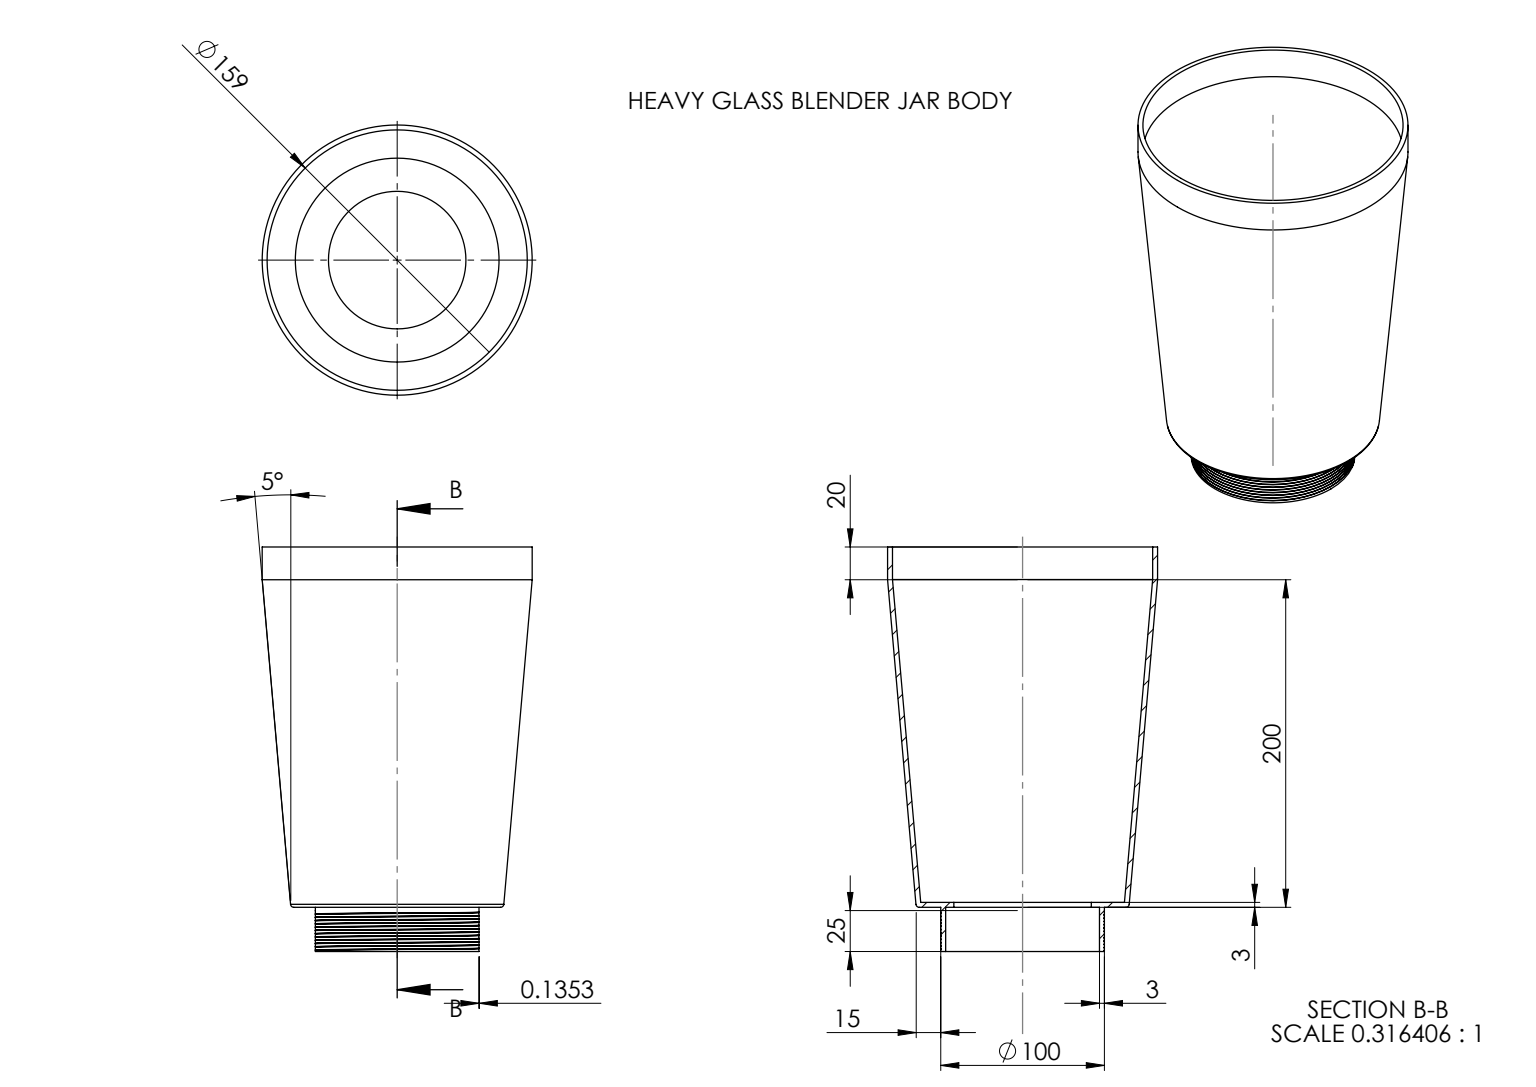
ISO-10303-21;
HEADER;
FILE_DESCRIPTION (('STEP AP214'),
    '1' );
FILE_NAME ('Heavy Glass Blender Jar Body.step',
    '2026-10-09T15:02:13',
    ( '' ),
    ( '' ),
    'SwSTEP 2.0',
    'SolidWorks 2026',
    '' );
FILE_SCHEMA (( 'AUTOMOTIVE_DESIGN' ));
ENDSEC;

DATA;
#4=CARTESIAN_POINT ( 'NONE',  ( -40.34137639590981905, 29.65937500034139518, -29.30972558990011478 ) ) ;
#8=CARTESIAN_POINT ( 'NONE',  ( 47.50025713571348263, 25.00000000000000000, -15.17274647889483496 ) ) ;
#9=CARTESIAN_POINT ( 'NONE',  ( 49.86468353124999453, 35.02187500034139589, -16.20201782572376104 ) ) ;
#10=EDGE_CURVE ( 'NONE', #4476, #13481, #11027, .T. ) ;
#13=LINE ( 'NONE', #15220, #1773 ) ;
#15=DIRECTION ( 'NONE',  ( 0.000000000000000000, 0.9961946980917455452, 0.08715574274765836016 ) ) ;
#18=CARTESIAN_POINT ( 'NONE',  ( 15.40903463028481113, 31.32187500034139305, -47.42413220539094709 ) ) ;
#22=CARTESIAN_POINT ( 'NONE',  ( -30.81806926056962226, 34.15937500034139163, 42.41743335407647209 ) ) ;
#23=ORIENTED_EDGE ( 'NONE', *, *, #4819, .F. ) ;
#26=CARTESIAN_POINT ( 'NONE',  ( -40.45084971874737079, 19.98125000068279888, 29.38926261462367151 ) ) ;
#28=CARTESIAN_POINT ( 'NONE',  ( 15.40903463028481113, 21.32187500034139660, -47.42413220539094709 ) ) ;
#33=CARTESIAN_POINT ( 'NONE',  ( -40.45084971874737789, 45.79999999999999716, -29.38926261462365730 ) ) ;
#41=EDGE_CURVE ( 'NONE', #13641, #5789, #12730, .T. ) ;
#47=( NAMED_UNIT ( * ) SI_UNIT ( $, .STERADIAN. ) SOLID_ANGLE_UNIT ( ) );
#54=CARTESIAN_POINT ( 'NONE',  ( -15.40903463028481646, 25.45937500034139589, -47.42413220539093999 ) ) ;
#56=CARTESIAN_POINT ( 'NONE',  ( -40.45084971874737789, 25.80000000000000071, -29.38926261462365730 ) ) ;
#59=FACE_OUTER_BOUND ( 'NONE', #13989, .T. ) ;
#61=CARTESIAN_POINT ( 'NONE',  ( -1.240322475938754499E-13, 36.28125000068280315, 50.00000000000000000 ) ) ;
#72=CARTESIAN_POINT ( 'NONE',  ( -49.99999999999999289, 23.90000000000000213, -16.24598481164531449 ) ) ;
#76=CARTESIAN_POINT ( 'NONE',  ( 49.86468353124999453, 44.95937500034139589, -16.20201782572376459 ) ) ;
#79=DIRECTION ( 'NONE',  ( -0.000000000000000000, -1.000000000000000000, -0.000000000000000000 ) ) ;
#80=CARTESIAN_POINT ( 'NONE',  ( -49.86468353124999453, 25.95937500034139944, 16.20201782572377525 ) ) ;
#85=CARTESIAN_POINT ( 'NONE',  ( 47.13255506291616115, 25.00000000000000711, -16.27994764699579022 ) ) ;
#86=CARTESIAN_POINT ( 'NONE',  ( -15.40903463028480580, 34.32187500034139305, 47.42413220539094709 ) ) ;
#87=( BOUNDED_CURVE ( )  B_SPLINE_CURVE ( 2, ( #12702, #8875, #13934, #16199, #7548, #15262, #4829, #3730, #6314, #2555, #11379, #10211, #16445 ),
 .UNSPECIFIED., .F., .F. ) 
 B_SPLINE_CURVE_WITH_KNOTS ( ( 3, 2, 2, 2, 2, 2, 3 ),
 ( 0.3166666666666667074, 0.3200000000000000067, 0.3266666666666666607, 0.3333333333333333148, 0.3400000000000000244, 0.3466666666666666785, 0.3500000000000000333 ),
 .UNSPECIFIED. ) 
 CURVE ( )  GEOMETRIC_REPRESENTATION_ITEM ( )  RATIONAL_B_SPLINE_CURVE ( ( 0.9755282581475768211, 0.9755282581475770431, 1.000000000000000000, 0.9510565162951535312, 1.000000000000000000, 0.9510565162951535312, 1.000000000000000000, 0.9510565162951535312, 1.000000000000000000, 0.9510565162951535312, 1.000000000000000000, 0.9755282581475765991, 0.9755282581475768211 ) ) 
 REPRESENTATION_ITEM ( '' )  );
#96=CARTESIAN_POINT ( 'NONE',  ( 30.81806926056964002, 30.62187500034139020, 42.41743335407647209 ) ) ;
#101=CARTESIAN_POINT ( 'NONE',  ( -40.34137639590981905, 35.65937500034139873, -29.30972558990011478 ) ) ;
#104=CARTESIAN_POINT ( 'NONE',  ( -30.81806926056963292, 47.55937500034139731, -42.41743335407647209 ) ) ;
#106=CARTESIAN_POINT ( 'NONE',  ( -49.86468353124999453, 23.82187500034139305, -16.20201782572375393 ) ) ;
#111=CARTESIAN_POINT ( 'NONE',  ( 40.45084971874737789, 44.79999999999999716, 29.38926261462365375 ) ) ;
#120=CARTESIAN_POINT ( 'NONE',  ( -30.90169943749473447, 32.30000000000000426, 42.53254041760200721 ) ) ;
#123=CARTESIAN_POINT ( 'NONE',  ( -49.86468353124999453, 48.02187500034139589, 16.20201782572377169 ) ) ;
#125=EDGE_CURVE ( 'NONE', #10026, #5291, #8135, .T. ) ;
#130=DIRECTION ( 'NONE',  ( 0.000000000000000000, 0.000000000000000000, -1.000000000000000000 ) ) ;
#135=CARTESIAN_POINT ( 'NONE',  ( -15.40903463028481646, 47.52187500034139589, -47.42413220539093999 ) ) ;
#136=ORIENTED_EDGE ( 'NONE', *, *, #8247, .T. ) ;
#138=ORIENTED_EDGE ( 'NONE', *, *, #3634, .T. ) ;
#145=DIRECTION ( 'NONE',  ( 0.000000000000000000, 1.000000000000000000, 0.000000000000000000 ) ) ;
#160=CARTESIAN_POINT ( 'NONE',  ( 15.45084971874737789, 20.60000000000000142, 47.55282581475767500 ) ) ;
#163=CARTESIAN_POINT ( 'NONE',  ( -49.86468353124999453, 37.95937500034140299, 16.20201782572377525 ) ) ;
#171=CARTESIAN_POINT ( 'NONE',  ( -40.34137639590981905, 31.65937500034139873, -29.30972558990011478 ) ) ;
#175=CARTESIAN_POINT ( 'NONE',  ( 46.62157290631164130, 24.99999999999999289, -17.69020581816995730 ) ) ;
#176=CARTESIAN_POINT ( 'NONE',  ( -40.34137639590981195, 32.12187500034140442, 29.30972558990012189 ) ) ;
#177=CARTESIAN_POINT ( 'NONE',  ( 30.90169943749475223, 46.48125000068280599, 42.53254041760199300 ) ) ;
#185=CARTESIAN_POINT ( 'NONE',  ( 9.631387414534489405E-15, 32.42187500034139447, 52.43083105670540789 ) ) ;
#186=ORIENTED_EDGE ( 'NONE', *, *, #13105, .F. ) ;
#187=CARTESIAN_POINT ( 'NONE',  ( 40.34137639590981195, 33.05937500034139731, -29.30972558990011834 ) ) ;
#188=ORIENTED_EDGE ( 'NONE', *, *, #204, .F. ) ;
#191=CARTESIAN_POINT ( 'NONE',  ( -30.90169943749473802, 20.08125000068279320, 42.53254041760200721 ) ) ;
#194=CARTESIAN_POINT ( 'NONE',  ( 30.81806926056964002, 26.62187500034139731, 42.41743335407647209 ) ) ;
#200=CARTESIAN_POINT ( 'NONE',  ( 30.90169943749474157, 49.29999999999999716, -42.53254041760200721 ) ) ;
#204=EDGE_CURVE ( 'NONE', #5010, #3842, #426, .T. ) ;
#206=EDGE_LOOP ( 'NONE', ( #10234, #136 ) ) ;
#207=CARTESIAN_POINT ( 'NONE',  ( 50.00000000000000000, 36.78125000068280315, -6.123233995736766085E-15 ) ) ;
#208=AXIS2_PLACEMENT_3D ( 'NONE', #5247, #15355, #10131 ) ;
#209=ORIENTED_EDGE ( 'NONE', *, *, #12461, .T. ) ;
#215=CARTESIAN_POINT ( 'NONE',  ( 49.86468353124999453, 45.02187500034138878, -16.20201782572376104 ) ) ;
#221=CARTESIAN_POINT ( 'NONE',  ( 50.00000000000000000, 34.78125000068280315, -6.123233995736766085E-15 ) ) ;
#225=CARTESIAN_POINT ( 'NONE',  ( -49.86468353125000164, 45.92187500034139447, 0.000000000000000000 ) ) ;
#241=CARTESIAN_POINT ( 'NONE',  ( -50.00000000000000000, 20.00000000000000000, 0.000000000000000000 ) ) ;
#244=CARTESIAN_POINT ( 'NONE',  ( -3.210462471511496205E-15, 39.35937500034138736, -52.43083105670540789 ) ) ;
#247=CARTESIAN_POINT ( 'NONE',  ( 49.99999999999999289, 48.88125000068279746, -16.24598481164532160 ) ) ;
#249=CARTESIAN_POINT ( 'NONE',  ( -49.86468353124999453, 31.75937500034140015, -16.20201782572375393 ) ) ;
#252=CARTESIAN_POINT ( 'NONE',  ( 50.00000000000000711, 26.89999999999999858, 16.24598481164530739 ) ) ;
#255=CARTESIAN_POINT ( 'NONE',  ( 30.81806926056962936, 35.22187500034138452, -42.41743335407646498 ) ) ;
#263=CARTESIAN_POINT ( 'NONE',  ( -15.40903463028481646, 27.52187500034139944, -47.42413220539093999 ) ) ;
#266=B_SPLINE_CURVE_WITH_KNOTS ( 'NONE', 3,
 ( #13888, #7584, #1338, #3766, #3845, #12662, #9000, #3929, #8825, #2503, #1169, #9081, #15216, #1258, #12497, #11416, #1090, #15389, #12572, #6350, #6265, #8, #6428, #1418, #6182, #14058, #2674, #11488, #85, #7748, #12816, #6510, #3692, #15064, #11567, #5111, #10245, #175, #10166, #5280, #11336, #10331, #4011, #2348, #16313, #7429, #11256, #8911, #4949, #10007, #8747, #13812, #2423, #7501, #16403, #10088, #13975, #5036, #2594, #15138, #7670 ),
 .UNSPECIFIED., .F., .F.,
 ( 4, 3, 3, 3, 3, 3, 3, 3, 3, 3, 3, 3, 3, 3, 3, 3, 3, 3, 3, 3, 4 ),
 ( 5.250942343321584884E-16, 0.0001250000981872776470, 0.0006250122739946113812, 0.001125024449802053753, 0.001625036625609322868, 0.002125048801416675251, 0.002625060977223842018, 0.003125073153031292413, 0.003625085328838458312, 0.004125097504645739571, 0.004625109680452853429, 0.005125121856260251782, 0.005625134032067363038, 0.006125146207874809963, 0.006625158383682325410, 0.007125170559489371613, 0.007625182735296599096, 0.008125194911103644432, 0.008625207086911109572, 0.009137502482430032158, 0.009649851960371033655 ),
 .UNSPECIFIED. ) ;
#267=CARTESIAN_POINT ( 'NONE',  ( 15.40903463028481113, 39.25937500034140015, -47.42413220539094709 ) ) ;
#268=ORIENTED_EDGE ( 'NONE', *, *, #1513, .T. ) ;
#271=CARTESIAN_POINT ( 'NONE',  ( -49.86468353124999453, 47.75937500034139305, -16.20201782572375393 ) ) ;
#272=CARTESIAN_POINT ( 'NONE',  ( -49.86468353125000164, 49.85937500034139447, 0.000000000000000000 ) ) ;
#273=CARTESIAN_POINT ( 'NONE',  ( -15.40903463028480580, 20.32187500034139660, 47.42413220539094709 ) ) ;
#278=CARTESIAN_POINT ( 'NONE',  ( -15.45084971874736368, 40.40000000000000568, 47.55282581475768211 ) ) ;
#287=CARTESIAN_POINT ( 'NONE',  ( 30.90169943749475578, 34.48125000068279888, 42.53254041760200010 ) ) ;
#291=DIRECTION ( 'NONE',  ( 0.000000000000000000, 0.000000000000000000, 1.000000000000000000 ) ) ;
#292=CARTESIAN_POINT ( 'NONE',  ( 49.86468353125000164, 48.92187500034139447, -6.106662507704105588E-15 ) ) ;
#299=CARTESIAN_POINT ( 'NONE',  ( 40.45084971874737079, 34.98125000068279888, -29.38926261462366440 ) ) ;
#303=CARTESIAN_POINT ( 'NONE',  ( 9.631387414534489405E-15, 48.42187500034140157, 52.43083105670540789 ) ) ;
#304=ORIENTED_EDGE ( 'NONE', *, *, #3039, .T. ) ;
#305=VERTEX_POINT ( 'NONE', #3593 ) ;
#319=CARTESIAN_POINT ( 'NONE',  ( 1.293669679204937499E-13, 37.28125000068280315, -50.00000000000000000 ) ) ;
#320=EDGE_CURVE ( 'NONE', #5080, #1275, #14407, .T. ) ;
#324=CARTESIAN_POINT ( 'NONE',  ( -49.86468353125000164, 39.85937500034139447, 0.000000000000000000 ) ) ;
#326=VERTEX_POINT ( 'NONE', #10076 ) ;
#327=CARTESIAN_POINT ( 'NONE',  ( -50.00000000000000000, 47.78125000068279604, 0.000000000000000000 ) ) ;
#330=CARTESIAN_POINT ( 'NONE',  ( -15.40903463028480580, 20.25937500034139660, 47.42413220539094709 ) ) ;
#336=CARTESIAN_POINT ( 'NONE',  ( 40.34137639590981195, 27.12187500034139731, -29.30972558990011834 ) ) ;
#343=CARTESIAN_POINT ( 'NONE',  ( 15.45084971874736723, 35.39999999999999858, -47.55282581475768211 ) ) ;
#348=CARTESIAN_POINT ( 'NONE',  ( 49.86468353124999453, 26.95937500034139944, -16.20201782572376104 ) ) ;
#351=CARTESIAN_POINT ( 'NONE',  ( -49.86468353124999453, 39.95937500034139589, 16.20201782572377525 ) ) ;
#358=CARTESIAN_POINT ( 'NONE',  ( -49.99999999999999289, 44.09999999999999432, 16.24598481164533226 ) ) ;
#360=CARTESIAN_POINT ( 'NONE',  ( -49.86468353124999453, 43.82187500034140015, -16.20201782572375393 ) ) ;
#363=CARTESIAN_POINT ( 'NONE',  ( -15.40903463028480580, 48.25937500034140015, 47.42413220539094709 ) ) ;
#365=CARTESIAN_POINT ( 'NONE',  ( 9.657523855033129090E-15, 36.28125000068278894, 52.57311121191334990 ) ) ;
#370=CARTESIAN_POINT ( 'NONE',  ( 9.631387414534489405E-15, 44.42187500034140157, 52.43083105670540789 ) ) ;
#376=CARTESIAN_POINT ( 'NONE',  ( 0.000000000000000000, 54.99999999999999289, 0.000000000000000000 ) ) ;
#380=CARTESIAN_POINT ( 'NONE',  ( -49.86468353124999453, 49.82187500034140015, -16.20201782572375393 ) ) ;
#389=DIRECTION ( 'NONE',  ( 0.000000000000000000, 0.000000000000000000, 1.000000000000000000 ) ) ;
#393=CARTESIAN_POINT ( 'NONE',  ( 0.000000000000000000, 193.4213562373095385, -50.00000000000000000 ) ) ;
#394=CARTESIAN_POINT ( 'NONE',  ( -50.00000000000000000, 33.78125000068280315, 0.000000000000000000 ) ) ;
#397=CARTESIAN_POINT ( 'NONE',  ( -1.240322475938754499E-13, 38.28125000068280315, 50.00000000000000000 ) ) ;
#402=EDGE_LOOP ( 'NONE', ( #5956, #13937, #15950, #9796 ) ) ;
#403=CARTESIAN_POINT ( 'NONE',  ( -49.86468353124999453, 39.95937500034139589, 16.20201782572377525 ) ) ;
#412=CARTESIAN_POINT ( 'NONE',  ( -15.40903463028480580, 22.25937500034139660, 47.42413220539094709 ) ) ;
#417=CARTESIAN_POINT ( 'NONE',  ( 30.90169943749473802, 35.29999999999999716, -42.53254041760200721 ) ) ;
#418=CARTESIAN_POINT ( 'NONE',  ( -40.34137639590981195, 42.05937500034139731, 29.30972558990012189 ) ) ;
#419=DIRECTION ( 'NONE',  ( 1.224646799147349509E-16, 0.000000000000000000, -1.000000000000000000 ) ) ;
#420=CARTESIAN_POINT ( 'NONE',  ( -3.210462471511496205E-15, 27.42187500034139092, -52.43083105670540789 ) ) ;
#421=CARTESIAN_POINT ( 'NONE',  ( -5.823736356558309156E-14, 44.50000000000000000, 50.00000000000000000 ) ) ;
#426=CIRCLE ( 'NONE', #15019, 62.25100647794772613 ) ;
#427=CARTESIAN_POINT ( 'NONE',  ( 40.45084971874737789, 34.80000000000000426, 29.38926261462365375 ) ) ;
#435=CARTESIAN_POINT ( 'NONE',  ( -15.40903463028481646, 29.45937500034139589, -47.42413220539093999 ) ) ;
#436=VERTEX_POINT ( 'NONE', #8430 ) ;
#438=CARTESIAN_POINT ( 'NONE',  ( 15.40903463028482356, 42.45937500034140299, 47.42413220539093999 ) ) ;
#439=CARTESIAN_POINT ( 'NONE',  ( -3.111920190527341144E-15, 27.50000000000000000, -50.00000000000000000 ) ) ;
#440=CARTESIAN_POINT ( 'NONE',  ( 9.631387414534489405E-15, 20.42187500034139802, 52.43083105670540789 ) ) ;
#447=CARTESIAN_POINT ( 'NONE',  ( -30.90169943749473802, 44.30000000000001137, 42.53254041760200721 ) ) ;
#449=CARTESIAN_POINT ( 'NONE',  ( 15.40903463028482356, 42.52187500034139589, 47.42413220539093999 ) ) ;
#453=ORIENTED_EDGE ( 'NONE', *, *, #626, .F. ) ;
#454=CARTESIAN_POINT ( 'NONE',  ( 50.00000000000000000, 30.78125000068279959, -6.123233995736766085E-15 ) ) ;
#459=CARTESIAN_POINT ( 'NONE',  ( 30.81806926056964002, 46.62187500034139731, 42.41743335407646498 ) ) ;
#468=CARTESIAN_POINT ( 'NONE',  ( -40.34137639590981905, 49.72187500034139873, -29.30972558990011478 ) ) ;
#480=AXIS2_PLACEMENT_3D ( 'NONE', #4431, #4348, #13149 ) ;
#486=CARTESIAN_POINT ( 'NONE',  ( 8.446640517145639571E-15, 26.28125000068279959, 50.00000000000000000 ) ) ;
#488=CARTESIAN_POINT ( 'NONE',  ( 15.40903463028481113, 37.25937500034140015, -47.42413220539094709 ) ) ;
#490=ORIENTED_EDGE ( 'NONE', *, *, #10727, .F. ) ;
#491=CARTESIAN_POINT ( 'NONE',  ( -15.45084971874736368, 48.18125000068280173, 47.55282581475768211 ) ) ;
#494=CARTESIAN_POINT ( 'NONE',  ( -49.86468353124999453, 23.75937500034140015, -16.20201782572375393 ) ) ;
#495=VERTEX_POINT ( 'NONE', #2020 ) ;
#497=CARTESIAN_POINT ( 'NONE',  ( -30.90169943749474513, 47.70000000000000284, -42.53254041760200721 ) ) ;
#500=CARTESIAN_POINT ( 'NONE',  ( -3.210462471511496205E-15, 25.42187500034139447, -52.43083105670540789 ) ) ;
#508=CIRCLE ( 'NONE', #13785, 50.00000000000000000 ) ;
#509=CARTESIAN_POINT ( 'NONE',  ( 15.45084971874737789, 32.60000000000000142, 47.55282581475767500 ) ) ;
#511=CARTESIAN_POINT ( 'NONE',  ( 1.293669679204937499E-13, 41.28125000068279604, -50.00000000000000000 ) ) ;
#514=CARTESIAN_POINT ( 'NONE',  ( 40.34137639590981195, 27.05937500034139731, -29.30972558990011834 ) ) ;
#517=CARTESIAN_POINT ( 'NONE',  ( 49.86468353125000164, 40.85937500034139447, -6.106662507704105588E-15 ) ) ;
#525=CARTESIAN_POINT ( 'NONE',  ( -40.45084971874737079, 40.20000000000000284, 29.38926261462367151 ) ) ;
#527=CARTESIAN_POINT ( 'NONE',  ( 15.40903463028481113, 47.32187500034140015, -47.42413220539094709 ) ) ;
#531=CARTESIAN_POINT ( 'NONE',  ( 15.40903463028481113, 47.25937500034140015, -47.42413220539094709 ) ) ;
#533=CARTESIAN_POINT ( 'NONE',  ( 50.00000000000000000, 32.78125000068279604, -6.123233995736766085E-15 ) ) ;
#534=EDGE_CURVE ( 'NONE', #9508, #1121, #9961, .T. ) ;
#538=CARTESIAN_POINT ( 'NONE',  ( 40.34137639590981195, 43.12187500034139731, -29.30972558990011834 ) ) ;
#540=FACE_OUTER_BOUND ( 'NONE', #4983, .T. ) ;
#546=CARTESIAN_POINT ( 'NONE',  ( -30.81806926056963292, 41.62187500034139020, -42.41743335407647209 ) ) ;
#559=LINE ( 'NONE', #811, #4989 ) ;
#561=CARTESIAN_POINT ( 'NONE',  ( 40.45084971874737789, 36.79999999999999716, 29.38926261462365375 ) ) ;
#563=CARTESIAN_POINT ( 'NONE',  ( -49.86468353124999453, 31.75937500034140015, -16.20201782572375393 ) ) ;
#565=ORIENTED_EDGE ( 'NONE', *, *, #14515, .F. ) ;
#570=CARTESIAN_POINT ( 'NONE',  ( 40.34137639590981905, 22.65937500034139518, 29.30972558990010768 ) ) ;
#575=CARTESIAN_POINT ( 'NONE',  ( 15.40903463028482356, 30.52187500034139589, 47.42413220539093999 ) ) ;
#576=DIRECTION ( 'NONE',  ( -0.000000000000000000, -1.000000000000000000, -0.000000000000000000 ) ) ;
#582=CARTESIAN_POINT ( 'NONE',  ( -49.99999999999999289, 35.90000000000000568, -16.24598481164531449 ) ) ;
#584=CARTESIAN_POINT ( 'NONE',  ( -40.34137639590981905, 47.65937500034139873, -29.30972558990011478 ) ) ;
#587=UNCERTAINTY_MEASURE_WITH_UNIT (LENGTH_MEASURE( 1.000000000000000082E-05 ), #11527, 'distance_accuracy_value', 'NONE');
#588=CARTESIAN_POINT ( 'NONE',  ( 15.40903463028482356, 28.45937500034139589, 47.42413220539093999 ) ) ;
#592=CARTESIAN_POINT ( 'NONE',  ( 30.81806926056962936, 41.15937500034139873, -42.41743335407647209 ) ) ;
#598=CARTESIAN_POINT ( 'NONE',  ( 30.81806926056962936, 31.22187500034139873, -42.41743335407647209 ) ) ;
#599=CARTESIAN_POINT ( 'NONE',  ( 30.90169943749474157, 39.30000000000000426, -42.53254041760200721 ) ) ;
#602=CARTESIAN_POINT ( 'NONE',  ( -49.86468353124999453, 46.02187500034140299, 16.20201782572377525 ) ) ;
#609=CARTESIAN_POINT ( 'NONE',  ( -40.45084971874737079, 29.98125000068279888, 29.38926261462367151 ) ) ;
#614=CARTESIAN_POINT ( 'NONE',  ( -30.81806926056963292, 39.62187500034139020, -42.41743335407646498 ) ) ;
#623=CARTESIAN_POINT ( 'NONE',  ( 15.40903463028482356, 40.52187500034139589, 47.42413220539093999 ) ) ;
#625=ORIENTED_EDGE ( 'NONE', *, *, #15445, .T. ) ;
#626=EDGE_CURVE ( 'NONE', #4982, #15172, #5286, .T. ) ;
#631=DIRECTION ( 'NONE',  ( -0.000000000000000000, -1.000000000000000000, -0.000000000000000000 ) ) ;
#636=CARTESIAN_POINT ( 'NONE',  ( -30.90169943749474513, 45.70000000000000284, -42.53254041760200721 ) ) ;
#643=CARTESIAN_POINT ( 'NONE',  ( -40.34137639590981905, 31.65937500034139873, -29.30972558990011478 ) ) ;
#647=CARTESIAN_POINT ( 'NONE',  ( -15.45084971874736368, 46.18125000068280173, 47.55282581475768211 ) ) ;
#649=CARTESIAN_POINT ( 'NONE',  ( -49.86468353125000164, 21.85937500034139802, 0.000000000000000000 ) ) ;
#651=CARTESIAN_POINT ( 'NONE',  ( -1.240322475938754499E-13, 38.50000000000000711, 50.00000000000000000 ) ) ;
#655=CARTESIAN_POINT ( 'NONE',  ( 9.631387414534489405E-15, 28.42187500034139447, 52.43083105670540789 ) ) ;
#657=EDGE_CURVE ( 'NONE', #9775, #5127, #7632, .T. ) ;
#665=CARTESIAN_POINT ( 'NONE',  ( -40.45084971874737789, 31.80000000000000071, -29.38926261462365730 ) ) ;
#669=CARTESIAN_POINT ( 'NONE',  ( -15.40903463028480580, 28.25937500034139660, 47.42413220539094709 ) ) ;
#670=ORIENTED_EDGE ( 'NONE', *, *, #3372, .F. ) ;
#673=CARTESIAN_POINT ( 'NONE',  ( 30.81806926056962936, 39.15937500034139873, -42.41743335407647209 ) ) ;
#681=AXIS2_PLACEMENT_3D ( 'NONE', #11414, #6347, #2840 ) ;
#683=CARTESIAN_POINT ( 'NONE',  ( -40.34137639590981905, 27.72187500034139873, -29.30972558990011478 ) ) ;
#684=CIRCLE ( 'NONE', #9999, 82.49773270518484480 ) ;
#685=CIRCLE ( 'NONE', #1492, 47.00000000000000000 ) ;
#688=CARTESIAN_POINT ( 'NONE',  ( -3.210462471511496205E-15, 43.42187500034140157, -52.43083105670540789 ) ) ;
#692=CARTESIAN_POINT ( 'NONE',  ( 30.81806926056964002, 48.55937500034139020, 42.41743335407646498 ) ) ;
#699=CARTESIAN_POINT ( 'NONE',  ( -30.90169943749473802, 28.08125000068280031, 42.53254041760200721 ) ) ;
#701=EDGE_CURVE ( 'NONE', #14905, #2524, #8950, .T. ) ;
#703=CARTESIAN_POINT ( 'NONE',  ( -3.210462471511496205E-15, 43.42187500034140157, -52.43083105670540789 ) ) ;
#710=CIRCLE ( 'NONE', #11875, 50.00000000000000000 ) ;
#715=CARTESIAN_POINT ( 'NONE',  ( -15.40903463028480580, 40.32187500034140015, 47.42413220539094709 ) ) ;
#722=( BOUNDED_CURVE ( )  B_SPLINE_CURVE ( 2, ( #13103, #13189, #11525, #15348, #2961, #2709, #1463, #9040, #11857, #15677, #292, #15427, #1708, #11770, #7789, #4222, #14094, #6468, #8029, #123, #9117, #2884, #6721, #9367, #14176, #2794, #7869, #3965, #6805, #1551, #4303, #9207, #14263, #459, #12858, #10368, #6644, #5391, #5238, #10294, #10542, #10450, #15506, #4132, #6557, #11617, #8109, #7953, #9289, #215, #13025, #1627, #14345, #5562, #5318, #370, #5473, #14417, #3037, #15601, #2112, #7125, #12096, #14741, #12015, #703, #11937, #2034, #538, #5791, #782, #4627, #6885, #9689, #9535, #5874, #1793, #3204, #863, #12262, #1866, #14829, #5632, #10936, #12183, #10696, #16000, #3376, #10858, #8441, #15924, #3286, #15752, #4546, #13505, #4380, #3458, #11020, #7039, #15844, #9609, #7199, #6962, #614, #13343, #14658, #8355, #5958, #16088, #5710, #13424, #9445, #4723, #14499, #9784, #8519, #3128, #8200, #1946, #13266, #10778, #4468, #14579, #8277, #14059, #1260, #1419, #4091, #10167, #945, #4012, #13584, #11489, #13889, #2753, #7671, #2191, #12663, #6351, #4806, #11417, #6429, #13976, #12904, #10246, #6044, #14138, #255, #5360, #9, #7829, #11115, #15217, #15307, #5112, #9082, #86, #1512, #10089, #5191, #12741, #10414, #16176, #6604, #6511, #11657, #7288, #15470, #2595, #12344, #7585, #15139, #3846, #3767, #8826, #3930, #9001, #2504, #176, #8912, #1339, #2675, #7749, #12817, #11568, #5281, #10332, #15390, #13306, #14305, #8072, #4344, #15641, #7000, #575, #11814, #4428, #10585, #1830, #5599, #11979, #1906, #2844, #11901, #10825, #8163, #6769, #6925, #12988, #1671, #3171, #9252, #11734, #9161, #4185, #655, #15797, #1592, #10737, #6686, #12055, #8240, #9497, #13145, #4264, #420, #5522, #5670, #336, #9331, #5756, #2927, #5435, #14218, #7994, #15888, #14543, #10497, #7911, #15555, #13068, #14382, #3003, #1754, #6853, #500, #9409, #10661, #15714, #14455, #3086 ),
 .UNSPECIFIED., .F., .T. ) 
 B_SPLINE_CURVE_WITH_KNOTS ( ( 3, 2, 2, 2, 2, 2, 2, 2, 2, 2, 2, 2, 2, 2, 2, 2, 2, 2, 2, 2, 2, 2, 2, 2, 2, 2, 2, 2, 2, 2, 2, 2, 2, 2, 2, 2, 2, 2, 2, 2, 2, 2, 2, 2, 2, 2, 2, 2, 2, 2, 2, 2, 2, 2, 2, 2, 2, 2, 2, 2, 2, 2, 2, 2, 2, 2, 2, 2, 2, 2, 2, 2, 2, 2, 2, 2, 2, 2, 2, 2, 2, 2, 2, 2, 2, 2, 2, 2, 2, 2, 2, 2, 2, 2, 2, 2, 2, 2, 2, 2, 2, 2, 2, 2, 2, 2, 2, 2, 2, 2, 2, 2, 2, 2, 2, 2, 2, 2, 2, 2, 2, 2, 2, 2, 2, 3 ),
 ( 0.000000000000000000, 0.006666666666666667095, 0.01333333333333333419, 0.02000000000000000042, 0.02666666666666666838, 0.03333333333333333287, 0.04000000000000000083, 0.04666666666666666879, 0.05333333333333333676, 0.05999999999999999778, 0.06666666666666666574, 0.07333333333333333370, 0.08000000000000000167, 0.08666666666666666963, 0.09333333333333333759, 0.1000000000000000194, 0.1066666666666666735, 0.1133333333333333276, 0.1199999999999999956, 0.1266666666666666774, 0.1333333333333333315, 0.1400000000000000133, 0.1466666666666666674, 0.1533333333333333215, 0.1600000000000000033, 0.1666666666666666574, 0.1733333333333333393, 0.1799999999999999933, 0.1866666666666666752, 0.1933333333333333570, 0.2000000000000000389, 0.2066666666666666652, 0.2133333333333333470, 0.2200000000000000011, 0.2266666666666666552, 0.2333333333333333370, 0.2399999999999999911, 0.2466666666666666730, 0.2533333333333333548, 0.2600000000000000089, 0.2666666666666666630, 0.2733333333333333171, 0.2800000000000000266, 0.2866666666666666807, 0.2933333333333333348, 0.2999999999999999889, 0.3066666666666666430, 0.3133333333333333526, 0.3200000000000000067, 0.3266666666666666052, 0.3333333333333333148, 0.3399999999999999689, 0.3466666666666666785, 0.3533333333333333326, 0.3599999999999999867, 0.3666666666666666408, 0.3733333333333333504, 0.3800000000000000044, 0.3866666666666667140, 0.3933333333333333126, 0.4000000000000000777, 0.4066666666666666763, 0.4133333333333333304, 0.4199999999999999845, 0.4266666666666666941, 0.4333333333333333481, 0.4400000000000000022, 0.4466666666666667118, 0.4533333333333333104, 0.4600000000000000755, 0.4666666666666666741, 0.4733333333333333282, 0.4799999999999999822, 0.4866666666666666918, 0.4933333333333333459, 0.5000000000000000000, 0.5066666666666667096, 0.5133333333333333082, 0.5200000000000000178, 0.5266666666666666163, 0.5333333333333333259, 0.5400000000000000355, 0.5466666666666666341, 0.5533333333333333437, 0.5600000000000000533, 0.5666666666666666519, 0.5733333333333333615, 0.5799999999999999600, 0.5866666666666666696, 0.5933333333333333792, 0.5999999999999999778, 0.6066666666666665764, 0.6133333333333332860, 0.6199999999999999956, 0.6266666666666667052, 0.6333333333333333037, 0.6400000000000000133, 0.6466666666666666119, 0.6533333333333332105, 0.6600000000000000311, 0.6666666666666666297, 0.6733333333333333393, 0.6799999999999999378, 0.6866666666666666474, 0.6933333333333333570, 0.6999999999999998446, 0.7066666666666666652, 0.7133333333333333748, 0.7199999999999999734, 0.7266666666666665719, 0.7333333333333332815, 0.7399999999999999911, 0.7466666666666667007, 0.7533333333333332993, 0.7600000000000000089, 0.7666666666666667185, 0.7733333333333334281, 0.7800000000000000266, 0.7866666666666666252, 0.7933333333333333348, 0.8000000000000001554, 0.8066666666666666430, 0.8133333333333333526, 0.8200000000000000622, 0.8266666666666666607, 0.8307121371438114243 ),
 .UNSPECIFIED. ) 
 CURVE ( )  GEOMETRIC_REPRESENTATION_ITEM ( )  RATIONAL_B_SPLINE_CURVE ( ( 1.000000000000000000, 0.9510565162951535312, 1.000000000000000000, 0.9510565162951535312, 1.000000000000000000, 0.9510565162951535312, 1.000000000000000000, 0.9510565162951535312, 1.000000000000000000, 0.9510565162951535312, 1.000000000000000000, 0.9510565162951535312, 1.000000000000000000, 0.9510565162951535312, 1.000000000000000000, 0.9510565162951535312, 1.000000000000000000, 0.9510565162951535312, 1.000000000000000000, 0.9510565162951535312, 1.000000000000000000, 0.9510565162951535312, 1.000000000000000000, 0.9510565162951535312, 1.000000000000000000, 0.9510565162951535312, 1.000000000000000000, 0.9510565162951535312, 1.000000000000000000, 0.9510565162951535312, 1.000000000000000000, 0.9510565162951535312, 1.000000000000000000, 0.9510565162951535312, 1.000000000000000000, 0.9510565162951535312, 1.000000000000000000, 0.9510565162951535312, 1.000000000000000000, 0.9510565162951535312, 1.000000000000000000, 0.9510565162951535312, 1.000000000000000000, 0.9510565162951535312, 1.000000000000000000, 0.9510565162951535312, 1.000000000000000000, 0.9510565162951535312, 1.000000000000000000, 0.9510565162951535312, 1.000000000000000000, 0.9510565162951535312, 1.000000000000000000, 0.9510565162951535312, 1.000000000000000000, 0.9510565162951535312, 1.000000000000000000, 0.9510565162951535312, 1.000000000000000000, 0.9510565162951535312, 1.000000000000000000, 0.9510565162951535312, 1.000000000000000000, 0.9510565162951535312, 1.000000000000000000, 0.9510565162951535312, 1.000000000000000000, 0.9510565162951535312, 1.000000000000000000, 0.9510565162951535312, 1.000000000000000000, 0.9510565162951535312, 1.000000000000000000, 0.9510565162951535312, 1.000000000000000000, 0.9510565162951535312, 1.000000000000000000, 0.9510565162951535312, 1.000000000000000000, 0.9510565162951535312, 1.000000000000000000, 0.9510565162951535312, 1.000000000000000000, 0.9510565162951535312, 1.000000000000000000, 0.9510565162951535312, 1.000000000000000000, 0.9510565162951535312, 1.000000000000000000, 0.9510565162951535312, 1.000000000000000000, 0.9510565162951535312, 1.000000000000000000, 0.9510565162951535312, 1.000000000000000000, 0.9510565162951535312, 1.000000000000000000, 0.9510565162951535312, 1.000000000000000000, 0.9510565162951535312, 1.000000000000000000, 0.9510565162951535312, 1.000000000000000000, 0.9510565162951535312, 1.000000000000000000, 0.9510565162951535312, 1.000000000000000000, 0.9510565162951535312, 1.000000000000000000, 0.9510565162951535312, 1.000000000000000000, 0.9510565162951535312, 1.000000000000000000, 0.9510565162951535312, 1.000000000000000000, 0.9510565162951535312, 1.000000000000000000, 0.9510565162951535312, 1.000000000000000000, 0.9510565162951535312, 1.000000000000000000, 0.9510565162951535312, 1.000000000000000000, 0.9510565162951535312, 1.000000000000000000, 0.9510565162951535312, 1.000000000000000000, 0.9510565162951535312, 1.000000000000000000, 0.9510565162951535312, 1.000000000000000000, 0.9510565162951535312, 1.000000000000000000, 0.9510565162951535312, 1.000000000000000000, 0.9510565162951535312, 1.000000000000000000, 0.9510565162951535312, 1.000000000000000000, 0.9510565162951535312, 1.000000000000000000, 0.9510565162951535312, 1.000000000000000000, 0.9510565162951535312, 1.000000000000000000, 0.9510565162951535312, 1.000000000000000000, 0.9510565162951535312, 1.000000000000000000, 0.9510565162951535312, 1.000000000000000000, 0.9510565162951535312, 1.000000000000000000, 0.9510565162951535312, 1.000000000000000000, 0.9510565162951535312, 1.000000000000000000, 0.9510565162951535312, 1.000000000000000000, 0.9510565162951535312, 1.000000000000000000, 0.9510565162951535312, 1.000000000000000000, 0.9510565162951535312, 1.000000000000000000, 0.9510565162951535312, 1.000000000000000000, 0.9510565162951535312, 1.000000000000000000, 0.9510565162951535312, 1.000000000000000000, 0.9510565162951535312, 1.000000000000000000, 0.9510565162951535312, 1.000000000000000000, 0.9510565162951535312, 1.000000000000000000, 0.9510565162951535312, 1.000000000000000000, 0.9510565162951535312, 1.000000000000000000, 0.9510565162951535312, 1.000000000000000000, 0.9510565162951535312, 1.000000000000000000, 0.9510565162951535312, 1.000000000000000000, 0.9510565162951535312, 1.000000000000000000, 0.9510565162951535312, 1.000000000000000000, 0.9510565162951535312, 1.000000000000000000, 0.9510565162951535312, 1.000000000000000000, 0.9510565162951535312, 1.000000000000000000, 0.9510565162951535312, 1.000000000000000000, 0.9510565162951535312, 1.000000000000000000, 0.9510565162951535312, 1.000000000000000000, 0.9510565162951535312, 1.000000000000000000, 0.9510565162951535312, 1.000000000000000000, 0.9510565162951535312, 1.000000000000000000, 0.9510565162951535312, 1.000000000000000000, 0.9510565162951535312, 1.000000000000000000, 0.9510565162951535312, 1.000000000000000000, 0.9510565162951535312, 1.000000000000000000, 0.9510565162951535312, 1.000000000000000000, 0.9510565162951535312, 1.000000000000000000, 0.9510565162951535312, 1.000000000000000000, 0.9510565162951535312, 1.000000000000000000, 0.9510565162951535312, 1.000000000000000000, 0.9510565162951535312, 1.000000000000000000, 0.9510565162951535312, 1.000000000000000000, 0.9510565162951535312, 1.000000000000000000, 0.9510565162951535312, 1.000000000000000000, 0.9510565162951535312, 1.000000000000000000, 0.9510565162951535312, 1.000000000000000000, 0.9510565162951535312, 1.000000000000000000, 0.9510565162951535312, 1.000000000000000000, 0.9510565162951535312, 1.000000000000000000, 0.9510565162951535312, 1.000000000000000000, 0.9510565162951535312, 1.000000000000000000, 0.9703000872435151303, 0.9766452105560694541 ) ) 
 REPRESENTATION_ITEM ( '' )  );
#723=ADVANCED_FACE ( 'NONE', ( #12824 ), #12909, .T. ) ;
#736=EDGE_LOOP ( 'NONE', ( #3284, #6956, #2417, #3297 ) ) ;
#737=CARTESIAN_POINT ( 'NONE',  ( -30.81806926056962226, 28.15937500034139518, 42.41743335407647919 ) ) ;
#741=CARTESIAN_POINT ( 'NONE',  ( -40.45084971874737079, 43.98125000068279888, 29.38926261462367151 ) ) ;
#746=CARTESIAN_POINT ( 'NONE',  ( -30.90169943749473447, 38.29999999999999716, 42.53254041760200721 ) ) ;
#748=DIRECTION ( 'NONE',  ( 0.000000000000000000, -1.000000000000000000, 0.000000000000000000 ) ) ;
#754=CARTESIAN_POINT ( 'NONE',  ( 9.657523855033129090E-15, 28.49999999999999645, 52.57311121191334990 ) ) ;
#756=CARTESIAN_POINT ( 'NONE',  ( 30.81806926056962936, 49.15937500034138452, -42.41743335407647209 ) ) ;
#763=CARTESIAN_POINT ( 'NONE',  ( -49.86468353124999453, 35.95937500034139589, 16.20201782572377525 ) ) ;
#765=CARTESIAN_POINT ( 'NONE',  ( -3.111920190527341144E-15, 45.28125000068279604, -50.00000000000000000 ) ) ;
#770=CARTESIAN_POINT ( 'NONE',  ( -30.81806926056963292, 29.62187500034139376, -42.41743335407647209 ) ) ;
#771=CARTESIAN_POINT ( 'NONE',  ( 49.99999999999999289, 33.10000000000000142, -16.24598481164532160 ) ) ;
#773=CARTESIAN_POINT ( 'NONE',  ( 30.81806926056962936, 35.22187500034138452, -42.41743335407647209 ) ) ;
#775=ORIENTED_EDGE ( 'NONE', *, *, #10887, .F. ) ;
#777=CARTESIAN_POINT ( 'NONE',  ( -49.86468353124999453, 41.95937500034139589, 16.20201782572377169 ) ) ;
#779=CARTESIAN_POINT ( 'NONE',  ( -49.99999999999999289, 33.68125000068278752, -16.24598481164531449 ) ) ;
#782=CARTESIAN_POINT ( 'NONE',  ( 49.86468353125000164, 42.92187500034140157, -6.106662507704105588E-15 ) ) ;
#786=CARTESIAN_POINT ( 'NONE',  ( -15.40903463028480580, 22.32187500034139660, 47.42413220539094709 ) ) ;
#795=CARTESIAN_POINT ( 'NONE',  ( 30.81806926056962936, 43.22187500034140584, -42.41743335407647209 ) ) ;
#801=CARTESIAN_POINT ( 'NONE',  ( 7.960204194457797252E-15, 52.00000000000000711, -65.00000000000000000 ) ) ;
#807=CARTESIAN_POINT ( 'NONE',  ( 30.90169943749473802, 25.30000000000000071, -42.53254041760200721 ) ) ;
#808=CARTESIAN_POINT ( 'NONE',  ( 6.123233995736766085E-15, 193.4213562373095385, 50.00000000000000000 ) ) ;
#809=( NAMED_UNIT ( * ) PLANE_ANGLE_UNIT ( ) SI_UNIT ( $, .RADIAN. ) );
#811=CARTESIAN_POINT ( 'NONE',  ( 0.000000000000000000, 193.4213562373095385, -50.00000000000000000 ) ) ;
#812=CARTESIAN_POINT ( 'NONE',  ( 30.90169943749475223, 42.48125000068279888, 42.53254041760199300 ) ) ;
#816=CARTESIAN_POINT ( 'NONE',  ( 30.81806926056964002, 32.55937500034139731, 42.41743335407647209 ) ) ;
#819=ORIENTED_EDGE ( 'NONE', *, *, #13945, .T. ) ;
#821=CARTESIAN_POINT ( 'NONE',  ( 40.45084971874737079, 42.98125000068279888, -29.38926261462366440 ) ) ;
#824=ORIENTED_EDGE ( 'NONE', *, *, #7579, .T. ) ;
#837=CARTESIAN_POINT ( 'NONE',  ( -49.99999999999999289, 25.89999999999999858, -16.24598481164531449 ) ) ;
#839=CARTESIAN_POINT ( 'NONE',  ( -49.86468353124999453, 47.95937500034138878, 16.20201782572377525 ) ) ;
#844=CARTESIAN_POINT ( 'NONE',  ( 30.81806926056962936, 35.15937500034139873, -42.41743335407647209 ) ) ;
#852=CARTESIAN_POINT ( 'NONE',  ( 15.40903463028481113, 33.32187500034139305, -47.42413220539094709 ) ) ;
#855=CARTESIAN_POINT ( 'NONE',  ( 9.631387414534489405E-15, 40.42187500034138736, 52.43083105670540789 ) ) ;
#859=CARTESIAN_POINT ( 'NONE',  ( 49.86468353124999453, 42.95937500034139589, -16.20201782572376104 ) ) ;
#861=CARTESIAN_POINT ( 'NONE',  ( 30.90169943749475578, 22.48125000068279533, 42.53254041760200010 ) ) ;
#863=CARTESIAN_POINT ( 'NONE',  ( -40.34137639590981195, 42.12187500034139731, 29.30972558990012189 ) ) ;
#865=CARTESIAN_POINT ( 'NONE',  ( 15.45084971874736723, 41.40000000000000568, -47.55282581475768211 ) ) ;
#866=CARTESIAN_POINT ( 'NONE',  ( -49.86468353125000164, 25.92187500034139802, 0.000000000000000000 ) ) ;
#873=CARTESIAN_POINT ( 'NONE',  ( 40.34137639590981195, 37.12187500034139731, -29.30972558990011834 ) ) ;
#892=CARTESIAN_POINT ( 'NONE',  ( -30.81806926056963292, 31.55937500034139731, -42.41743335407647209 ) ) ;
#896=AXIS2_PLACEMENT_3D ( 'NONE', #7779, #2786, #3798 ) ;
#897=CARTESIAN_POINT ( 'NONE',  ( -40.45084971874737789, 41.58125000068280031, -29.38926261462365730 ) ) ;
#912=CARTESIAN_POINT ( 'NONE',  ( 30.90169943749475578, 26.70000000000000284, 42.53254041760200010 ) ) ;
#914=CARTESIAN_POINT ( 'NONE',  ( -40.45084971874737079, 44.20000000000000284, 29.38926261462367151 ) ) ;
#920=EDGE_LOOP ( 'NONE', ( #2916, #8700, #11462, #7137 ) ) ;
#922=CARTESIAN_POINT ( 'NONE',  ( -30.81806926056963292, 37.55937500034139020, -42.41743335407647209 ) ) ;
#924=CARTESIAN_POINT ( 'NONE',  ( 0.000000000000000000, 193.4213562373095385, -50.00000000000000000 ) ) ;
#931=CARTESIAN_POINT ( 'NONE',  ( -30.81806926056963292, 31.62187500034139731, -42.41743335407647209 ) ) ;
#932=CARTESIAN_POINT ( 'NONE',  ( 15.45084971874737789, 32.60000000000000142, 47.55282581475767500 ) ) ;
#934=CARTESIAN_POINT ( 'NONE',  ( -49.86468353124999453, 39.82187500034140015, -16.20201782572375393 ) ) ;
#938=CARTESIAN_POINT ( 'NONE',  ( -49.86468353124999453, 43.95937500034138878, 16.20201782572377169 ) ) ;
#940=CARTESIAN_POINT ( 'NONE',  ( -30.90169943749474868, 27.48125000068279888, -42.53254041760200721 ) ) ;
#945=CARTESIAN_POINT ( 'NONE',  ( 49.86468353124999453, 37.02187500034138878, -16.20201782572376104 ) ) ;
#947=PRODUCT_DEFINITION_FORMATION_WITH_SPECIFIED_SOURCE ( 'ANY', '', #7717, .NOT_KNOWN. ) ;
#949=CARTESIAN_POINT ( 'NONE',  ( 40.34137639590981905, 20.72187500034139873, 29.30972558990010768 ) ) ;
#957=CARTESIAN_POINT ( 'NONE',  ( 9.631387414534489405E-15, 38.42187500034139447, 52.43083105670540789 ) ) ;
#966=CARTESIAN_POINT ( 'NONE',  ( -49.99999999999999289, 49.89999999999999147, -16.24598481164531449 ) ) ;
#971=CARTESIAN_POINT ( 'NONE',  ( 0.000000000000000000, 25.00000000000000000, 0.000000000000000000 ) ) ;
#974=DIRECTION ( 'NONE',  ( 0.000000000000000000, 0.000000000000000000, -1.000000000000000000 ) ) ;
#978=CARTESIAN_POINT ( 'NONE',  ( -49.86468353124999453, 21.75937500034140015, -16.20201782572375393 ) ) ;
#980=EDGE_LOOP ( 'NONE', ( #7460, #8207, #4357, #5512 ) ) ;
#981=ORIENTED_EDGE ( 'NONE', *, *, #4267, .T. ) ;
#983=CARTESIAN_POINT ( 'NONE',  ( -49.99999999999999289, 45.88125000068279746, 16.24598481164533226 ) ) ;
#985=ORIENTED_EDGE ( 'NONE', *, *, #3765, .T. ) ;
#986=CARTESIAN_POINT ( 'NONE',  ( 1.293669679204937499E-13, 39.28125000068280315, -50.00000000000000000 ) ) ;
#992=FACE_OUTER_BOUND ( 'NONE', #13500, .T. ) ;
#993=CARTESIAN_POINT ( 'NONE',  ( 40.45084971874737789, 36.58125000068280031, 29.38926261462365375 ) ) ;
#994=CARTESIAN_POINT ( 'NONE',  ( -49.99999999999999289, 41.90000000000000568, -16.24598481164531449 ) ) ;
#997=CARTESIAN_POINT ( 'NONE',  ( -15.45084971874737256, 31.60000000000000142, -47.55282581475767500 ) ) ;
#1000=CARTESIAN_POINT ( 'NONE',  ( -3.210462471511496205E-15, 43.35937500034138736, -52.43083105670540789 ) ) ;
#1001=VERTEX_POINT ( 'NONE', #7172 ) ;
#1006=CARTESIAN_POINT ( 'NONE',  ( 49.86468353125000164, 32.85937500034139447, -6.106662507704105588E-15 ) ) ;
#1012=CARTESIAN_POINT ( 'NONE',  ( 40.45084971874737079, 44.98125000068279888, -29.38926261462366440 ) ) ;
#1021=CARTESIAN_POINT ( 'NONE',  ( 40.34137639590981195, 37.12187500034139731, -29.30972558990011834 ) ) ;
#1024=ADVANCED_FACE ( 'NONE', ( #5926 ), #3253, .T. ) ;
#1025=CARTESIAN_POINT ( 'NONE',  ( -49.86468353125000164, 41.85937500034139447, 0.000000000000000000 ) ) ;
#1027=CARTESIAN_POINT ( 'NONE',  ( -40.45084971874737789, 21.58125000068279675, -29.38926261462365730 ) ) ;
#1032=CARTESIAN_POINT ( 'NONE',  ( 49.86468353125000164, 22.92187500034139802, -6.106662507704105588E-15 ) ) ;
#1038=CARTESIAN_POINT ( 'NONE',  ( -15.40903463028481646, 37.52187500034139589, -47.42413220539093999 ) ) ;
#1059=CARTESIAN_POINT ( 'NONE',  ( 40.34137639590981195, 27.05937500034139731, -29.30972558990011834 ) ) ;
#1060=EDGE_LOOP ( 'NONE', ( #3862, #4804, #10733, #13726 ) ) ;
#1062=VERTEX_POINT ( 'NONE', #8489 ) ;
#1063=CARTESIAN_POINT ( 'NONE',  ( -15.45084971874737256, 39.38125000068279746, -47.55282581475767500 ) ) ;
#1064=CARTESIAN_POINT ( 'NONE',  ( 15.45084971874736723, 47.40000000000000568, -47.55282581475768211 ) ) ;
#1068=CARTESIAN_POINT ( 'NONE',  ( -40.45084971874737079, 38.20000000000000284, 29.38926261462367151 ) ) ;
#1072=DIRECTION ( 'NONE',  ( -0.000000000000000000, -1.000000000000000000, -0.000000000000000000 ) ) ;
#1077=DIRECTION ( 'NONE',  ( -0.000000000000000000, -1.000000000000000000, -0.000000000000000000 ) ) ;
#1078=CARTESIAN_POINT ( 'NONE',  ( 40.45084971874737789, 28.80000000000000426, 29.38926261462365375 ) ) ;
#1082=CARTESIAN_POINT ( 'NONE',  ( -30.81806926056962226, 46.15937500034139873, 42.41743335407647919 ) ) ;
#1087=CARTESIAN_POINT ( 'NONE',  ( -15.40903463028480580, 34.25937500034139305, 47.42413220539094709 ) ) ;
#1090=CARTESIAN_POINT ( 'NONE',  ( 47.74744883082096436, 24.99999999999999289, -14.37691108325706679 ) ) ;
#1091=CARTESIAN_POINT ( 'NONE',  ( 49.99999999999999289, 46.88125000068279036, -16.24598481164532160 ) ) ;
#1098=CARTESIAN_POINT ( 'NONE',  ( -30.81806926056962226, 36.22187500034139873, 42.41743335407647919 ) ) ;
#1102=CARTESIAN_POINT ( 'NONE',  ( -15.40903463028481646, 41.45937500034140299, -47.42413220539093999 ) ) ;
#1104=CARTESIAN_POINT ( 'NONE',  ( 40.45084971874737789, 22.58125000068279675, 29.38926261462365375 ) ) ;
#1108=CARTESIAN_POINT ( 'NONE',  ( -2.547328955960238000E-13, 30.49999999999999645, 49.99999999999999289 ) ) ;
#1110=CARTESIAN_POINT ( 'NONE',  ( 30.81806926056964002, 24.62187500034139731, 42.41743335407647209 ) ) ;
#1116=CARTESIAN_POINT ( 'NONE',  ( -40.34137639590981195, 34.12187500034139731, 29.30972558990012189 ) ) ;
#1121=VERTEX_POINT ( 'NONE', #6248 ) ;
#1132=CARTESIAN_POINT ( 'NONE',  ( -50.00000000000000000, 35.78125000068280315, 0.000000000000000000 ) ) ;
#1135=CARTESIAN_POINT ( 'NONE',  ( -49.86468353125000164, 27.85937500034139447, 0.000000000000000000 ) ) ;
#1136=CARTESIAN_POINT ( 'NONE',  ( -49.99999999999999289, 47.88125000068281167, 16.24598481164533226 ) ) ;
#1138=VERTEX_POINT ( 'NONE', #14043 ) ;
#1140=CARTESIAN_POINT ( 'NONE',  ( -15.45084971874736368, 36.18125000068280173, 47.55282581475768211 ) ) ;
#1142=ADVANCED_FACE ( 'NONE', ( #7415 ), #13717, .T. ) ;
#1146=CARTESIAN_POINT ( 'NONE',  ( 40.45084971874737789, 38.58125000068280031, 29.38926261462365375 ) ) ;
#1156=CARTESIAN_POINT ( 'NONE',  ( 40.45084971874737079, 23.20000000000000284, -29.38926261462366440 ) ) ;
#1158=CARTESIAN_POINT ( 'NONE',  ( -5.823736356558307894E-14, 44.50000000000000000, 50.00000000000000000 ) ) ;
#1160=CARTESIAN_POINT ( 'NONE',  ( -49.86468353124999453, 41.95937500034138878, 16.20201782572377525 ) ) ;
#1162=ORIENTED_EDGE ( 'NONE', *, *, #8619, .T. ) ;
#1164=CARTESIAN_POINT ( 'NONE',  ( -15.40903463028480580, 30.25937500034140015, 47.42413220539094709 ) ) ;
#1169=CARTESIAN_POINT ( 'NONE',  ( 48.02615145421076193, 25.00000000000000000, -13.41652781627779234 ) ) ;
#1179=CARTESIAN_POINT ( 'NONE',  ( 49.86468353124999453, 29.02187500034139234, -16.20201782572376459 ) ) ;
#1183=CARTESIAN_POINT ( 'NONE',  ( 30.81806926056964002, 34.55937500034139731, 42.41743335407646498 ) ) ;
#1186=CARTESIAN_POINT ( 'NONE',  ( 15.45084971874736723, 23.18125000068279817, -47.55282581475768211 ) ) ;
#1188=CARTESIAN_POINT ( 'NONE',  ( 9.631387414534489405E-15, 22.42187500034139802, 52.43083105670540789 ) ) ;
#1189=DIRECTION ( 'NONE',  ( 0.000000000000000000, 1.000000000000000000, 0.000000000000000000 ) ) ;
#1192=AXIS2_PLACEMENT_3D ( 'NONE', #11874, #15769, #13204 ) ;
#1193=CARTESIAN_POINT ( 'NONE',  ( -15.45084971874736368, 46.40000000000000568, 47.55282581475768211 ) ) ;
#1195=CARTESIAN_POINT ( 'NONE',  ( -30.81806926056963292, 49.62187500034139020, -42.41743335407647209 ) ) ;
#1198=CARTESIAN_POINT ( 'NONE',  ( 15.40903463028482356, 38.52187500034139589, 47.42413220539093999 ) ) ;
#1203=CIRCLE ( 'NONE', #13968, 42.00000000000000711 ) ;
#1224=CARTESIAN_POINT ( 'NONE',  ( 40.34137639590981905, 22.65937500034139518, 29.30972558990010768 ) ) ;
#1235=CARTESIAN_POINT ( 'NONE',  ( 1.293669679204937499E-13, 37.50000000000000711, -50.00000000000000000 ) ) ;
#1238=CARTESIAN_POINT ( 'NONE',  ( 30.90169943749475223, 26.48125000068279888, 42.53254041760199300 ) ) ;
#1240=CYLINDRICAL_SURFACE ( 'NONE', #6816, 50.00000000000000000 ) ;
#1244=CARTESIAN_POINT ( 'NONE',  ( 50.00000000000000711, 24.90000000000000213, 16.24598481164530739 ) ) ;
#1248=CARTESIAN_POINT ( 'NONE',  ( -3.210462471511496205E-15, 41.35937500034138736, -52.43083105670540789 ) ) ;
#1254=CARTESIAN_POINT ( 'NONE',  ( 49.86468353125001585, 26.75937500034139660, 16.20201782572375038 ) ) ;
#1258=CARTESIAN_POINT ( 'NONE',  ( 47.88920767661677047, 25.00000000000000000, -13.89741811465768428 ) ) ;
#1259=ADVANCED_BREP_SHAPE_REPRESENTATION ( '', ( #3161, #15812 ), #11844 ) ;
#1260=CARTESIAN_POINT ( 'NONE',  ( -3.210462471511496205E-15, 37.42187500034140157, -52.43083105670540789 ) ) ;
#1261=( BOUNDED_CURVE ( )  B_SPLINE_CURVE ( 2, ( #986, #7239, #9979, #6086, #8722, #5011, #13788, #12548, #1146, #3741, #8803, #13866, #7164 ),
 .UNSPECIFIED., .F., .F. ) 
 B_SPLINE_CURVE_WITH_KNOTS ( ( 3, 2, 2, 2, 2, 2, 3 ),
 ( 0.3500000000000000333, 0.3533333333333333326, 0.3599999999999999867, 0.3666666666666666408, 0.3733333333333333504, 0.3800000000000000044, 0.3833333333333333592 ),
 .UNSPECIFIED. ) 
 CURVE ( )  GEOMETRIC_REPRESENTATION_ITEM ( )  RATIONAL_B_SPLINE_CURVE ( ( 0.9755282581475768211, 0.9755282581475770431, 1.000000000000000000, 0.9510565162951535312, 1.000000000000000000, 0.9510565162951535312, 1.000000000000000000, 0.9510565162951535312, 1.000000000000000000, 0.9510565162951535312, 1.000000000000000000, 0.9755282581475765991, 0.9755282581475768211 ) ) 
 REPRESENTATION_ITEM ( '' )  );
#1269=CARTESIAN_POINT ( 'NONE',  ( 40.34137639590981905, 32.72187500034139873, 29.30972558990010768 ) ) ;
#1274=CARTESIAN_POINT ( 'NONE',  ( 30.81806926056962936, 35.15937500034139873, -42.41743335407646498 ) ) ;
#1275=VERTEX_POINT ( 'NONE', #13128 ) ;
#1278=CARTESIAN_POINT ( 'NONE',  ( -49.86468353124999453, 45.75937500034140015, -16.20201782572375393 ) ) ;
#1280=CARTESIAN_POINT ( 'NONE',  ( 49.86468353125000164, 22.92187500034139802, -6.106662507704105588E-15 ) ) ;
#1284=CARTESIAN_POINT ( 'NONE',  ( -50.00000000000000000, 25.78125000068279959, 0.000000000000000000 ) ) ;
#1285=CARTESIAN_POINT ( 'NONE',  ( 49.99999999999999289, 47.10000000000000853, -16.24598481164532160 ) ) ;
#1297=EDGE_CURVE ( 'NONE', #4024, #14468, #9336, .T. ) ;
#1306=CARTESIAN_POINT ( 'NONE',  ( -15.40903463028480580, 22.25937500034139660, 47.42413220539094709 ) ) ;
#1307=ORIENTED_EDGE ( 'NONE', *, *, #9049, .T. ) ;
#1315=CARTESIAN_POINT ( 'NONE',  ( -50.00000000000000000, 38.00000000000000711, 0.000000000000000000 ) ) ;
#1324=CARTESIAN_POINT ( 'NONE',  ( -49.99999999999999289, 24.10000000000000142, 16.24598481164533226 ) ) ;
#1327=CARTESIAN_POINT ( 'NONE',  ( 9.631387414534489405E-15, 46.35937500034139447, 52.43083105670540789 ) ) ;
#1332=CARTESIAN_POINT ( 'NONE',  ( -40.34137639590981195, 26.05937500034139731, 29.30972558990012189 ) ) ;
#1338=CARTESIAN_POINT ( 'NONE',  ( 48.33688377893788157, 25.00000000000000000, -12.24883938693806229 ) ) ;
#1339=CARTESIAN_POINT ( 'NONE',  ( -49.86468353125000164, 31.92187500034139447, 0.000000000000000000 ) ) ;
#1347=CARTESIAN_POINT ( 'NONE',  ( -40.34137639590981905, 31.72187500034139873, -29.30972558990011478 ) ) ;
#1349=ORIENTED_EDGE ( 'NONE', *, *, #2891, .T. ) ;
#1351=CARTESIAN_POINT ( 'NONE',  ( -49.86468353125000164, 35.85937500034140157, 0.000000000000000000 ) ) ;
#1352=VERTEX_POINT ( 'NONE', #9237 ) ;
#1356=CARTESIAN_POINT ( 'NONE',  ( -50.00000000000000000, 19.78125000068279604, 0.000000000000000000 ) ) ;
#1360=CARTESIAN_POINT ( 'NONE',  ( 49.86468353125000164, 20.92187500034139802, -6.106662507704105588E-15 ) ) ;
#1365=CARTESIAN_POINT ( 'NONE',  ( 15.45084971874737789, 46.60000000000000142, 47.55282581475767500 ) ) ;
#1370=CARTESIAN_POINT ( 'NONE',  ( 0.000000000000000000, 51.99999999999999289, 0.000000000000000000 ) ) ;
#1383=CARTESIAN_POINT ( 'NONE',  ( 40.45084971874737789, 34.58125000068280031, 29.38926261462365375 ) ) ;
#1388=CARTESIAN_POINT ( 'NONE',  ( -30.81806926056963292, 21.55937500034140086, -42.41743335407647209 ) ) ;
#1390=CARTESIAN_POINT ( 'NONE',  ( -15.45084971874736368, 26.40000000000000213, 47.55282581475768211 ) ) ;
#1395=CARTESIAN_POINT ( 'NONE',  ( -15.45084971874736368, 28.40000000000000213, 47.55282581475768211 ) ) ;
#1405=CARTESIAN_POINT ( 'NONE',  ( 50.00000000000000000, 25.00000000000000000, -6.123233995736766085E-15 ) ) ;
#1406=DIRECTION ( 'NONE',  ( -0.000000000000000000, -1.000000000000000000, -0.000000000000000000 ) ) ;
#1408=CARTESIAN_POINT ( 'NONE',  ( -15.40903463028480580, 38.25937500034140015, 47.42413220539094709 ) ) ;
#1413=CARTESIAN_POINT ( 'NONE',  ( 40.34137639590981905, 30.65937500034139518, 29.30972558990010768 ) ) ;
#1418=CARTESIAN_POINT ( 'NONE',  ( 47.39803307437463786, 25.00000000000000000, -15.49002591438228293 ) ) ;
#1419=CARTESIAN_POINT ( 'NONE',  ( 15.40903463028481113, 37.32187500034140015, -47.42413220539094709 ) ) ;
#1420=CARTESIAN_POINT ( 'NONE',  ( 7.919222016226807881, 46.33250428222964246, 50.00000000000000000 ) ) ;
#1430=CARTESIAN_POINT ( 'NONE',  ( 40.34137639590981195, 31.12187500034139731, -29.30972558990011834 ) ) ;
#1432=EDGE_CURVE ( 'NONE', #8369, #9508, #559, .T. ) ;
#1436=CARTESIAN_POINT ( 'NONE',  ( -30.81806926056962226, 36.15937500034139163, 42.41743335407647209 ) ) ;
#1440=CARTESIAN_POINT ( 'NONE',  ( -30.81806926056963292, 45.55937500034139731, -42.41743335407647209 ) ) ;
#1443=CARTESIAN_POINT ( 'NONE',  ( 40.34137639590981905, 24.72187500034139873, 29.30972558990010768 ) ) ;
#1448=CARTESIAN_POINT ( 'NONE',  ( -30.90169943749474868, 49.70000000000000284, -42.53254041760200721 ) ) ;
#1453=( BOUNDED_CURVE ( )  B_SPLINE_CURVE ( 2, ( #4655, #4750, #9560, #12463, #7064, #9808, #12376, #14859, #3404, #9724, #13611, #6148, #14605 ),
 .UNSPECIFIED., .F., .F. ) 
 B_SPLINE_CURVE_WITH_KNOTS ( ( 3, 2, 2, 2, 2, 2, 3 ),
 ( 0.5166666666666667185, 0.5200000000000000178, 0.5266666666666666163, 0.5333333333333333259, 0.5400000000000000355, 0.5466666666666666341, 0.5500000000000000444 ),
 .UNSPECIFIED. ) 
 CURVE ( )  GEOMETRIC_REPRESENTATION_ITEM ( )  RATIONAL_B_SPLINE_CURVE ( ( 0.9755282581475768211, 0.9755282581475771542, 1.000000000000000000, 0.9510565162951535312, 1.000000000000000000, 0.9510565162951535312, 1.000000000000000000, 0.9510565162951535312, 1.000000000000000000, 0.9510565162951535312, 1.000000000000000000, 0.9755282581475763770, 0.9755282581475768211 ) ) 
 REPRESENTATION_ITEM ( '' )  );
#1456=CARTESIAN_POINT ( 'NONE',  ( -30.90169943749474868, 39.48125000068278467, -42.53254041760200721 ) ) ;
#1463=CARTESIAN_POINT ( 'NONE',  ( 15.40903463028481113, 49.32187500034139305, -47.42413220539094709 ) ) ;
#1469=CARTESIAN_POINT ( 'NONE',  ( 50.00000000000000000, 25.00000000000000000, -6.123233995736766085E-15 ) ) ;
#1472=ORIENTED_EDGE ( 'NONE', *, *, #10992, .T. ) ;
#1474=CARTESIAN_POINT ( 'NONE',  ( -30.81806926056962226, 46.22187500034139163, 42.41743335407647919 ) ) ;
#1478=EDGE_LOOP ( 'NONE', ( #4757, #9240, #1605, #15687, #2456, #2395, #11688, #12194 ) ) ;
#1483=CARTESIAN_POINT ( 'NONE',  ( -40.45084971874737079, 28.20000000000000284, 29.38926261462367151 ) ) ;
#1488=VECTOR ( 'NONE', #16400, 1000.000000000000000 ) ;
#1489=CARTESIAN_POINT ( 'NONE',  ( 30.90169943749473802, 49.08125000068280031, -42.53254041760200721 ) ) ;
#1492=AXIS2_PLACEMENT_3D ( 'NONE', #15123, #13345, #9612 ) ;
#1494=( GEOMETRIC_REPRESENTATION_CONTEXT ( 3 ) GLOBAL_UNCERTAINTY_ASSIGNED_CONTEXT ( ( #9092 ) ) GLOBAL_UNIT_ASSIGNED_CONTEXT ( ( #11140, #9883, #15945 ) ) REPRESENTATION_CONTEXT ( 'NONE', 'WORKASPACE' ) );
#1500=CARTESIAN_POINT ( 'NONE',  ( 49.86468353125001585, 34.75937500034139305, 16.20201782572375038 ) ) ;
#1505=CARTESIAN_POINT ( 'NONE',  ( 15.45084971874736723, 47.18125000068280173, -47.55282581475768211 ) ) ;
#1507=CARTESIAN_POINT ( 'NONE',  ( 30.81806926056964002, 30.55937500034139731, 42.41743335407647209 ) ) ;
#1512=CARTESIAN_POINT ( 'NONE',  ( -30.81806926056962226, 34.22187500034139163, 42.41743335407647209 ) ) ;
#1513=EDGE_CURVE ( 'NONE', #326, #15172, #4405, .T. ) ;
#1523=CARTESIAN_POINT ( 'NONE',  ( 15.40903463028481113, 29.32187500034139660, -47.42413220539094709 ) ) ;
#1526=CARTESIAN_POINT ( 'NONE',  ( 49.86468353125000164, 36.85937500034139447, -6.106662507704105588E-15 ) ) ;
#1529=CARTESIAN_POINT ( 'NONE',  ( -49.86468353124999453, 47.95937500034138878, 16.20201782572377525 ) ) ;
#1531=CARTESIAN_POINT ( 'NONE',  ( -15.40903463028481646, 23.52187500034139944, -47.42413220539093999 ) ) ;
#1538=CARTESIAN_POINT ( 'NONE',  ( -40.34137639590981195, 20.12187500034139731, 29.30972558990012189 ) ) ;
#1541=CARTESIAN_POINT ( 'NONE',  ( 9.631387414534489405E-15, 48.42187500034140157, 52.43083105670540789 ) ) ;
#1545=ORIENTED_EDGE ( 'NONE', *, *, #9863, .F. ) ;
#1546=CARTESIAN_POINT ( 'NONE',  ( -30.90169943749474868, 35.48125000068279888, -42.53254041760200721 ) ) ;
#1551=CARTESIAN_POINT ( 'NONE',  ( 49.86468353124999453, 47.02187500034139589, -16.20201782572376104 ) ) ;
#1560=CARTESIAN_POINT ( 'NONE',  ( -3.210462471511496205E-15, 49.42187500034138736, -52.43083105670540789 ) ) ;
#1568=CARTESIAN_POINT ( 'NONE',  ( 15.45084971874736723, 29.40000000000000213, -47.55282581475768211 ) ) ;
#1576=CARTESIAN_POINT ( 'NONE',  ( 0.000000000000000000, 272.0000000000000000, 0.000000000000000000 ) ) ;
#1582=CARTESIAN_POINT ( 'NONE',  ( 49.86468353124999453, 36.95937500034139589, -16.20201782572376459 ) ) ;
#1585=CARTESIAN_POINT ( 'NONE',  ( 30.90169943749475578, 48.48125000068279888, 42.53254041760200010 ) ) ;
#1586=CARTESIAN_POINT ( 'NONE',  ( 8.446640517145639571E-15, 28.49999999999999645, 50.00000000000000000 ) ) ;
#1587=CARTESIAN_POINT ( 'NONE',  ( 49.86468353124999453, 20.95937500034138878, -16.20201782572376459 ) ) ;
#1588=ORIENTED_EDGE ( 'NONE', *, *, #13663, .F. ) ;
#1589=CARTESIAN_POINT ( 'NONE',  ( 7.919222016226809657, 27.44874571845315003, -50.00000000000000000 ) ) ;
#1592=CARTESIAN_POINT ( 'NONE',  ( -30.81806926056962226, 28.22187500034139873, 42.41743335407647209 ) ) ;
#1598=CARTESIAN_POINT ( 'NONE',  ( -50.00000000000000000, 36.00000000000000711, 0.000000000000000000 ) ) ;
#1600=CARTESIAN_POINT ( 'NONE',  ( 30.81806926056962936, 27.22187500034139518, -42.41743335407647209 ) ) ;
#1604=CARTESIAN_POINT ( 'NONE',  ( 30.81806926056962936, 27.15937500034139163, -42.41743335407646498 ) ) ;
#1605=ORIENTED_EDGE ( 'NONE', *, *, #9196, .T. ) ;
#1607=CARTESIAN_POINT ( 'NONE',  ( -30.81806926056963292, 43.55937500034139731, -42.41743335407647209 ) ) ;
#1614=CARTESIAN_POINT ( 'NONE',  ( -40.45084971874737079, 38.20000000000000284, 29.38926261462367151 ) ) ;
#1617=CARTESIAN_POINT ( 'NONE',  ( 49.86468353125001585, 46.82187500034139305, 16.20201782572375038 ) ) ;
#1619=CARTESIAN_POINT ( 'NONE',  ( -49.86468353125000164, 47.85937500034139447, 0.000000000000000000 ) ) ;
#1621=CARTESIAN_POINT ( 'NONE',  ( 9.657523855033129090E-15, 34.28125000068278894, 52.57311121191334990 ) ) ;
#1624=CARTESIAN_POINT ( 'NONE',  ( 0.000000000000000000, 272.0000000000000000, -82.49773270518484480 ) ) ;
#1626=CARTESIAN_POINT ( 'NONE',  ( 50.00000000000000000, 32.78125000068279604, -6.123233995736766085E-15 ) ) ;
#1627=CARTESIAN_POINT ( 'NONE',  ( 49.86468353125001585, 44.82187500034139305, 16.20201782572375038 ) ) ;
#1629=CARTESIAN_POINT ( 'NONE',  ( -30.90169943749474513, 39.48125000068278467, -42.53254041760200721 ) ) ;
#1631=FACE_OUTER_BOUND ( 'NONE', #14650, .T. ) ;
#1632=ADVANCED_FACE ( 'NONE', ( #12769 ), #7108, .T. ) ;
#1638=CARTESIAN_POINT ( 'NONE',  ( 30.81806926056964002, 48.62187500034139731, 42.41743335407647209 ) ) ;
#1639=VERTEX_POINT ( 'NONE', #1891 ) ;
#1640=CARTESIAN_POINT ( 'NONE',  ( -7.919222016226804328, 26.44874571845315359, 50.00000000000000000 ) ) ;
#1642=ORIENTED_EDGE ( 'NONE', *, *, #3754, .T. ) ;
#1649=DIRECTION ( 'NONE',  ( -0.000000000000000000, -1.000000000000000000, -0.000000000000000000 ) ) ;
#1650=CARTESIAN_POINT ( 'NONE',  ( -30.90169943749473447, 46.30000000000000426, 42.53254041760200721 ) ) ;
#1652=CARTESIAN_POINT ( 'NONE',  ( -3.111920190527341144E-15, 43.28125000068280315, -50.00000000000000000 ) ) ;
#1655=AXIS2_PLACEMENT_3D ( 'NONE', #14370, #1406, #6837 ) ;
#1659=CARTESIAN_POINT ( 'NONE',  ( 49.86468353125000164, 36.85937500034139447, -6.106662507704105588E-15 ) ) ;
#1665=CARTESIAN_POINT ( 'NONE',  ( -49.86468353124999453, 19.95937500034138878, 16.20201782572377525 ) ) ;
#1666=VECTOR ( 'NONE', #3718, 1000.000000000000000 ) ;
#1668=CARTESIAN_POINT ( 'NONE',  ( 0.000000000000000000, 252.1309828287255357, 0.000000000000000000 ) ) ;
#1669=CARTESIAN_POINT ( 'NONE',  ( 15.45084971874736723, 35.39999999999999858, -47.55282581475768211 ) ) ;
#1671=CARTESIAN_POINT ( 'NONE',  ( 49.86468353124999453, 29.02187500034139234, -16.20201782572376104 ) ) ;
#1677=CARTESIAN_POINT ( 'NONE',  ( 30.90169943749474157, 37.30000000000000426, -42.53254041760200721 ) ) ;
#1681=ORIENTED_EDGE ( 'NONE', *, *, #11408, .T. ) ;
#1683=CARTESIAN_POINT ( 'NONE',  ( -3.210462471511496205E-15, 31.35937500034138736, -52.43083105670540789 ) ) ;
#1687=CARTESIAN_POINT ( 'NONE',  ( -49.86468353125000164, 43.85937500034140157, 0.000000000000000000 ) ) ;
#1695=CARTESIAN_POINT ( 'NONE',  ( -40.45084971874737079, 42.20000000000000284, 29.38926261462367151 ) ) ;
#1697=CARTESIAN_POINT ( 'NONE',  ( 49.86468353125000164, 42.92187500034140157, -6.106662507704105588E-15 ) ) ;
#1703=CARTESIAN_POINT ( 'NONE',  ( -30.90169943749474868, 33.48125000068279888, -42.53254041760200721 ) ) ;
#1706=CARTESIAN_POINT ( 'NONE',  ( 0.000000000000000000, 193.4213562373095385, -50.00000000000000000 ) ) ;
#1707=CARTESIAN_POINT ( 'NONE',  ( 40.45084971874737079, 32.98125000068279888, -29.38926261462366440 ) ) ;
#1708=CARTESIAN_POINT ( 'NONE',  ( 40.34137639590981905, 48.72187500034139873, 29.30972558990010768 ) ) ;
#1710=CARTESIAN_POINT ( 'NONE',  ( 5.143516556418884111E-15, 272.0000000000000000, 42.00000000000000711 ) ) ;
#1711=AXIS2_PLACEMENT_3D ( 'NONE', #16274, #4910, #12536 ) ;
#1718=CARTESIAN_POINT ( 'NONE',  ( -30.81806926056962226, 20.15937500034139518, 42.41743335407647919 ) ) ;
#1720=DIRECTION ( 'NONE',  ( 0.000000000000000000, 0.000000000000000000, 1.000000000000000000 ) ) ;
#1721=EDGE_LOOP ( 'NONE', ( #9897, #11430, #1349, #3595 ) ) ;
#1725=EDGE_CURVE ( 'NONE', #13481, #11385, #10478, .T. ) ;
#1737=FACE_OUTER_BOUND ( 'NONE', #736, .T. ) ;
#1739=ORIENTED_EDGE ( 'NONE', *, *, #16001, .F. ) ;
#1741=CARTESIAN_POINT ( 'NONE',  ( 30.81806926056964002, 36.55937500034139731, 42.41743335407647209 ) ) ;
#1746=CARTESIAN_POINT ( 'NONE',  ( 49.86468353125000164, 22.85937500034139802, -6.106662507704105588E-15 ) ) ;
#1751=CARTESIAN_POINT ( 'NONE',  ( 40.45084971874737079, 35.20000000000000284, -29.38926261462366440 ) ) ;
#1754=CARTESIAN_POINT ( 'NONE',  ( -30.81806926056963292, 25.62187500034139731, -42.41743335407646498 ) ) ;
#1760=CARTESIAN_POINT ( 'NONE',  ( -3.219174618344376363E-15, 33.50000000000000711, -52.57311121191334990 ) ) ;
#1767=VERTEX_POINT ( 'NONE', #8620 ) ;
#1768=CARTESIAN_POINT ( 'NONE',  ( -40.34137639590981905, 29.65937500034139518, -29.30972558990011478 ) ) ;
#1771=CARTESIAN_POINT ( 'NONE',  ( 40.34137639590981195, 43.05937500034139731, -29.30972558990011834 ) ) ;
#1773=VECTOR ( 'NONE', #10170, 1000.000000000000000 ) ;
#1780=CARTESIAN_POINT ( 'NONE',  ( 50.00000000000000711, 38.89999999999999858, 16.24598481164530739 ) ) ;
#1783=CARTESIAN_POINT ( 'NONE',  ( -40.34137639590981905, 41.72187500034139873, -29.30972558990011478 ) ) ;
#1787=CARTESIAN_POINT ( 'NONE',  ( 30.81806926056962936, 49.15937500034139163, -42.41743335407646498 ) ) ;
#1789=CARTESIAN_POINT ( 'NONE',  ( 50.00000000000000000, 28.78125000068279959, -6.123233995736766085E-15 ) ) ;
#1792=CARTESIAN_POINT ( 'NONE',  ( 30.90169943749475223, 32.48125000068280599, 42.53254041760199300 ) ) ;
#1793=CARTESIAN_POINT ( 'NONE',  ( -15.40903463028480580, 42.32187500034139305, 47.42413220539094709 ) ) ;
#1801=CARTESIAN_POINT ( 'NONE',  ( -40.45084971874737789, 45.58125000068280031, -29.38926261462365730 ) ) ;
#1803=CARTESIAN_POINT ( 'NONE',  ( -30.81806926056962226, 44.22187500034139163, 42.41743335407647919 ) ) ;
#1806=EDGE_CURVE ( 'NONE', #7158, #15132, #8259, .T. ) ;
#1807=CARTESIAN_POINT ( 'NONE',  ( -5.823736356558309156E-14, 44.28125000068280315, 50.00000000000000000 ) ) ;
#1814=CARTESIAN_POINT ( 'NONE',  ( -15.45084971874737256, 45.60000000000000142, -47.55282581475767500 ) ) ;
#1818=EDGE_CURVE ( 'NONE', #7740, #9508, #1453, .T. ) ;
#1820=CARTESIAN_POINT ( 'NONE',  ( -40.34137639590981195, 30.05937500034139731, 29.30972558990012189 ) ) ;
#1828=CARTESIAN_POINT ( 'NONE',  ( 15.45084971874737789, 34.60000000000000853, 47.55282581475767500 ) ) ;
#1830=CARTESIAN_POINT ( 'NONE',  ( -40.34137639590981195, 30.12187500034139731, 29.30972558990012189 ) ) ;
#1837=CARTESIAN_POINT ( 'NONE',  ( -30.90169943749474868, 35.69999999999999574, -42.53254041760200721 ) ) ;
#1839=CYLINDRICAL_SURFACE ( 'NONE', #13610, 50.00000000000000000 ) ;
#1840=VERTEX_POINT ( 'NONE', #7795 ) ;
#1842=CARTESIAN_POINT ( 'NONE',  ( 49.86468353124999453, 30.95937500034139944, -16.20201782572376104 ) ) ;
#1844=DIRECTION ( 'NONE',  ( -0.000000000000000000, -1.000000000000000000, -0.000000000000000000 ) ) ;
#1845=CARTESIAN_POINT ( 'NONE',  ( -40.34137639590981195, 40.05937500034140442, 29.30972558990012189 ) ) ;
#1846=AXIS2_PLACEMENT_3D ( 'NONE', #12793, #145, #15039 ) ;
#1847=CARTESIAN_POINT ( 'NONE',  ( -49.86468353124999453, 20.02187500034139589, 16.20201782572377525 ) ) ;
#1852=CARTESIAN_POINT ( 'NONE',  ( 49.86468353124999453, 29.02187500034139234, -16.20201782572376459 ) ) ;
#1853=CARTESIAN_POINT ( 'NONE',  ( 9.657523855033129090E-15, 40.50000000000000711, 52.57311121191334990 ) ) ;
#1855=CARTESIAN_POINT ( 'NONE',  ( 40.34137639590981195, 45.12187500034139731, -29.30972558990011834 ) ) ;
#1860=CARTESIAN_POINT ( 'NONE',  ( -40.34137639590981195, 46.05937500034139731, 29.30972558990012189 ) ) ;
#1862=CARTESIAN_POINT ( 'NONE',  ( 50.00000000000000711, 28.68125000068279462, 16.24598481164530739 ) ) ;
#1863=VERTEX_POINT ( 'NONE', #6315 ) ;
#1866=CARTESIAN_POINT ( 'NONE',  ( -49.86468353125000164, 41.92187500034139447, 0.000000000000000000 ) ) ;
#1871=EDGE_CURVE ( 'NONE', #1062, #5162, #15872, .T. ) ;
#1875=ORIENTED_EDGE ( 'NONE', *, *, #125, .F. ) ;
#1876=CARTESIAN_POINT ( 'NONE',  ( 49.86468353125001585, 40.82187500034140726, 16.20201782572375038 ) ) ;
#1880=EDGE_CURVE ( 'NONE', #3644, #8369, #7005, .T. ) ;
#1882=DIRECTION ( 'NONE',  ( -0.000000000000000000, -1.000000000000000000, -0.000000000000000000 ) ) ;
#1889=CARTESIAN_POINT ( 'NONE',  ( 0.000000000000000000, 193.4213562373095385, 0.000000000000000000 ) ) ;
#1891=CARTESIAN_POINT ( 'NONE',  ( 0.000000000000000000, 252.1309828287255357, 79.49773270518484480 ) ) ;
#1892=CARTESIAN_POINT ( 'NONE',  ( 49.99999999999999289, 37.10000000000000142, -16.24598481164532160 ) ) ;
#1894=CARTESIAN_POINT ( 'NONE',  ( 49.86468353125001585, 28.75937500034139305, 16.20201782572375038 ) ) ;
#1898=CARTESIAN_POINT ( 'NONE',  ( 50.00000000000000000, 42.78125000068280315, -6.123233995736766085E-15 ) ) ;
#1900=CARTESIAN_POINT ( 'NONE',  ( -15.40903463028481646, 25.45937500034139589, -47.42413220539093999 ) ) ;
#1902=CARTESIAN_POINT ( 'NONE',  ( -15.45084971874737256, 27.38125000068280102, -47.55282581475767500 ) ) ;
#1905=CARTESIAN_POINT ( 'NONE',  ( 0.000000000000000000, 193.4213562373095385, 0.000000000000000000 ) ) ;
#1906=CARTESIAN_POINT ( 'NONE',  ( -49.86468353124999453, 29.82187500034139660, -16.20201782572375393 ) ) ;
#1912=CARTESIAN_POINT ( 'NONE',  ( -50.00000000000000000, 32.00000000000000000, 0.000000000000000000 ) ) ;
#1916=ADVANCED_FACE ( 'NONE', ( #9964 ), #7549, .T. ) ;
#1919=CARTESIAN_POINT ( 'NONE',  ( 30.81806926056962936, 29.15937500034139518, -42.41743335407646498 ) ) ;
#1922=CARTESIAN_POINT ( 'NONE',  ( 40.34137639590981905, 44.65937500034139163, 29.30972558990010768 ) ) ;
#1930=CARTESIAN_POINT ( 'NONE',  ( 9.631387414534489405E-15, 28.42187500034139092, 52.43083105670540789 ) ) ;
#1935=CARTESIAN_POINT ( 'NONE',  ( 30.81806926056964002, 44.62187500034140442, 42.41743335407647209 ) ) ;
#1939=FACE_OUTER_BOUND ( 'NONE', #2477, .T. ) ;
#1940=ORIENTED_EDGE ( 'NONE', *, *, #7735, .F. ) ;
#1942=CARTESIAN_POINT ( 'NONE',  ( -50.00000000000000000, 27.78125000068279959, 0.000000000000000000 ) ) ;
#1946=CARTESIAN_POINT ( 'NONE',  ( -40.34137639590981195, 38.12187500034139731, 29.30972558990012189 ) ) ;
#1950=AXIS2_PLACEMENT_3D ( 'NONE', #12374, #11049, #974 ) ;
#1952=CARTESIAN_POINT ( 'NONE',  ( -49.99999999999999289, 45.88125000068279746, 16.24598481164533226 ) ) ;
#1954=CARTESIAN_POINT ( 'NONE',  ( -49.86468353124999453, 39.82187500034140015, -16.20201782572375393 ) ) ;
#1960=CIRCLE ( 'NONE', #12861, 42.00000000000000711 ) ;
#1961=CARTESIAN_POINT ( 'NONE',  ( 0.000000000000000000, 55.00000000000000711, 62.25100647794772613 ) ) ;
#1966=DIRECTION ( 'NONE',  ( 0.000000000000000000, 1.000000000000000000, 0.000000000000000000 ) ) ;
#1970=CARTESIAN_POINT ( 'NONE',  ( 50.00000000000000711, 42.68125000068280173, 16.24598481164530739 ) ) ;
#1975=CARTESIAN_POINT ( 'NONE',  ( -30.81806926056963292, 29.55937500034139376, -42.41743335407647209 ) ) ;
#1976=EDGE_LOOP ( 'NONE', ( #5329, #7799, #7517, #2611 ) ) ;
#1979=( BOUNDED_CURVE ( )  B_SPLINE_CURVE ( 2, ( #12632, #2652, #1568, #10468, #3987, #15526, #12877, #3908, #6661, #6328, #9059, #2727, #2482 ),
 .UNSPECIFIED., .F., .T. ) 
 B_SPLINE_CURVE_WITH_KNOTS ( ( 3, 2, 2, 2, 2, 2, 3 ),
 ( 0.6833333333333333481, 0.6866666666666666474, 0.6933333333333333570, 0.6999999999999999556, 0.7066666666666666652, 0.7133333333333333748, 0.7166666666666666741 ),
 .UNSPECIFIED. ) 
 CURVE ( )  GEOMETRIC_REPRESENTATION_ITEM ( )  RATIONAL_B_SPLINE_CURVE ( ( 0.9755282581475768211, 0.9755282581475768211, 1.000000000000000000, 0.9510565162951535312, 1.000000000000000000, 0.9510565162951535312, 1.000000000000000000, 0.9510565162951535312, 1.000000000000000000, 0.9510565162951535312, 1.000000000000000000, 0.9755282581475768211, 0.9755282581475768211 ) ) 
 REPRESENTATION_ITEM ( '' )  );
#1980=CARTESIAN_POINT ( 'NONE',  ( 40.45084971874737789, 44.58125000068280031, 29.38926261462365375 ) ) ;
#1987=CARTESIAN_POINT ( 'NONE',  ( 7.919222016226693306, 34.55125428154684641, 50.00000000000003553 ) ) ;
#1993=CARTESIAN_POINT ( 'NONE',  ( 0.000000000000000000, 25.00000000000000000, -47.00000000000000000 ) ) ;
#1997=CARTESIAN_POINT ( 'NONE',  ( -50.00000000000000000, 28.00000000000000000, 0.000000000000000000 ) ) ;
#1999=CARTESIAN_POINT ( 'NONE',  ( 0.000000000000000000, 252.0000000000000000, 82.49773270518484480 ) ) ;
#2007=CARTESIAN_POINT ( 'NONE',  ( -49.86468353124999453, 33.75937500034140015, -16.20201782572375393 ) ) ;
#2016=CIRCLE ( 'NONE', #8120, 79.49773270518484480 ) ;
#2018=CARTESIAN_POINT ( 'NONE',  ( -15.40903463028480580, 30.32187500034140015, 47.42413220539094709 ) ) ;
#2020=CARTESIAN_POINT ( 'NONE',  ( 9.041411772857449839E-15, 53.82568851450475478, -65.15972704814865324 ) ) ;
#2022=CARTESIAN_POINT ( 'NONE',  ( -30.81806926056963292, 39.62187500034138310, -42.41743335407647209 ) ) ;
#2026=CARTESIAN_POINT ( 'NONE',  ( -40.34137639590981905, 41.65937500034139873, -29.30972558990011478 ) ) ;
#2030=CARTESIAN_POINT ( 'NONE',  ( -49.99999999999999289, 33.88125000068280457, 16.24598481164533226 ) ) ;
#2034=CARTESIAN_POINT ( 'NONE',  ( 30.81806926056962936, 43.22187500034139873, -42.41743335407646498 ) ) ;
#2038=CARTESIAN_POINT ( 'NONE',  ( 15.40903463028482356, 24.52187500034139589, 47.42413220539093999 ) ) ;
#2045=CARTESIAN_POINT ( 'NONE',  ( 49.86468353124999453, 39.02187500034138878, -16.20201782572376459 ) ) ;
#2065=CARTESIAN_POINT ( 'NONE',  ( 30.81806926056962936, 29.15937500034139518, -42.41743335407647209 ) ) ;
#2070=CARTESIAN_POINT ( 'NONE',  ( -15.45084971874736368, 44.18125000068280173, 47.55282581475768211 ) ) ;
#2078=CARTESIAN_POINT ( 'NONE',  ( -2.445080149700054274E-14, 46.28125000068280315, 50.00000000000000000 ) ) ;
#2084=CARTESIAN_POINT ( 'NONE',  ( -3.219174618344376363E-15, 29.49999999999999645, -52.57311121191334990 ) ) ;
#2086=CARTESIAN_POINT ( 'NONE',  ( 49.86468353125001585, 48.75937500034140015, 16.20201782572375038 ) ) ;
#2089=CARTESIAN_POINT ( 'NONE',  ( -49.86468353124999453, 25.95937500034139589, 16.20201782572377169 ) ) ;
#2092=CARTESIAN_POINT ( 'NONE',  ( 9.631387414534489405E-15, 38.35937500034139447, 52.43083105670540789 ) ) ;
#2095=CARTESIAN_POINT ( 'NONE',  ( 49.99999999999999289, 44.88125000068279036, -16.24598481164532160 ) ) ;
#2100=CARTESIAN_POINT ( 'NONE',  ( -49.86468353124999453, 27.82187500034139305, -16.20201782572375393 ) ) ;
#2103=CARTESIAN_POINT ( 'NONE',  ( 49.86468353124999453, 41.02187500034139589, -16.20201782572376459 ) ) ;
#2106=VECTOR ( 'NONE', #5726, 1000.000000000000000 ) ;
#2107=CARTESIAN_POINT ( 'NONE',  ( -40.34137639590981195, 42.05937500034139731, 29.30972558990012189 ) ) ;
#2108=ORIENTED_EDGE ( 'NONE', *, *, #9058, .T. ) ;
#2109=CARTESIAN_POINT ( 'NONE',  ( -15.45084971874736368, 26.18125000068280173, 47.55282581475768211 ) ) ;
#2112=CARTESIAN_POINT ( 'NONE',  ( -49.86468353125000164, 43.92187500034140157, 0.000000000000000000 ) ) ;
#2115=CARTESIAN_POINT ( 'NONE',  ( -30.81806926056962226, 26.22187500034139518, 42.41743335407647919 ) ) ;
#2118=LINE ( 'NONE', #14917, #5932 ) ;
#2120=CARTESIAN_POINT ( 'NONE',  ( -49.86468353125000164, 41.92187500034139447, 0.000000000000000000 ) ) ;
#2121=CARTESIAN_POINT ( 'NONE',  ( -50.00000000000000000, 43.78125000068280315, 0.000000000000000000 ) ) ;
#2123=ORIENTED_EDGE ( 'NONE', *, *, #4267, .F. ) ;
#2124=( BOUNDED_SURFACE ( )  B_SPLINE_SURFACE ( 1, 2, ( 
 ( #4522, #9507, #5766, #2247, #15897, #14709, #8327, #756, #10910, #7257, #15974, #2086, #8413, #11083, #13638, #13480, #12237, #14632, #7341, #839, #10993, #10748, #584, #15806, #3179, #3256, #13391, #11246, #5101, #11478, #7660, #12563, #10155, #3594, #16304, #1327, #12410, #1082, #4940, #8653, #16392, #13964, #13725, #12731, #5181, #5025, #4857, #6419, #15295, #76, #14048, #10235, #15130, #9914, #3920, #9994, #8991, #2665, #2587, #7420, #2339, #12489, #6100, #3683, #6254, #1000, #13804, #8737, #6173, #11170, #7493, #14968, #2496, #15055, #16225, #10078, #7573, #2415, #418, #1160, #11324, #3757, #8816, #13881, #12650, #1248, #6341, #11405, #15206, #3837, #8902, #6595, #9398, #10651, #14126, #6501, #6839, #2832, #9073, #403, #324, #5350, #8061, #11649, #7739, #244, #6675, #12979, #7818, #11557, #12806, #5511, #11804, #14207, #13057, #10404, #1408, #9242, #15460, #163, #9321, #4331, #2742, #2917, #10482, #11890, #488, #4078, #13134, #1582, #1659, #5271, #15629, #1741, #14294, #10321, #5424, #15704, #9152, #12891, #7902, #6758, #2992, #15380, #11724, #15542, #4172, #7983, #14372, #10574, #4254, #1500, #4001, #5588, #14446, #3071, #13538, #5822, #15876, #12042, #10813, #8387, #5905, #2143, #4498, #9636, #8306, #10723, #9810, #3408, #10888, #5739, #7231, #816, #11056, #10966, #14689, #16031, #6914, #12289, #13372, #563, #643, #892, #14532, #12215, #5988, #9728, #4659, #11967, #15951, #14776, #8472, #16124, #4754, #9563, #8151, #3316, #1820, #9483, #13218, #5658, #13458, #1975, #13294, #15785, #14609, #2065, #4410, #3154, #8228, #1894, #7155, #6986, #3233, #7068, #12131, #737, #4573, #15186, #1135, #6319, #13939, #8714, #16449, #8625, #8545, #10055, #1059, #6078, #9969, #3658, #3490, #11300, #7641, #5081, #13779, #13697, #4832, #3570, #4915, #2313, #2221, #7398, #54, #16203, #7473, #6151, #15027, #2392, #13859, #16279, #16362, #12540, #10134, #3815, #6229, #5000, #12467, #5158, #15109, #3734, #13615, #8795, #7316, #11458, #11221, #2474, #7552, #12624, #2562, #8880, #1224, #11384, #11145, #12707, #1306, #14861, #6397, #12381, #9889, #978, #14943, #1388, #5484, #2971, #14187, #2642, #15610, #13112, #4232, #11867, #10554, #12956, #7716, #14354, #7798, #1718, #6817, #11780, #5250 ),
 ( #3900, #380, #468, #10302, #5402, #1560, #8041, #10215, #12868, #9301, #15438, #15516, #15267, #1638, #8969, #303, #14027, #7879, #12785, #14104, #11534, #10382, #4147, #6477, #135, #2805, #4057, #11628, #9127, #15359, #13035, #6654, #3978, #9050, #7962, #10460, #2719, #1474, #11704, #6570, #225, #5331, #9219, #6733, #14272, #2896, #12109, #10793, #13199, #12270, #5884, #8285, #8208, #9702, #3296, #5719, #14667, #1803, #4390, #10946, #5572, #10704, #14512, #6895, #9543, #7134, #11948, #795, #14757, #14588, #14427, #16011, #8452, #4637, #7209, #3386, #13354, #3047, #13516, #3136, #2120, #10632, #12193, #546, #5638, #15763, #15684, #13276, #15855, #4311, #6971, #1876, #9458, #9377, #623, #8124, #715, #12024, #4477, #3214, #5799, #1954, #9618, #7046, #10869, #15933, #4555, #8365, #13437, #2045, #13594, #13840, #7380, #8602, #1198, #957, #6299, #7535, #2201, #11031, #3719, #13676, #8526, #7457, #1038, #16186, #10039, #6055, #873, #11126, #12446, #2291, #12353, #16102, #6134, #3469, #15003, #15091, #7297, #3550, #9792, #4815, #4980, #14839, #11205, #9868, #14919, #9948, #16257, #4891, #3641, #8695, #13761, #4735, #2374, #5968, #8779, #12524, #1116, #6212, #11282, #16340, #2454, #12604, #9597, #5944, #852, #5780, #10846, #14567, #6029, #12169, #15910, #9431, #8342, #14481, #12329, #9520, #4534, #3191, #8429, #14815, #11007, #931, #14644, #8186, #5860, #598, #3114, #3272, #10924, #3446, #3358, #16069, #13328, #13403, #2018, #15735, #15986, #5693, #10761, #13573, #7113, #770, #4366, #8264, #13252, #2177, #15823, #1852, #8508, #4612, #4455, #13492, #9675, #1930, #4704, #7023, #6948, #12077, #14725, #2100, #683, #12002, #7188, #12249, #9768, #7273, #9022, #6450, #5134, #7520, #6621, #194, #2615, #2529, #4029, #14077, #7848, #7768, #11509, #12838, #3711, #15412, #10187, #13830, #8850, #9099, #11357, #2692, #14158, #6531, #1443, #8768, #12761, #11596, #5300, #10349, #2774, #7609, #12928, #106, #15082, #6287, #1531, #2443, #5212, #15241, #10108, #12593, #1280, #15329, #16331, #10030, #4970, #1188, #3948, #16422, #5058, #15160, #3786, #13910, #12684, #6370, #7691, #11436, #28, #3866, #8939, #13998, #1360, #10272, #14326, #2864, #6787, #440, #273, #8091, #4449, #1847, #5543 ) ),
 .UNSPECIFIED., .F., .F., .F. ) 
 B_SPLINE_SURFACE_WITH_KNOTS ( ( 2, 2 ),
 ( 3, 2, 2, 2, 2, 2, 2, 2, 2, 2, 2, 2, 2, 2, 2, 2, 2, 2, 2, 2, 2, 2, 2, 2, 2, 2, 2, 2, 2, 2, 2, 2, 2, 2, 2, 2, 2, 2, 2, 2, 2, 2, 2, 2, 2, 2, 2, 2, 2, 2, 2, 2, 2, 2, 2, 2, 2, 2, 2, 2, 2, 2, 2, 2, 2, 2, 2, 2, 2, 2, 2, 2, 2, 2, 2, 2, 2, 2, 2, 2, 2, 2, 2, 2, 2, 2, 2, 2, 2, 2, 2, 2, 2, 2, 2, 2, 2, 2, 2, 2, 2, 2, 2, 2, 2, 2, 2, 2, 2, 2, 2, 2, 2, 2, 2, 2, 2, 2, 2, 2, 2, 2, 2, 2, 2, 2, 2, 2, 2, 2, 2, 2, 2, 2, 2, 2, 2, 2, 2, 2, 2, 2, 2, 2, 2, 2, 2, 2, 2, 2, 3 ),
 ( 0.000000000000000000, 1.000000000000000000 ),
 ( 0.000000000000000000, 0.006666666666666667095, 0.01333333333333333419, 0.02000000000000000042, 0.02666666666666666838, 0.03333333333333333287, 0.04000000000000000083, 0.04666666666666666879, 0.05333333333333333676, 0.05999999999999999778, 0.06666666666666666574, 0.07333333333333333370, 0.08000000000000000167, 0.08666666666666666963, 0.09333333333333333759, 0.1000000000000000056, 0.1066666666666666735, 0.1133333333333333276, 0.1199999999999999956, 0.1266666666666666774, 0.1333333333333333315, 0.1400000000000000133, 0.1466666666666666674, 0.1533333333333333215, 0.1600000000000000033, 0.1666666666666666574, 0.1733333333333333393, 0.1799999999999999933, 0.1866666666666666752, 0.1933333333333333293, 0.2000000000000000111, 0.2066666666666666652, 0.2133333333333333470, 0.2200000000000000011, 0.2266666666666666552, 0.2333333333333333370, 0.2399999999999999911, 0.2466666666666666730, 0.2533333333333333548, 0.2600000000000000089, 0.2666666666666666630, 0.2733333333333333171, 0.2800000000000000266, 0.2866666666666666807, 0.2933333333333333348, 0.2999999999999999889, 0.3066666666666666430, 0.3133333333333333526, 0.3200000000000000067, 0.3266666666666666607, 0.3333333333333333148, 0.3400000000000000244, 0.3466666666666666785, 0.3533333333333333326, 0.3599999999999999867, 0.3666666666666666408, 0.3733333333333333504, 0.3800000000000000044, 0.3866666666666666585, 0.3933333333333333126, 0.4000000000000000222, 0.4066666666666666763, 0.4133333333333333304, 0.4199999999999999845, 0.4266666666666666941, 0.4333333333333333481, 0.4400000000000000022, 0.4466666666666666563, 0.4533333333333333104, 0.4600000000000000200, 0.4666666666666666741, 0.4733333333333333282, 0.4799999999999999822, 0.4866666666666666918, 0.4933333333333333459, 0.5000000000000000000, 0.5066666666666667096, 0.5133333333333333082, 0.5200000000000000178, 0.5266666666666666163, 0.5333333333333333259, 0.5400000000000000355, 0.5466666666666666341, 0.5533333333333333437, 0.5600000000000000533, 0.5666666666666666519, 0.5733333333333333615, 0.5799999999999999600, 0.5866666666666666696, 0.5933333333333333792, 0.5999999999999999778, 0.6066666666666666874, 0.6133333333333332860, 0.6199999999999999956, 0.6266666666666667052, 0.6333333333333333037, 0.6400000000000000133, 0.6466666666666666119, 0.6533333333333333215, 0.6600000000000000311, 0.6666666666666666297, 0.6733333333333333393, 0.6800000000000000488, 0.6866666666666666474, 0.6933333333333333570, 0.6999999999999999556, 0.7066666666666666652, 0.7133333333333333748, 0.7199999999999999734, 0.7266666666666666829, 0.7333333333333332815, 0.7399999999999999911, 0.7466666666666667007, 0.7533333333333332993, 0.7600000000000000089, 0.7666666666666667185, 0.7733333333333333171, 0.7800000000000000266, 0.7866666666666666252, 0.7933333333333333348, 0.8000000000000000444, 0.8066666666666666430, 0.8133333333333333526, 0.8199999999999999512, 0.8266666666666666607, 0.8333333333333333703, 0.8399999999999999689, 0.8466666666666666785, 0.8533333333333333881, 0.8599999999999999867, 0.8666666666666666963, 0.8733333333333332948, 0.8800000000000000044, 0.8866666666666667140, 0.8933333333333333126, 0.9000000000000000222, 0.9066666666666666208, 0.9133333333333333304, 0.9200000000000000400, 0.9266666666666666385, 0.9333333333333333481, 0.9399999999999999467, 0.9466666666666666563, 0.9533333333333333659, 0.9599999999999999645, 0.9666666666666666741, 0.9733333333333333837, 0.9799999999999999822, 0.9866666666666666918, 0.9933333333333332904, 1.000000000000000000 ),
 .UNSPECIFIED. ) 
 GEOMETRIC_REPRESENTATION_ITEM ( )  RATIONAL_B_SPLINE_SURFACE ( (
 ( 1.000000000000000000, 0.9510565162951535312, 1.000000000000000000, 0.9510565162951535312, 1.000000000000000000, 0.9510565162951535312, 1.000000000000000000, 0.9510565162951535312, 1.000000000000000000, 0.9510565162951535312, 1.000000000000000000, 0.9510565162951535312, 1.000000000000000000, 0.9510565162951535312, 1.000000000000000000, 0.9510565162951535312, 1.000000000000000000, 0.9510565162951535312, 1.000000000000000000, 0.9510565162951535312, 1.000000000000000000, 0.9510565162951535312, 1.000000000000000000, 0.9510565162951535312, 1.000000000000000000, 0.9510565162951535312, 1.000000000000000000, 0.9510565162951535312, 1.000000000000000000, 0.9510565162951535312, 1.000000000000000000, 0.9510565162951535312, 1.000000000000000000, 0.9510565162951535312, 1.000000000000000000, 0.9510565162951535312, 1.000000000000000000, 0.9510565162951535312, 1.000000000000000000, 0.9510565162951535312, 1.000000000000000000, 0.9510565162951535312, 1.000000000000000000, 0.9510565162951535312, 1.000000000000000000, 0.9510565162951535312, 1.000000000000000000, 0.9510565162951535312, 1.000000000000000000, 0.9510565162951535312, 1.000000000000000000, 0.9510565162951535312, 1.000000000000000000, 0.9510565162951535312, 1.000000000000000000, 0.9510565162951535312, 1.000000000000000000, 0.9510565162951535312, 1.000000000000000000, 0.9510565162951535312, 1.000000000000000000, 0.9510565162951535312, 1.000000000000000000, 0.9510565162951535312, 1.000000000000000000, 0.9510565162951535312, 1.000000000000000000, 0.9510565162951535312, 1.000000000000000000, 0.9510565162951535312, 1.000000000000000000, 0.9510565162951535312, 1.000000000000000000, 0.9510565162951535312, 1.000000000000000000, 0.9510565162951535312, 1.000000000000000000, 0.9510565162951535312, 1.000000000000000000, 0.9510565162951535312, 1.000000000000000000, 0.9510565162951535312, 1.000000000000000000, 0.9510565162951535312, 1.000000000000000000, 0.9510565162951535312, 1.000000000000000000, 0.9510565162951535312, 1.000000000000000000, 0.9510565162951535312, 1.000000000000000000, 0.9510565162951535312, 1.000000000000000000, 0.9510565162951535312, 1.000000000000000000, 0.9510565162951535312, 1.000000000000000000, 0.9510565162951535312, 1.000000000000000000, 0.9510565162951535312, 1.000000000000000000, 0.9510565162951535312, 1.000000000000000000, 0.9510565162951535312, 1.000000000000000000, 0.9510565162951535312, 1.000000000000000000, 0.9510565162951535312, 1.000000000000000000, 0.9510565162951535312, 1.000000000000000000, 0.9510565162951535312, 1.000000000000000000, 0.9510565162951535312, 1.000000000000000000, 0.9510565162951535312, 1.000000000000000000, 0.9510565162951535312, 1.000000000000000000, 0.9510565162951535312, 1.000000000000000000, 0.9510565162951535312, 1.000000000000000000, 0.9510565162951535312, 1.000000000000000000, 0.9510565162951535312, 1.000000000000000000, 0.9510565162951535312, 1.000000000000000000, 0.9510565162951535312, 1.000000000000000000, 0.9510565162951535312, 1.000000000000000000, 0.9510565162951535312, 1.000000000000000000, 0.9510565162951535312, 1.000000000000000000, 0.9510565162951535312, 1.000000000000000000, 0.9510565162951535312, 1.000000000000000000, 0.9510565162951535312, 1.000000000000000000, 0.9510565162951535312, 1.000000000000000000, 0.9510565162951535312, 1.000000000000000000, 0.9510565162951535312, 1.000000000000000000, 0.9510565162951535312, 1.000000000000000000, 0.9510565162951535312, 1.000000000000000000, 0.9510565162951535312, 1.000000000000000000, 0.9510565162951535312, 1.000000000000000000, 0.9510565162951535312, 1.000000000000000000, 0.9510565162951535312, 1.000000000000000000, 0.9510565162951535312, 1.000000000000000000, 0.9510565162951535312, 1.000000000000000000, 0.9510565162951535312, 1.000000000000000000, 0.9510565162951535312, 1.000000000000000000, 0.9510565162951535312, 1.000000000000000000, 0.9510565162951535312, 1.000000000000000000, 0.9510565162951535312, 1.000000000000000000, 0.9510565162951535312, 1.000000000000000000, 0.9510565162951535312, 1.000000000000000000, 0.9510565162951535312, 1.000000000000000000, 0.9510565162951535312, 1.000000000000000000, 0.9510565162951535312, 1.000000000000000000, 0.9510565162951535312, 1.000000000000000000, 0.9510565162951535312, 1.000000000000000000, 0.9510565162951535312, 1.000000000000000000, 0.9510565162951535312, 1.000000000000000000, 0.9510565162951535312, 1.000000000000000000, 0.9510565162951535312, 1.000000000000000000, 0.9510565162951535312, 1.000000000000000000, 0.9510565162951535312, 1.000000000000000000, 0.9510565162951535312, 1.000000000000000000, 0.9510565162951535312, 1.000000000000000000, 0.9510565162951535312, 1.000000000000000000, 0.9510565162951535312, 1.000000000000000000, 0.9510565162951535312, 1.000000000000000000, 0.9510565162951535312, 1.000000000000000000, 0.9510565162951535312, 1.000000000000000000, 0.9510565162951535312, 1.000000000000000000, 0.9510565162951535312, 1.000000000000000000, 0.9510565162951535312, 1.000000000000000000, 0.9510565162951535312, 1.000000000000000000, 0.9510565162951535312, 1.000000000000000000, 0.9510565162951535312, 1.000000000000000000, 0.9510565162951535312, 1.000000000000000000, 0.9510565162951535312, 1.000000000000000000, 0.9510565162951535312, 1.000000000000000000, 0.9510565162951535312, 1.000000000000000000, 0.9510565162951535312, 1.000000000000000000, 0.9510565162951535312, 1.000000000000000000, 0.9510565162951535312, 1.000000000000000000, 0.9510565162951535312, 1.000000000000000000, 0.9510565162951535312, 1.000000000000000000, 0.9510565162951535312, 1.000000000000000000, 0.9510565162951535312, 1.000000000000000000, 0.9510565162951535312, 1.000000000000000000, 0.9510565162951535312, 1.000000000000000000, 0.9510565162951535312, 1.000000000000000000, 0.9510565162951535312, 1.000000000000000000, 0.9510565162951535312, 1.000000000000000000, 0.9510565162951535312, 1.000000000000000000, 0.9510565162951535312, 1.000000000000000000, 0.9510565162951535312, 1.000000000000000000, 0.9510565162951535312, 1.000000000000000000, 0.9510565162951535312, 1.000000000000000000, 0.9510565162951535312, 1.000000000000000000, 0.9510565162951535312, 1.000000000000000000, 0.9510565162951535312, 1.000000000000000000, 0.9510565162951535312, 1.000000000000000000, 0.9510565162951535312, 1.000000000000000000, 0.9510565162951535312, 1.000000000000000000, 0.9510565162951535312, 1.000000000000000000, 0.9510565162951535312, 1.000000000000000000, 0.9510565162951535312, 1.000000000000000000, 0.9510565162951535312, 1.000000000000000000, 0.9510565162951535312, 1.000000000000000000, 0.9510565162951535312, 1.000000000000000000, 0.9510565162951535312, 1.000000000000000000, 0.9510565162951535312, 1.000000000000000000, 0.9510565162951535312, 1.000000000000000000, 0.9510565162951535312, 1.000000000000000000),
 ( 1.000000000000000000, 0.9510565162951535312, 1.000000000000000000, 0.9510565162951535312, 1.000000000000000000, 0.9510565162951535312, 1.000000000000000000, 0.9510565162951535312, 1.000000000000000000, 0.9510565162951535312, 1.000000000000000000, 0.9510565162951535312, 1.000000000000000000, 0.9510565162951535312, 1.000000000000000000, 0.9510565162951535312, 1.000000000000000000, 0.9510565162951535312, 1.000000000000000000, 0.9510565162951535312, 1.000000000000000000, 0.9510565162951535312, 1.000000000000000000, 0.9510565162951535312, 1.000000000000000000, 0.9510565162951535312, 1.000000000000000000, 0.9510565162951535312, 1.000000000000000000, 0.9510565162951535312, 1.000000000000000000, 0.9510565162951535312, 1.000000000000000000, 0.9510565162951535312, 1.000000000000000000, 0.9510565162951535312, 1.000000000000000000, 0.9510565162951535312, 1.000000000000000000, 0.9510565162951535312, 1.000000000000000000, 0.9510565162951535312, 1.000000000000000000, 0.9510565162951535312, 1.000000000000000000, 0.9510565162951535312, 1.000000000000000000, 0.9510565162951535312, 1.000000000000000000, 0.9510565162951535312, 1.000000000000000000, 0.9510565162951535312, 1.000000000000000000, 0.9510565162951535312, 1.000000000000000000, 0.9510565162951535312, 1.000000000000000000, 0.9510565162951535312, 1.000000000000000000, 0.9510565162951535312, 1.000000000000000000, 0.9510565162951535312, 1.000000000000000000, 0.9510565162951535312, 1.000000000000000000, 0.9510565162951535312, 1.000000000000000000, 0.9510565162951535312, 1.000000000000000000, 0.9510565162951535312, 1.000000000000000000, 0.9510565162951535312, 1.000000000000000000, 0.9510565162951535312, 1.000000000000000000, 0.9510565162951535312, 1.000000000000000000, 0.9510565162951535312, 1.000000000000000000, 0.9510565162951535312, 1.000000000000000000, 0.9510565162951535312, 1.000000000000000000, 0.9510565162951535312, 1.000000000000000000, 0.9510565162951535312, 1.000000000000000000, 0.9510565162951535312, 1.000000000000000000, 0.9510565162951535312, 1.000000000000000000, 0.9510565162951535312, 1.000000000000000000, 0.9510565162951535312, 1.000000000000000000, 0.9510565162951535312, 1.000000000000000000, 0.9510565162951535312, 1.000000000000000000, 0.9510565162951535312, 1.000000000000000000, 0.9510565162951535312, 1.000000000000000000, 0.9510565162951535312, 1.000000000000000000, 0.9510565162951535312, 1.000000000000000000, 0.9510565162951535312, 1.000000000000000000, 0.9510565162951535312, 1.000000000000000000, 0.9510565162951535312, 1.000000000000000000, 0.9510565162951535312, 1.000000000000000000, 0.9510565162951535312, 1.000000000000000000, 0.9510565162951535312, 1.000000000000000000, 0.9510565162951535312, 1.000000000000000000, 0.9510565162951535312, 1.000000000000000000, 0.9510565162951535312, 1.000000000000000000, 0.9510565162951535312, 1.000000000000000000, 0.9510565162951535312, 1.000000000000000000, 0.9510565162951535312, 1.000000000000000000, 0.9510565162951535312, 1.000000000000000000, 0.9510565162951535312, 1.000000000000000000, 0.9510565162951535312, 1.000000000000000000, 0.9510565162951535312, 1.000000000000000000, 0.9510565162951535312, 1.000000000000000000, 0.9510565162951535312, 1.000000000000000000, 0.9510565162951535312, 1.000000000000000000, 0.9510565162951535312, 1.000000000000000000, 0.9510565162951535312, 1.000000000000000000, 0.9510565162951535312, 1.000000000000000000, 0.9510565162951535312, 1.000000000000000000, 0.9510565162951535312, 1.000000000000000000, 0.9510565162951535312, 1.000000000000000000, 0.9510565162951535312, 1.000000000000000000, 0.9510565162951535312, 1.000000000000000000, 0.9510565162951535312, 1.000000000000000000, 0.9510565162951535312, 1.000000000000000000, 0.9510565162951535312, 1.000000000000000000, 0.9510565162951535312, 1.000000000000000000, 0.9510565162951535312, 1.000000000000000000, 0.9510565162951535312, 1.000000000000000000, 0.9510565162951535312, 1.000000000000000000, 0.9510565162951535312, 1.000000000000000000, 0.9510565162951535312, 1.000000000000000000, 0.9510565162951535312, 1.000000000000000000, 0.9510565162951535312, 1.000000000000000000, 0.9510565162951535312, 1.000000000000000000, 0.9510565162951535312, 1.000000000000000000, 0.9510565162951535312, 1.000000000000000000, 0.9510565162951535312, 1.000000000000000000, 0.9510565162951535312, 1.000000000000000000, 0.9510565162951535312, 1.000000000000000000, 0.9510565162951535312, 1.000000000000000000, 0.9510565162951535312, 1.000000000000000000, 0.9510565162951535312, 1.000000000000000000, 0.9510565162951535312, 1.000000000000000000, 0.9510565162951535312, 1.000000000000000000, 0.9510565162951535312, 1.000000000000000000, 0.9510565162951535312, 1.000000000000000000, 0.9510565162951535312, 1.000000000000000000, 0.9510565162951535312, 1.000000000000000000, 0.9510565162951535312, 1.000000000000000000, 0.9510565162951535312, 1.000000000000000000, 0.9510565162951535312, 1.000000000000000000, 0.9510565162951535312, 1.000000000000000000, 0.9510565162951535312, 1.000000000000000000, 0.9510565162951535312, 1.000000000000000000, 0.9510565162951535312, 1.000000000000000000, 0.9510565162951535312, 1.000000000000000000, 0.9510565162951535312, 1.000000000000000000, 0.9510565162951535312, 1.000000000000000000, 0.9510565162951535312, 1.000000000000000000, 0.9510565162951535312, 1.000000000000000000, 0.9510565162951535312, 1.000000000000000000, 0.9510565162951535312, 1.000000000000000000, 0.9510565162951535312, 1.000000000000000000, 0.9510565162951535312, 1.000000000000000000, 0.9510565162951535312, 1.000000000000000000, 0.9510565162951535312, 1.000000000000000000, 0.9510565162951535312, 1.000000000000000000, 0.9510565162951535312, 1.000000000000000000, 0.9510565162951535312, 1.000000000000000000, 0.9510565162951535312, 1.000000000000000000, 0.9510565162951535312, 1.000000000000000000, 0.9510565162951535312, 1.000000000000000000, 0.9510565162951535312, 1.000000000000000000, 0.9510565162951535312, 1.000000000000000000, 0.9510565162951535312, 1.000000000000000000, 0.9510565162951535312, 1.000000000000000000, 0.9510565162951535312, 1.000000000000000000, 0.9510565162951535312, 1.000000000000000000, 0.9510565162951535312, 1.000000000000000000, 0.9510565162951535312, 1.000000000000000000, 0.9510565162951535312, 1.000000000000000000, 0.9510565162951535312, 1.000000000000000000, 0.9510565162951535312, 1.000000000000000000, 0.9510565162951535312, 1.000000000000000000, 0.9510565162951535312, 1.000000000000000000, 0.9510565162951535312, 1.000000000000000000, 0.9510565162951535312, 1.000000000000000000, 0.9510565162951535312, 1.000000000000000000, 0.9510565162951535312, 1.000000000000000000, 0.9510565162951535312, 1.000000000000000000, 0.9510565162951535312, 1.000000000000000000, 0.9510565162951535312, 1.000000000000000000) ) ) 
 REPRESENTATION_ITEM ( '' )  SURFACE ( )  );
#2128=CARTESIAN_POINT ( 'NONE',  ( 2.600676159226421000E-13, 33.49999999999999289, -49.99999999999999289 ) ) ;
#2129=CARTESIAN_POINT ( 'NONE',  ( -30.90169943749474513, 49.70000000000000284, -42.53254041760200721 ) ) ;
#2139=EDGE_CURVE ( 'NONE', #13613, #10886, #15084, .T. ) ;
#2141=CARTESIAN_POINT ( 'NONE',  ( -3.111920190527341144E-15, 25.28125000068279604, -50.00000000000000000 ) ) ;
#2142=ORIENTED_EDGE ( 'NONE', *, *, #4336, .F. ) ;
#2143=CARTESIAN_POINT ( 'NONE',  ( -30.81806926056963292, 33.55937500034138310, -42.41743335407647209 ) ) ;
#2145=ORIENTED_EDGE ( 'NONE', *, *, #8837, .T. ) ;
#2147=CARTESIAN_POINT ( 'NONE',  ( 15.45084971874737789, 46.38125000068279746, 47.55282581475767500 ) ) ;
#2151=DIRECTION ( 'NONE',  ( 0.000000000000000000, 1.000000000000000000, 0.000000000000000000 ) ) ;
#2156=FACE_OUTER_BOUND ( 'NONE', #8589, .T. ) ;
#2157=CYLINDRICAL_SURFACE ( 'NONE', #10270, 50.00000000000000000 ) ;
#2158=CARTESIAN_POINT ( 'NONE',  ( 0.000000000000000000, 0.000000000000000000, 0.000000000000000000 ) ) ;
#2162=CARTESIAN_POINT ( 'NONE',  ( -15.45084971874736368, 28.40000000000000213, 47.55282581475768211 ) ) ;
#2165=ORIENTED_EDGE ( 'NONE', *, *, #6538, .F. ) ;
#2170=CARTESIAN_POINT ( 'NONE',  ( 15.40903463028482356, 34.45937500034139589, 47.42413220539093999 ) ) ;
#2177=CARTESIAN_POINT ( 'NONE',  ( 30.81806926056962936, 29.22187500034139873, -42.41743335407647209 ) ) ;
#2180=CARTESIAN_POINT ( 'NONE',  ( 40.34137639590981905, 36.72187500034139163, 29.30972558990010768 ) ) ;
#2185=CARTESIAN_POINT ( 'NONE',  ( -49.86468353124999453, 43.75937500034140015, -16.20201782572375393 ) ) ;
#2187=CARTESIAN_POINT ( 'NONE',  ( -15.45084971874737256, 23.38125000068280102, -47.55282581475767500 ) ) ;
#2191=CARTESIAN_POINT ( 'NONE',  ( -15.40903463028480580, 36.32187500034140015, 47.42413220539094709 ) ) ;
#2194=CARTESIAN_POINT ( 'NONE',  ( 15.40903463028481113, 25.32187500034139660, -47.42413220539094709 ) ) ;
#2201=CARTESIAN_POINT ( 'NONE',  ( -40.34137639590981195, 38.12187500034139731, 29.30972558990012189 ) ) ;
#2202=CARTESIAN_POINT ( 'NONE',  ( -15.45084971874737256, 31.38125000068280102, -47.55282581475767500 ) ) ;
#2217=CARTESIAN_POINT ( 'NONE',  ( -3.111920190527341144E-15, 43.28125000068280315, -50.00000000000000000 ) ) ;
#2218=DIRECTION ( 'NONE',  ( 0.000000000000000000, -1.000000000000000000, 0.000000000000000000 ) ) ;
#2219=ORIENTED_EDGE ( 'NONE', *, *, #7014, .F. ) ;
#2221=CARTESIAN_POINT ( 'NONE',  ( -40.34137639590981905, 25.65937500034139518, -29.30972558990011478 ) ) ;
#2228=CARTESIAN_POINT ( 'NONE',  ( 40.45084971874737079, 40.98125000068279888, -29.38926261462366440 ) ) ;
#2230=CARTESIAN_POINT ( 'NONE',  ( 6.123233995736766085E-15, 193.4213562373095385, 50.00000000000000000 ) ) ;
#2231=ORIENTED_EDGE ( 'NONE', *, *, #7880, .T. ) ;
#2233=CARTESIAN_POINT ( 'NONE',  ( -15.45084971874736368, 28.18125000068279817, 47.55282581475768211 ) ) ;
#2243=DIRECTION ( 'NONE',  ( 0.000000000000000000, 0.000000000000000000, -1.000000000000000000 ) ) ;
#2246=CARTESIAN_POINT ( 'NONE',  ( 50.00000000000000711, 26.89999999999999503, 16.24598481164530739 ) ) ;
#2247=CARTESIAN_POINT ( 'NONE',  ( -30.81806926056963292, 49.55937500034139731, -42.41743335407647209 ) ) ;
#2248=ORIENTED_EDGE ( 'NONE', *, *, #9105, .T. ) ;
#2252=CARTESIAN_POINT ( 'NONE',  ( -49.86468353125000164, 37.85937500034139447, 0.000000000000000000 ) ) ;
#2255=CARTESIAN_POINT ( 'NONE',  ( 15.45084971874737789, 40.38125000068280457, 47.55282581475767500 ) ) ;
#2257=CARTESIAN_POINT ( 'NONE',  ( 2.600676159226421000E-13, 31.28125000068279604, -49.99999999999999289 ) ) ;
#2258=CARTESIAN_POINT ( 'NONE',  ( 50.00000000000000711, 44.68125000068278752, 16.24598481164530739 ) ) ;
#2266=CARTESIAN_POINT ( 'NONE',  ( -15.40903463028481646, 35.52187500034139589, -47.42413220539093999 ) ) ;
#2272=CARTESIAN_POINT ( 'NONE',  ( 49.86468353124999453, 40.95937500034140299, -16.20201782572376104 ) ) ;
#2275=CARTESIAN_POINT ( 'NONE',  ( -50.00000000000000000, 23.78125000068279959, 0.000000000000000000 ) ) ;
#2278=AXIS2_PLACEMENT_3D ( 'NONE', #11213, #11289, #3478 ) ;
#2283=CARTESIAN_POINT ( 'NONE',  ( 50.00000000000000711, 30.89999999999999858, 16.24598481164530739 ) ) ;
#2284=CARTESIAN_POINT ( 'NONE',  ( 49.86468353124999453, 23.02187500034139944, -16.20201782572376459 ) ) ;
#2291=CARTESIAN_POINT ( 'NONE',  ( 49.86468353125001585, 36.82187500034140015, 16.20201782572375038 ) ) ;
#2294=ORIENTED_EDGE ( 'NONE', *, *, #3693, .F. ) ;
#2310=CARTESIAN_POINT ( 'NONE',  ( 30.90169943749473802, 43.08125000068280031, -42.53254041760200721 ) ) ;
#2313=CARTESIAN_POINT ( 'NONE',  ( -49.86468353124999453, 25.75937500034140015, -16.20201782572375393 ) ) ;
#2315=CARTESIAN_POINT ( 'NONE',  ( -50.00000000000000000, 47.78125000068279604, 0.000000000000000000 ) ) ;
#2318=CARTESIAN_POINT ( 'NONE',  ( 15.45084971874737789, 36.38125000068279746, 47.55282581475767500 ) ) ;
#2319=CARTESIAN_POINT ( 'NONE',  ( 50.00000000000000711, 46.90000000000000568, 16.24598481164530739 ) ) ;
#2326=CARTESIAN_POINT ( 'NONE',  ( 50.00000000000000000, 26.78125000068279959, -6.123233995736766085E-15 ) ) ;
#2327=CARTESIAN_POINT ( 'NONE',  ( 5.143516556418884111E-15, 52.00000000000000711, 42.00000000000000711 ) ) ;
#2330=CARTESIAN_POINT ( 'NONE',  ( -1.240322475938754499E-13, 36.28125000068280315, 50.00000000000000000 ) ) ;
#2332=CARTESIAN_POINT ( 'NONE',  ( 7.919222016226807881, 49.44874571845315359, -50.00000000000000000 ) ) ;
#2336=CARTESIAN_POINT ( 'NONE',  ( 15.45084971874737789, 26.60000000000000142, 47.55282581475767500 ) ) ;
#2339=CARTESIAN_POINT ( 'NONE',  ( -49.86468353125000164, 43.85937500034140157, 0.000000000000000000 ) ) ;
#2341=CARTESIAN_POINT ( 'NONE',  ( -49.86468353124999453, 25.75937500034139660, -16.20201782572375393 ) ) ;
#2344=CARTESIAN_POINT ( 'NONE',  ( 30.81806926056964002, 38.55937500034140442, 42.41743335407647209 ) ) ;
#2346=CARTESIAN_POINT ( 'NONE',  ( 1.293669679204937499E-13, 41.28125000068279604, -50.00000000000000000 ) ) ;
#2348=CARTESIAN_POINT ( 'NONE',  ( 46.25745152662987891, 25.00000000000000000, -18.62156331807923593 ) ) ;
#2349=EDGE_CURVE ( 'NONE', #11917, #15953, #722, .T. ) ;
#2357=CARTESIAN_POINT ( 'NONE',  ( 9.631387414534489405E-15, 36.42187500034139447, 52.43083105670540789 ) ) ;
#2361=CARTESIAN_POINT ( 'NONE',  ( 40.34137639590981195, 45.05937500034139731, -29.30972558990011834 ) ) ;
#2363=CARTESIAN_POINT ( 'NONE',  ( -15.45084971874737256, 21.38125000068279746, -47.55282581475767500 ) ) ;
#2368=CARTESIAN_POINT ( 'NONE',  ( 1.293669679204937499E-13, 41.50000000000000000, -50.00000000000000000 ) ) ;
#2369=CARTESIAN_POINT ( 'NONE',  ( -15.40903463028480580, 26.32187500034140015, 47.42413220539094709 ) ) ;
#2374=CARTESIAN_POINT ( 'NONE',  ( 15.40903463028482356, 34.52187500034140299, 47.42413220539093999 ) ) ;
#2379=CARTESIAN_POINT ( 'NONE',  ( -15.45084971874737256, 31.60000000000000142, -47.55282581475767500 ) ) ;
#2387=CARTESIAN_POINT ( 'NONE',  ( 0.000000000000000000, 272.0000000000000000, 0.000000000000000000 ) ) ;
#2389=CARTESIAN_POINT ( 'NONE',  ( 15.45084971874736723, 25.18125000068279817, -47.55282581475768211 ) ) ;
#2390=EDGE_LOOP ( 'NONE', ( #1940, #14090 ) ) ;
#2392=CARTESIAN_POINT ( 'NONE',  ( 49.86468353124999453, 24.95937500034139234, -16.20201782572376459 ) ) ;
#2395=ORIENTED_EDGE ( 'NONE', *, *, #10165, .T. ) ;
#2397=EDGE_LOOP ( 'NONE', ( #16288, #625, #15296, #11611 ) ) ;
#2398=CARTESIAN_POINT ( 'NONE',  ( 30.90169943749474157, 39.08125000068280031, -42.53254041760200721 ) ) ;
#2405=DIRECTION ( 'NONE',  ( -0.000000000000000000, -1.000000000000000000, -0.000000000000000000 ) ) ;
#2406=CARTESIAN_POINT ( 'NONE',  ( 15.45084971874736723, 27.18125000068279817, -47.55282581475768211 ) ) ;
#2409=LINE ( 'NONE', #16464, #4097 ) ;
#2412=CARTESIAN_POINT ( 'NONE',  ( -40.45084971874737789, 23.80000000000000071, -29.38926261462365730 ) ) ;
#2415=CARTESIAN_POINT ( 'NONE',  ( -30.81806926056962226, 42.15937500034139163, 42.41743335407647919 ) ) ;
#2417=ORIENTED_EDGE ( 'NONE', *, *, #13348, .F. ) ;
#2420=CARTESIAN_POINT ( 'NONE',  ( -15.40903463028480580, 28.25937500034139660, 47.42413220539094709 ) ) ;
#2421=CARTESIAN_POINT ( 'NONE',  ( 0.000000000000000000, 54.00000000000000711, 0.000000000000000000 ) ) ;
#2423=CARTESIAN_POINT ( 'NONE',  ( 45.67643563158024023, 25.00000000000000000, -20.00444126042648207 ) ) ;
#2425=CARTESIAN_POINT ( 'NONE',  ( 49.99999999999999289, 30.88125000068279746, -16.24598481164532160 ) ) ;
#2428=CARTESIAN_POINT ( 'NONE',  ( 50.00000000000000000, 43.00000000000000000, -6.123233995736766085E-15 ) ) ;
#2433=CARTESIAN_POINT ( 'NONE',  ( -49.86468353124999453, 33.82187500034138594, -16.20201782572375393 ) ) ;
#2437=CARTESIAN_POINT ( 'NONE',  ( 40.34137639590981195, 35.05937500034139731, -29.30972558990011834 ) ) ;
#2440=CARTESIAN_POINT ( 'NONE',  ( -3.219174618344376363E-15, 23.28125000068279959, -52.57311121191334990 ) ) ;
#2443=CARTESIAN_POINT ( 'NONE',  ( -3.210462471511496205E-15, 23.42187500034139802, -52.43083105670540789 ) ) ;
#2445=EDGE_CURVE ( 'NONE', #1138, #5870, #13520, .T. ) ;
#2448=CARTESIAN_POINT ( 'NONE',  ( 40.45084971874737789, 48.80000000000000426, 29.38926261462365375 ) ) ;
#2454=CARTESIAN_POINT ( 'NONE',  ( -40.34137639590981905, 33.72187500034139873, -29.30972558990011478 ) ) ;
#2455=CARTESIAN_POINT ( 'NONE',  ( -7.919222016226773242, 42.22999571913594963, 50.00000000000000711 ) ) ;
#2456=ORIENTED_EDGE ( 'NONE', *, *, #14582, .T. ) ;
#2472=ORIENTED_EDGE ( 'NONE', *, *, #5004, .T. ) ;
#2473=B_SPLINE_CURVE_WITH_KNOTS ( 'NONE', 3,
 ( #1469, #5396, #10455, #15512 ),
 .UNSPECIFIED., .F., .F.,
 ( 4, 4 ),
 ( 0.000000000000000000, 0.01231015999390750251 ),
 .UNSPECIFIED. ) ;
#2474=CARTESIAN_POINT ( 'NONE',  ( 30.81806926056962936, 23.15937500034139873, -42.41743335407647209 ) ) ;
#2477=EDGE_LOOP ( 'NONE', ( #3235, #12674, #6153, #11970 ) ) ;
#2482=CARTESIAN_POINT ( 'NONE',  ( 8.446640517145639571E-15, 28.49999999999999645, 50.00000000000000000 ) ) ;
#2493=CARTESIAN_POINT ( 'NONE',  ( 50.00000000000000000, 23.00000000000000355, -6.123233995736766085E-15 ) ) ;
#2496=CARTESIAN_POINT ( 'NONE',  ( 40.34137639590981905, 42.65937500034139873, 29.30972558990010768 ) ) ;
#2500=CARTESIAN_POINT ( 'NONE',  ( 49.86468353125001585, 28.75937500034139305, 16.20201782572375038 ) ) ;
#2503=CARTESIAN_POINT ( 'NONE',  ( 48.07045810499300842, 25.00000000000000000, -13.25585611146359177 ) ) ;
#2504=CARTESIAN_POINT ( 'NONE',  ( -30.81806926056962226, 32.22187500034139163, 42.41743335407647209 ) ) ;
#2509=CARTESIAN_POINT ( 'NONE',  ( 40.45084971874737079, 43.20000000000000284, -29.38926261462366440 ) ) ;
#2514=CARTESIAN_POINT ( 'NONE',  ( -30.81806926056962226, 32.22187500034139163, 42.41743335407647919 ) ) ;
#2521=CARTESIAN_POINT ( 'NONE',  ( -3.210462471511496205E-15, 39.35937500034138736, -52.43083105670540789 ) ) ;
#2523=EDGE_LOOP ( 'NONE', ( #15213, #12449 ) ) ;
#2524=VERTEX_POINT ( 'NONE', #2327 ) ;
#2526=CARTESIAN_POINT ( 'NONE',  ( -15.40903463028481646, 49.45937500034140299, -47.42413220539093999 ) ) ;
#2529=CARTESIAN_POINT ( 'NONE',  ( 9.631387414534489405E-15, 26.42187500034139447, 52.43083105670540789 ) ) ;
#2532=VECTOR ( 'NONE', #14359, 1000.000000000000000 ) ;
#2533=CARTESIAN_POINT ( 'NONE',  ( -49.99999999999999289, 48.10000000000000142, 16.24598481164533226 ) ) ;
#2536=CARTESIAN_POINT ( 'NONE',  ( -30.81806926056963292, 47.62187500034139731, -42.41743335407647209 ) ) ;
#2542=AXIS2_PLACEMENT_3D ( 'NONE', #15257, #6388, #7868 ) ;
#2545=CARTESIAN_POINT ( 'NONE',  ( -40.45084971874737079, 32.20000000000000284, 29.38926261462367151 ) ) ;
#2547=ADVANCED_FACE ( 'NONE', ( #2156 ), #7245, .T. ) ;
#2555=CARTESIAN_POINT ( 'NONE',  ( -30.90169943749474513, 39.69999999999999574, -42.53254041760200721 ) ) ;
#2562=CARTESIAN_POINT ( 'NONE',  ( 49.86468353125000164, 22.85937500034139802, -6.106662507704105588E-15 ) ) ;
#2566=ORIENTED_EDGE ( 'NONE', *, *, #5224, .T. ) ;
#2569=CARTESIAN_POINT ( 'NONE',  ( 0.000000000000000000, 193.4213562373095385, -50.00000000000000000 ) ) ;
#2575=DIRECTION ( 'NONE',  ( -0.000000000000000000, -1.000000000000000000, -0.000000000000000000 ) ) ;
#2582=CARTESIAN_POINT ( 'NONE',  ( -3.219174618344376363E-15, 21.50000000000000355, -52.57311121191334990 ) ) ;
#2586=VECTOR ( 'NONE', #7969, 1000.000000000000000 ) ;
#2587=CARTESIAN_POINT ( 'NONE',  ( -40.34137639590981195, 44.05937500034139731, 29.30972558990012189 ) ) ;
#2591=CARTESIAN_POINT ( 'NONE',  ( 49.86468353125000164, 28.85937500034139802, -6.106662507704105588E-15 ) ) ;
#2594=CARTESIAN_POINT ( 'NONE',  ( 45.25922935877483155, 25.00000000000000000, -20.93126818148093804 ) ) ;
#2595=CARTESIAN_POINT ( 'NONE',  ( 40.34137639590981195, 33.12187500034139731, -29.30972558990011834 ) ) ;
#2604=CARTESIAN_POINT ( 'NONE',  ( -30.81806926056962226, 30.22187500034139518, 42.41743335407647919 ) ) ;
#2607=ORIENTED_EDGE ( 'NONE', *, *, #7708, .F. ) ;
#2608=ORIENTED_EDGE ( 'NONE', *, *, #657, .F. ) ;
#2609=CARTESIAN_POINT ( 'NONE',  ( 49.86468353125001585, 38.75937500034139305, 16.20201782572375038 ) ) ;
#2611=ORIENTED_EDGE ( 'NONE', *, *, #1818, .F. ) ;
#2613=CARTESIAN_POINT ( 'NONE',  ( 49.86468353125001585, 48.75937500034140015, 16.20201782572375038 ) ) ;
#2615=CARTESIAN_POINT ( 'NONE',  ( 15.40903463028482356, 26.52187500034139589, 47.42413220539093999 ) ) ;
#2620=CARTESIAN_POINT ( 'NONE',  ( -30.90169943749474513, 25.48125000068279888, -42.53254041760200721 ) ) ;
#2621=CARTESIAN_POINT ( 'NONE',  ( 15.40903463028482356, 20.52187500034139589, 47.42413220539093999 ) ) ;
#2638=CARTESIAN_POINT ( 'NONE',  ( -30.90169943749474513, 35.48125000068279888, -42.53254041760200721 ) ) ;
#2642=CARTESIAN_POINT ( 'NONE',  ( 30.81806926056962936, 21.15937500034140228, -42.41743335407647209 ) ) ;
#2643=ORIENTED_EDGE ( 'NONE', *, *, #11408, .F. ) ;
#2645=ORIENTED_EDGE ( 'NONE', *, *, #3926, .T. ) ;
#2652=CARTESIAN_POINT ( 'NONE',  ( 7.919222016226809657, 29.44874571845315359, -50.00000000000000000 ) ) ;
#2662=CARTESIAN_POINT ( 'NONE',  ( 9.657523855033129090E-15, 24.50000000000000355, 52.57311121191334990 ) ) ;
#2665=CARTESIAN_POINT ( 'NONE',  ( -30.81806926056962226, 44.15937500034139163, 42.41743335407647919 ) ) ;
#2670=CARTESIAN_POINT ( 'NONE',  ( 15.40903463028482356, 26.45937500034139589, 47.42413220539093999 ) ) ;
#2671=ORIENTED_EDGE ( 'NONE', *, *, #15404, .T. ) ;
#2674=CARTESIAN_POINT ( 'NONE',  ( 47.24032962522667134, 25.00000000000000711, -15.96451374291363301 ) ) ;
#2675=CARTESIAN_POINT ( 'NONE',  ( -49.86468353124999453, 31.82187500034139305, -16.20201782572375393 ) ) ;
#2676=CARTESIAN_POINT ( 'NONE',  ( 15.45084971874737789, 30.38125000068280102, 47.55282581475767500 ) ) ;
#2680=CARTESIAN_POINT ( 'NONE',  ( 0.000000000000000000, 52.00000000000000711, 65.00000000000000000 ) ) ;
#2683=CARTESIAN_POINT ( 'NONE',  ( -49.86468353124999453, 34.02187500034140299, 16.20201782572377525 ) ) ;
#2686=CARTESIAN_POINT ( 'NONE',  ( 30.81806926056964002, 36.55937500034139731, 42.41743335407646498 ) ) ;
#2690=CARTESIAN_POINT ( 'NONE',  ( 49.86468353124999453, 46.95937500034139589, -16.20201782572376459 ) ) ;
#2692=CARTESIAN_POINT ( 'NONE',  ( 49.86468353124999453, 25.02187500034139589, -16.20201782572376459 ) ) ;
#2697=CARTESIAN_POINT ( 'NONE',  ( 15.45084971874737789, 44.60000000000000142, 47.55282581475767500 ) ) ;
#2704=CARTESIAN_POINT ( 'NONE',  ( -30.90169943749474868, 37.48125000068279888, -42.53254041760200721 ) ) ;
#2709=CARTESIAN_POINT ( 'NONE',  ( -3.210462471511496205E-15, 49.42187500034138736, -52.43083105670540789 ) ) ;
#2714=CARTESIAN_POINT ( 'NONE',  ( 15.45084971874737789, 34.38125000068280457, 47.55282581475767500 ) ) ;
#2719=CARTESIAN_POINT ( 'NONE',  ( -15.40903463028480580, 46.32187500034140015, 47.42413220539094709 ) ) ;
#2727=CARTESIAN_POINT ( 'NONE',  ( 7.919222016226822092, 28.55125428154684286, 49.99999999999999289 ) ) ;
#2730=CARTESIAN_POINT ( 'NONE',  ( 2.600676159226421000E-13, 31.49999999999999289, -49.99999999999999289 ) ) ;
#2734=CARTESIAN_POINT ( 'NONE',  ( 40.45084971874737789, 48.80000000000000426, 29.38926261462365375 ) ) ;
#2737=CARTESIAN_POINT ( 'NONE',  ( -15.45084971874737256, 21.60000000000000142, -47.55282581475767500 ) ) ;
#2742=CARTESIAN_POINT ( 'NONE',  ( -40.34137639590981905, 37.65937500034139873, -29.30972558990011478 ) ) ;
#2748=CARTESIAN_POINT ( 'NONE',  ( -49.86468353124999453, 29.75937500034139305, -16.20201782572375393 ) ) ;
#2750=CARTESIAN_POINT ( 'NONE',  ( 30.90169943749475223, 26.70000000000000284, 42.53254041760199300 ) ) ;
#2753=CARTESIAN_POINT ( 'NONE',  ( 15.40903463028482356, 36.52187500034139589, 47.42413220539093999 ) ) ;
#2763=CARTESIAN_POINT ( 'NONE',  ( -40.34137639590981195, 34.12187500034139731, 29.30972558990012189 ) ) ;
#2767=PRODUCT_DEFINITION_CONTEXT ( 'detailed design', #16090, 'design' ) ;
#2768=CARTESIAN_POINT ( 'NONE',  ( -30.81806926056963292, 37.55937500034139020, -42.41743335407646498 ) ) ;
#2771=CARTESIAN_POINT ( 'NONE',  ( -30.81806926056963292, 49.55937500034139731, -42.41743335407647209 ) ) ;
#2774=CARTESIAN_POINT ( 'NONE',  ( -40.34137639590981195, 24.12187500034139731, 29.30972558990012189 ) ) ;
#2780=CARTESIAN_POINT ( 'NONE',  ( -30.90169943749474868, 47.70000000000000995, -42.53254041760200721 ) ) ;
#2786=DIRECTION ( 'NONE',  ( -0.000000000000000000, -1.000000000000000000, -0.000000000000000000 ) ) ;
#2788=CARTESIAN_POINT ( 'NONE',  ( -50.00000000000000000, 37.78125000068280315, 0.000000000000000000 ) ) ;
#2794=CARTESIAN_POINT ( 'NONE',  ( -3.210462471511496205E-15, 47.42187500034138736, -52.43083105670540789 ) ) ;
#2803=ORIENTED_EDGE ( 'NONE', *, *, #2952, .F. ) ;
#2805=CARTESIAN_POINT ( 'NONE',  ( -3.210462471511496205E-15, 47.42187500034138736, -52.43083105670540789 ) ) ;
#2810=VERTEX_POINT ( 'NONE', #4162 ) ;
#2820=CIRCLE ( 'NONE', #681, 2.000000000000001776 ) ;
#2832=CARTESIAN_POINT ( 'NONE',  ( -30.81806926056962226, 40.15937500034139163, 42.41743335407647919 ) ) ;
#2836=CARTESIAN_POINT ( 'NONE',  ( -15.45084971874737256, 49.38125000068280457, -47.55282581475767500 ) ) ;
#2838=CARTESIAN_POINT ( 'NONE',  ( 30.81806926056962936, 25.15937500034139518, -42.41743335407647209 ) ) ;
#2840=DIRECTION ( 'NONE',  ( 0.000000000000000000, 0.000000000000000000, 1.000000000000000000 ) ) ;
#2844=CARTESIAN_POINT ( 'NONE',  ( -40.34137639590981905, 29.72187500034139518, -29.30972558990011478 ) ) ;
#2854=CARTESIAN_POINT ( 'NONE',  ( -49.86468353125000164, 27.92187500034139447, 0.000000000000000000 ) ) ;
#2858=CARTESIAN_POINT ( 'NONE',  ( -15.40903463028481646, 27.45937500034139944, -47.42413220539093999 ) ) ;
#2861=CARTESIAN_POINT ( 'NONE',  ( 40.34137639590981905, 48.65937500034139873, 29.30972558990010768 ) ) ;
#2864=CARTESIAN_POINT ( 'NONE',  ( 30.81806926056964002, 20.62187500034139020, 42.41743335407647209 ) ) ;
#2870=CARTESIAN_POINT ( 'NONE',  ( 9.657523855033129090E-15, 38.50000000000000711, 52.57311121191334990 ) ) ;
#2873=CARTESIAN_POINT ( 'NONE',  ( 49.86468353125000164, 44.92187500034140157, -6.106662507704105588E-15 ) ) ;
#2878=CARTESIAN_POINT ( 'NONE',  ( -50.00000000000000000, 35.78125000068280315, 0.000000000000000000 ) ) ;
#2882=DIRECTION ( 'NONE',  ( -0.000000000000000000, -1.000000000000000000, -0.000000000000000000 ) ) ;
#2884=CARTESIAN_POINT ( 'NONE',  ( -49.86468353124999453, 47.82187500034140015, -16.20201782572375393 ) ) ;
#2886=ADVANCED_FACE ( 'NONE', ( #14199, #11958 ), #12968, .F. ) ;
#2891=EDGE_CURVE ( 'NONE', #12805, #6547, #3145, .T. ) ;
#2894=CARTESIAN_POINT ( 'NONE',  ( 8.446640517145639571E-15, 28.28125000068279959, 50.00000000000000000 ) ) ;
#2896=CARTESIAN_POINT ( 'NONE',  ( -3.210462471511496205E-15, 45.42187500034139447, -52.43083105670540789 ) ) ;
#2911=CARTESIAN_POINT ( 'NONE',  ( -7.919222016226752814, 37.33250428222964246, -50.00000000000000711 ) ) ;
#2916=ORIENTED_EDGE ( 'NONE', *, *, #14086, .F. ) ;
#2917=CARTESIAN_POINT ( 'NONE',  ( -30.81806926056963292, 37.55937500034139020, -42.41743335407647209 ) ) ;
#2920=CARTESIAN_POINT ( 'NONE',  ( 40.45084971874737079, 46.98125000068280599, -29.38926261462366440 ) ) ;
#2922=CARTESIAN_POINT ( 'NONE',  ( 49.86468353124999453, 24.95937500034139234, -16.20201782572376459 ) ) ;
#2927=CARTESIAN_POINT ( 'NONE',  ( 49.86468353125001585, 26.82187500034139305, 16.20201782572375038 ) ) ;
#2933=CARTESIAN_POINT ( 'NONE',  ( -15.45084971874737256, 33.60000000000000142, -47.55282581475767500 ) ) ;
#2936=ORIENTED_EDGE ( 'NONE', *, *, #3693, .T. ) ;
#2938=CARTESIAN_POINT ( 'NONE',  ( 40.34137639590981905, 26.65937500034139518, 29.30972558990010768 ) ) ;
#2941=CARTESIAN_POINT ( 'NONE',  ( -15.40903463028480580, 44.25937500034140015, 47.42413220539094709 ) ) ;
#2948=CARTESIAN_POINT ( 'NONE',  ( -3.219174618344376363E-15, 43.50000000000000000, -52.57311121191334990 ) ) ;
#2950=CARTESIAN_POINT ( 'NONE',  ( -40.34137639590981195, 46.12187500034139731, 29.30972558990012189 ) ) ;
#2952=EDGE_CURVE ( 'NONE', #7138, #5789, #10642, .T. ) ;
#2953=CARTESIAN_POINT ( 'NONE',  ( 30.81806926056964002, 46.55937500034139020, 42.41743335407646498 ) ) ;
#2955=CARTESIAN_POINT ( 'NONE',  ( -15.45084971874737256, 29.38125000068279746, -47.55282581475767500 ) ) ;
#2961=CARTESIAN_POINT ( 'NONE',  ( -15.40903463028481646, 49.52187500034140299, -47.42413220539093999 ) ) ;
#2963=DIRECTION ( 'NONE',  ( 0.000000000000000000, 0.000000000000000000, 1.000000000000000000 ) ) ;
#2969=CARTESIAN_POINT ( 'NONE',  ( -30.90169943749474513, 45.48125000068279178, -42.53254041760200721 ) ) ;
#2971=CARTESIAN_POINT ( 'NONE',  ( -3.210462471511496205E-15, 21.35937500034139092, -52.43083105670540789 ) ) ;
#2982=EDGE_CURVE ( 'NONE', #6547, #1767, #508, .T. ) ;
#2992=CARTESIAN_POINT ( 'NONE',  ( -40.34137639590981905, 35.65937500034139873, -29.30972558990011478 ) ) ;
#2997=CARTESIAN_POINT ( 'NONE',  ( 15.40903463028482356, 22.45937500034139589, 47.42413220539093999 ) ) ;
#3003=CARTESIAN_POINT ( 'NONE',  ( -40.34137639590981905, 25.72187500034139518, -29.30972558990011478 ) ) ;
#3009=CARTESIAN_POINT ( 'NONE',  ( 30.90169943749475578, 36.70000000000000995, 42.53254041760200010 ) ) ;
#3013=ORIENTED_EDGE ( 'NONE', *, *, #8619, .F. ) ;
#3014=CARTESIAN_POINT ( 'NONE',  ( 49.86468353125000164, 28.85937500034139802, -6.106662507704105588E-15 ) ) ;
#3017=CARTESIAN_POINT ( 'NONE',  ( 40.34137639590981195, 41.05937500034139731, -29.30972558990011834 ) ) ;
#3020=AXIS2_PLACEMENT_3D ( 'NONE', #6336, #16384, #15288 ) ;
#3025=CARTESIAN_POINT ( 'NONE',  ( 40.45084971874737079, 43.20000000000000284, -29.38926261462366440 ) ) ;
#3027=CARTESIAN_POINT ( 'NONE',  ( -40.34137639590981195, 42.12187500034139731, 29.30972558990012189 ) ) ;
#3032=ORIENTED_EDGE ( 'NONE', *, *, #1513, .F. ) ;
#3033=CARTESIAN_POINT ( 'NONE',  ( -30.90169943749474868, 29.48125000068279888, -42.53254041760200721 ) ) ;
#3037=CARTESIAN_POINT ( 'NONE',  ( -40.34137639590981195, 44.12187500034139731, 29.30972558990012189 ) ) ;
#3039=EDGE_CURVE ( 'NONE', #8435, #436, #6579, .T. ) ;
#3040=CONICAL_SURFACE ( 'NONE', #12336, 65.00000000000000000, 0.08726646259971666819 ) ;
#3047=CARTESIAN_POINT ( 'NONE',  ( -30.81806926056962226, 42.22187500034139163, 42.41743335407647919 ) ) ;
#3048=EDGE_LOOP ( 'NONE', ( #4640, #11034, #186, #6569 ) ) ;
#3051=VECTOR ( 'NONE', #3664, 1000.000000000000000 ) ;
#3053=CARTESIAN_POINT ( 'NONE',  ( 0.000000000000000000, 272.0000000000000000, 0.000000000000000000 ) ) ;
#3056=CARTESIAN_POINT ( 'NONE',  ( 6.123233995736766085E-15, 193.4213562373095385, 50.00000000000000000 ) ) ;
#3059=CARTESIAN_POINT ( 'NONE',  ( 40.45084971874737789, 48.58125000068280031, 29.38926261462365375 ) ) ;
#3061=FACE_BOUND ( 'NONE', #2390, .T. ) ;
#3067=EDGE_CURVE ( 'NONE', #5789, #15481, #12823, .T. ) ;
#3071=CARTESIAN_POINT ( 'NONE',  ( 9.631387414534489405E-15, 34.35937500034139447, 52.43083105670540789 ) ) ;
#3074=CARTESIAN_POINT ( 'NONE',  ( 50.00000000000000000, 48.78125000068279604, -6.123233995736766085E-15 ) ) ;
#3079=CARTESIAN_POINT ( 'NONE',  ( -40.34137639590981905, 25.65937500034139518, -29.30972558990011478 ) ) ;
#3086=CARTESIAN_POINT ( 'NONE',  ( 48.35726954556789536, 24.99999999999999645, -12.16803787670825265 ) ) ;
#3095=CARTESIAN_POINT ( 'NONE',  ( 50.00000000000000711, 32.89999999999999147, 16.24598481164530739 ) ) ;
#3101=CARTESIAN_POINT ( 'NONE',  ( 49.86468353124999453, 32.95937500034138878, -16.20201782572376104 ) ) ;
#3102=ORIENTED_EDGE ( 'NONE', *, *, #5714, .F. ) ;
#3104=CARTESIAN_POINT ( 'NONE',  ( 30.81806926056964002, 42.55937500034139020, 42.41743335407647209 ) ) ;
#3114=CARTESIAN_POINT ( 'NONE',  ( 40.34137639590981195, 31.12187500034139731, -29.30972558990011834 ) ) ;
#3115=CARTESIAN_POINT ( 'NONE',  ( -40.45084971874737079, 44.20000000000000284, 29.38926261462367151 ) ) ;
#3117=CARTESIAN_POINT ( 'NONE',  ( 15.40903463028482356, 44.52187500034139589, 47.42413220539093999 ) ) ;
#3122=CARTESIAN_POINT ( 'NONE',  ( -30.81806926056963292, 47.55937500034139731, -42.41743335407646498 ) ) ;
#3123=ORIENTED_EDGE ( 'NONE', *, *, #8180, .T. ) ;
#3124=CARTESIAN_POINT ( 'NONE',  ( -15.45084971874736368, 32.18125000068279462, 47.55282581475768211 ) ) ;
#3128=CARTESIAN_POINT ( 'NONE',  ( -15.40903463028480580, 38.32187500034140015, 47.42413220539094709 ) ) ;
#3130=CARTESIAN_POINT ( 'NONE',  ( 0.000000000000000000, 52.00000000000000711, 0.000000000000000000 ) ) ;
#3136=CARTESIAN_POINT ( 'NONE',  ( -49.86468353124999453, 42.02187500034139589, 16.20201782572377525 ) ) ;
#3137=EDGE_LOOP ( 'NONE', ( #3032, #5277, #14535, #2645 ) ) ;
#3138=ORIENTED_EDGE ( 'NONE', *, *, #5655, .T. ) ;
#3141=DIRECTION ( 'NONE',  ( -0.000000000000000000, -1.000000000000000000, -0.000000000000000000 ) ) ;
#3145=LINE ( 'NONE', #8219, #6902 ) ;
#3154=CARTESIAN_POINT ( 'NONE',  ( 49.86468353124999453, 28.95937500034139944, -16.20201782572376459 ) ) ;
#3161=MANIFOLD_SOLID_BREP ( 'Cavity1', #12370 ) ;
#3162=CARTESIAN_POINT ( 'NONE',  ( -15.45084971874737256, 47.38125000068279746, -47.55282581475767500 ) ) ;
#3163=AXIS2_PLACEMENT_3D ( 'NONE', #12305, #1072, #6001 ) ;
#3165=CARTESIAN_POINT ( 'NONE',  ( -15.40903463028480580, 24.25937500034139660, 47.42413220539094709 ) ) ;
#3168=CARTESIAN_POINT ( 'NONE',  ( 2.978552182361884590E-14, 47.50000000000000711, -50.00000000000000000 ) ) ;
#3171=CARTESIAN_POINT ( 'NONE',  ( 49.86468353125000164, 28.92187500034139802, -6.106662507704105588E-15 ) ) ;
#3177=CARTESIAN_POINT ( 'NONE',  ( 30.90169943749474157, 33.30000000000000426, -42.53254041760200721 ) ) ;
#3179=CARTESIAN_POINT ( 'NONE',  ( -15.40903463028481646, 47.45937500034139589, -47.42413220539093999 ) ) ;
#3181=CARTESIAN_POINT ( 'NONE',  ( 49.86468353125000164, 30.85937500034139802, -6.106662507704105588E-15 ) ) ;
#3184=CARTESIAN_POINT ( 'NONE',  ( 40.34137639590981905, 40.65937500034139873, 29.30972558990010768 ) ) ;
#3185=DIRECTION ( 'NONE',  ( 0.000000000000000000, 1.000000000000000000, 0.000000000000000000 ) ) ;
#3186=CARTESIAN_POINT ( 'NONE',  ( 7.919222016226791006, 44.33250428222964246, 50.00000000000000711 ) ) ;
#3191=CARTESIAN_POINT ( 'NONE',  ( -49.86468353124999453, 32.02187500034139589, 16.20201782572377525 ) ) ;
#3192=CARTESIAN_POINT ( 'NONE',  ( 40.45084971874737789, 38.80000000000000426, 29.38926261462365375 ) ) ;
#3194=CARTESIAN_POINT ( 'NONE',  ( -30.81806926056963292, 41.62187500034139020, -42.41743335407647209 ) ) ;
#3200=CARTESIAN_POINT ( 'NONE',  ( 15.45084971874736723, 33.18125000068279462, -47.55282581475768211 ) ) ;
#3204=CARTESIAN_POINT ( 'NONE',  ( -30.81806926056962226, 42.22187500034139163, 42.41743335407647209 ) ) ;
#3212=CARTESIAN_POINT ( 'NONE',  ( -49.99999999999999289, 45.68125000068280173, -16.24598481164531449 ) ) ;
#3214=CARTESIAN_POINT ( 'NONE',  ( -49.86468353124999453, 40.02187500034140299, 16.20201782572377525 ) ) ;
#3224=CARTESIAN_POINT ( 'NONE',  ( 15.45084971874736723, 25.40000000000000213, -47.55282581475768211 ) ) ;
#3233=CARTESIAN_POINT ( 'NONE',  ( 15.40903463028482356, 28.45937500034139589, 47.42413220539093999 ) ) ;
#3234=VERTEX_POINT ( 'NONE', #11620 ) ;
#3235=ORIENTED_EDGE ( 'NONE', *, *, #11996, .F. ) ;
#3237=CARTESIAN_POINT ( 'NONE',  ( 15.45084971874737789, 42.38125000068279746, 47.55282581475767500 ) ) ;
#3241=CARTESIAN_POINT ( 'NONE',  ( -7.919222016226870942, 38.44874571845316069, 49.99999999999997158 ) ) ;
#3253=CYLINDRICAL_SURFACE ( 'NONE', #7628, 50.00000000000000000 ) ;
#3254=CARTESIAN_POINT ( 'NONE',  ( 40.45084971874737789, 36.79999999999999716, 29.38926261462365375 ) ) ;
#3256=CARTESIAN_POINT ( 'NONE',  ( -3.210462471511496205E-15, 47.35937500034138736, -52.43083105670540789 ) ) ;
#3257=ORIENTED_EDGE ( 'NONE', *, *, #534, .T. ) ;
#3263=CARTESIAN_POINT ( 'NONE',  ( 15.40903463028482356, 44.45937500034139589, 47.42413220539093999 ) ) ;
#3267=LINE ( 'NONE', #8335, #5665 ) ;
#3272=CARTESIAN_POINT ( 'NONE',  ( 49.86468353124999453, 31.02187500034139234, -16.20201782572376459 ) ) ;
#3276=CARTESIAN_POINT ( 'NONE',  ( 49.86468353124999453, 37.02187500034138878, -16.20201782572376459 ) ) ;
#3280=CARTESIAN_POINT ( 'NONE',  ( -30.81806926056962226, 40.15937500034139163, 42.41743335407647209 ) ) ;
#3282=CARTESIAN_POINT ( 'NONE',  ( -40.45084971874737789, 31.58125000068280031, -29.38926261462365730 ) ) ;
#3284=ORIENTED_EDGE ( 'NONE', *, *, #7560, .T. ) ;
#3286=CARTESIAN_POINT ( 'NONE',  ( 49.86468353125001585, 40.82187500034140726, 16.20201782572375038 ) ) ;
#3289=CARTESIAN_POINT ( 'NONE',  ( -49.86468353124999453, 26.02187500034139944, 16.20201782572377525 ) ) ;
#3292=AXIS2_PLACEMENT_3D ( 'NONE', #10396, #5417, #15533 ) ;
#3296=CARTESIAN_POINT ( 'NONE',  ( 15.40903463028482356, 44.52187500034139589, 47.42413220539093999 ) ) ;
#3297=ORIENTED_EDGE ( 'NONE', *, *, #9014, .F. ) ;
#3298=ORIENTED_EDGE ( 'NONE', *, *, #14234, .F. ) ;
#3299=( BOUNDED_CURVE ( )  B_SPLINE_CURVE ( 2, ( #13870, #14039, #2406, #6490, #11546, #4846, #2326, #7410, #6162, #1238, #12552, #15121, #16461 ),
 .UNSPECIFIED., .F., .F. ) 
 B_SPLINE_CURVE_WITH_KNOTS ( ( 3, 2, 2, 2, 2, 2, 3 ),
 ( 0.7500000000000000000, 0.7533333333333332993, 0.7600000000000000089, 0.7666666666666667185, 0.7733333333333333171, 0.7800000000000000266, 0.7833333333333333259 ),
 .UNSPECIFIED. ) 
 CURVE ( )  GEOMETRIC_REPRESENTATION_ITEM ( )  RATIONAL_B_SPLINE_CURVE ( ( 0.9755282581475768211, 0.9755282581475768211, 1.000000000000000000, 0.9510565162951535312, 1.000000000000000000, 0.9510565162951535312, 1.000000000000000000, 0.9510565162951535312, 1.000000000000000000, 0.9510565162951535312, 1.000000000000000000, 0.9755282581475768211, 0.9755282581475768211 ) ) 
 REPRESENTATION_ITEM ( '' )  );
#3303=AXIS2_PLACEMENT_3D ( 'NONE', #2387, #11295, #16355 ) ;
#3308=CARTESIAN_POINT ( 'NONE',  ( -7.919222016226934890, 30.44874571845316069, 49.99999999999996447 ) ) ;
#3312=CARTESIAN_POINT ( 'NONE',  ( 40.45084971874737789, 42.58125000068280031, 29.38926261462365375 ) ) ;
#3315=AXIS2_PLACEMENT_3D ( 'NONE', #10769, #13179, #10615 ) ;
#3316=CARTESIAN_POINT ( 'NONE',  ( -30.81806926056962226, 30.15937500034139163, 42.41743335407647919 ) ) ;
#3321=CARTESIAN_POINT ( 'NONE',  ( -40.45084971874737079, 41.98125000068279888, 29.38926261462367151 ) ) ;
#3324=ORIENTED_EDGE ( 'NONE', *, *, #1297, .T. ) ;
#3330=CARTESIAN_POINT ( 'NONE',  ( 38.60409515610501074, 25.00000000000000000, -31.77615201968907144 ) ) ;
#3331=VECTOR ( 'NONE', #6236, 1000.000000000000000 ) ;
#3338=CARTESIAN_POINT ( 'NONE',  ( -15.45084971874737256, 25.60000000000000142, -47.55282581475767500 ) ) ;
#3348=CARTESIAN_POINT ( 'NONE',  ( 15.40903463028481113, 33.25937500034140015, -47.42413220539094709 ) ) ;
#3349=DIRECTION ( 'NONE',  ( 0.000000000000000000, 0.000000000000000000, -1.000000000000000000 ) ) ;
#3351=DIRECTION ( 'NONE',  ( -0.000000000000000000, -1.000000000000000000, -0.000000000000000000 ) ) ;
#3358=CARTESIAN_POINT ( 'NONE',  ( 40.34137639590981905, 30.72187500034139518, 29.30972558990010768 ) ) ;
#3361=CARTESIAN_POINT ( 'NONE',  ( 49.86468353125000164, 34.92187500034140157, -6.106662507704105588E-15 ) ) ;
#3365=ORIENTED_EDGE ( 'NONE', *, *, #8445, .T. ) ;
#3366=CARTESIAN_POINT ( 'NONE',  ( 9.631387414534489405E-15, 42.35937500034140157, 52.43083105670540789 ) ) ;
#3367=AXIS2_PLACEMENT_3D ( 'NONE', #15719, #9087, #6775 ) ;
#3370=CARTESIAN_POINT ( 'NONE',  ( 49.99999999999999289, 24.88125000068279746, -16.24598481164532160 ) ) ;
#3371=ADVANCED_FACE ( 'NONE', ( #14786 ), #11066, .T. ) ;
#3372=EDGE_CURVE ( 'NONE', #1863, #7138, #8788, .T. ) ;
#3376=CARTESIAN_POINT ( 'NONE',  ( 30.81806926056962936, 41.22187500034139873, -42.41743335407646498 ) ) ;
#3378=CARTESIAN_POINT ( 'NONE',  ( 7.919222016226693306, 30.55125428154684286, 50.00000000000003553 ) ) ;
#3379=CARTESIAN_POINT ( 'NONE',  ( -3.210462471511496205E-15, 21.42187500034139802, -52.43083105670540789 ) ) ;
#3386=CARTESIAN_POINT ( 'NONE',  ( 9.631387414534489405E-15, 42.42187500034140157, 52.43083105670540789 ) ) ;
#3387=CARTESIAN_POINT ( 'NONE',  ( -5.823736356558307894E-14, 44.28125000068280315, 50.00000000000000000 ) ) ;
#3392=EDGE_CURVE ( 'NONE', #16058, #13965, #8169, .T. ) ;
#3403=DIRECTION ( 'NONE',  ( -0.000000000000000000, -1.000000000000000000, -0.000000000000000000 ) ) ;
#3404=CARTESIAN_POINT ( 'NONE',  ( -40.45084971874737789, 33.80000000000000426, -29.38926261462365730 ) ) ;
#3407=( BOUNDED_CURVE ( )  B_SPLINE_CURVE ( 2, ( #5885, #2455, #13762, #9949, #16341, #7458, #15004, #4638, #13677, #3642, #12525, #8696, #6213 ),
 .UNSPECIFIED., .F., .F. ) 
 B_SPLINE_CURVE_WITH_KNOTS ( ( 3, 2, 2, 2, 2, 2, 3 ),
 ( 0.2500000000000000000, 0.2533333333333333548, 0.2600000000000000089, 0.2666666666666666630, 0.2733333333333333171, 0.2800000000000000266, 0.2833333333333333814 ),
 .UNSPECIFIED. ) 
 CURVE ( )  GEOMETRIC_REPRESENTATION_ITEM ( )  RATIONAL_B_SPLINE_CURVE ( ( 0.9755282581475765991, 0.9755282581475765991, 1.000000000000000000, 0.9510565162951535312, 1.000000000000000000, 0.9510565162951535312, 1.000000000000000000, 0.9510565162951535312, 1.000000000000000000, 0.9510565162951535312, 1.000000000000000000, 0.9755282581475765991, 0.9755282581475768211 ) ) 
 REPRESENTATION_ITEM ( '' )  );
#3408=CARTESIAN_POINT ( 'NONE',  ( 49.86468353124999453, 32.95937500034138168, -16.20201782572376459 ) ) ;
#3410=ORIENTED_EDGE ( 'NONE', *, *, #11996, .T. ) ;
#3412=CARTESIAN_POINT ( 'NONE',  ( -30.90169943749474868, 43.48125000068279178, -42.53254041760200721 ) ) ;
#3413=CARTESIAN_POINT ( 'NONE',  ( 30.90169943749475223, 46.69999999999999574, 42.53254041760199300 ) ) ;
#3417=CARTESIAN_POINT ( 'NONE',  ( -3.111920190527341144E-15, 27.28125000068279604, -50.00000000000000000 ) ) ;
#3421=FACE_OUTER_BOUND ( 'NONE', #920, .T. ) ;
#3424=FACE_OUTER_BOUND ( 'NONE', #5431, .T. ) ;
#3430=CARTESIAN_POINT ( 'NONE',  ( 40.45084971874737079, 29.19999999999999929, -29.38926261462366440 ) ) ;
#3434=EDGE_LOOP ( 'NONE', ( #6959, #1307, #15382, #3013 ) ) ;
#3437=CARTESIAN_POINT ( 'NONE',  ( 30.81806926056964002, 34.55937500034139731, 42.41743335407647209 ) ) ;
#3438=DIRECTION ( 'NONE',  ( -0.000000000000000000, -1.000000000000000000, -0.000000000000000000 ) ) ;
#3446=CARTESIAN_POINT ( 'NONE',  ( 49.86468353125001585, 30.82187500034139660, 16.20201782572375038 ) ) ;
#3447=CARTESIAN_POINT ( 'NONE',  ( 40.45084971874737789, 32.80000000000000426, 29.38926261462365375 ) ) ;
#3449=CARTESIAN_POINT ( 'NONE',  ( 30.81806926056964002, 36.62187500034139731, 42.41743335407647209 ) ) ;
#3452=AXIS2_PLACEMENT_3D ( 'NONE', #8398, #5997, #5915 ) ;
#3453=CARTESIAN_POINT ( 'NONE',  ( -15.40903463028480580, 42.25937500034139305, 47.42413220539094709 ) ) ;
#3455=CARTESIAN_POINT ( 'NONE',  ( -49.99999999999999289, 25.68125000068279462, -16.24598481164531449 ) ) ;
#3458=CARTESIAN_POINT ( 'NONE',  ( -15.40903463028480580, 40.32187500034140015, 47.42413220539094709 ) ) ;
#3460=CARTESIAN_POINT ( 'NONE',  ( 40.45084971874737789, 40.80000000000000426, 29.38926261462365375 ) ) ;
#3461=CARTESIAN_POINT ( 'NONE',  ( -40.34137639590981905, 25.72187500034139518, -29.30972558990011478 ) ) ;
#3465=EDGE_CURVE ( 'NONE', #14577, #6674, #9030, .T. ) ;
#3467=CARTESIAN_POINT ( 'NONE',  ( 6.123233995736766085E-15, 193.4213562373095385, 50.00000000000000000 ) ) ;
#3469=CARTESIAN_POINT ( 'NONE',  ( 9.631387414534489405E-15, 36.42187500034139447, 52.43083105670540789 ) ) ;
#3470=CARTESIAN_POINT ( 'NONE',  ( -7.919222016226816763, 43.33250428222963535, -49.99999999999999289 ) ) ;
#3473=VERTEX_POINT ( 'NONE', #3742 ) ;
#3478=DIRECTION ( 'NONE',  ( 0.000000000000000000, 0.000000000000000000, -1.000000000000000000 ) ) ;
#3490=CARTESIAN_POINT ( 'NONE',  ( 40.34137639590981905, 26.65937500034139518, 29.30972558990010768 ) ) ;
#3492=VERTEX_POINT ( 'NONE', #7650 ) ;
#3494=CARTESIAN_POINT ( 'NONE',  ( 30.90169943749475578, 46.48125000068280599, 42.53254041760200010 ) ) ;
#3509=( BOUNDED_CURVE ( )  B_SPLINE_CURVE ( 2, ( #8487, #12230, #12402, #12307, #12150, #13310, #5924, #994, #13631, #11162, #9748, #14793, #13553 ),
 .UNSPECIFIED., .F., .T. ) 
 B_SPLINE_CURVE_WITH_KNOTS ( ( 3, 2, 2, 2, 2, 2, 3 ),
 ( 0.2500000000000000000, 0.2533333333333333548, 0.2600000000000000089, 0.2666666666666666630, 0.2733333333333333171, 0.2800000000000000266, 0.2833333333333333814 ),
 .UNSPECIFIED. ) 
 CURVE ( )  GEOMETRIC_REPRESENTATION_ITEM ( )  RATIONAL_B_SPLINE_CURVE ( ( 0.9755282581475765991, 0.9755282581475765991, 1.000000000000000000, 0.9510565162951535312, 1.000000000000000000, 0.9510565162951535312, 1.000000000000000000, 0.9510565162951535312, 1.000000000000000000, 0.9510565162951535312, 1.000000000000000000, 0.9755282581475765991, 0.9755282581475768211 ) ) 
 REPRESENTATION_ITEM ( '' )  );
#3511=CARTESIAN_POINT ( 'NONE',  ( -30.90169943749473802, 26.29999999999999716, 42.53254041760200721 ) ) ;
#3519=CARTESIAN_POINT ( 'NONE',  ( 40.34137639590981905, 32.65937500034139873, 29.30972558990010768 ) ) ;
#3521=CARTESIAN_POINT ( 'NONE',  ( -49.99999999999999289, 49.68125000068279462, -16.24598481164531449 ) ) ;
#3522=DIRECTION ( 'NONE',  ( -0.000000000000000000, -1.000000000000000000, -0.000000000000000000 ) ) ;
#3530=CARTESIAN_POINT ( 'NONE',  ( -15.40903463028480580, 36.32187500034140015, 47.42413220539094709 ) ) ;
#3534=CARTESIAN_POINT ( 'NONE',  ( 49.86468353125000164, 42.85937500034140157, -6.106662507704105588E-15 ) ) ;
#3537=CARTESIAN_POINT ( 'NONE',  ( -3.219174618344376363E-15, 27.28125000068279249, -52.57311121191334990 ) ) ;
#3543=CARTESIAN_POINT ( 'NONE',  ( -30.81806926056962226, 24.22187500034139163, 42.41743335407647919 ) ) ;
#3550=CARTESIAN_POINT ( 'NONE',  ( -49.86468353124999453, 36.02187500034139589, 16.20201782572377525 ) ) ;
#3551=CARTESIAN_POINT ( 'NONE',  ( -30.90169943749473447, 32.08125000068280031, 42.53254041760200721 ) ) ;
#3558=FACE_OUTER_BOUND ( 'NONE', #1478, .T. ) ;
#3562=CARTESIAN_POINT ( 'NONE',  ( 40.45084971874737079, 25.19999999999999929, -29.38926261462366440 ) ) ;
#3570=CARTESIAN_POINT ( 'NONE',  ( -49.86468353124999453, 25.95937500034139944, 16.20201782572377525 ) ) ;
#3571=CARTESIAN_POINT ( 'NONE',  ( 8.446640517145639571E-15, 48.28125000068279604, 50.00000000000000000 ) ) ;
#3575=CARTESIAN_POINT ( 'NONE',  ( -15.45084971874736368, 40.18125000068280173, 47.55282581475768211 ) ) ;
#3579=CARTESIAN_POINT ( 'NONE',  ( -40.45084971874737789, 27.58125000068280031, -29.38926261462365730 ) ) ;
#3582=CARTESIAN_POINT ( 'NONE',  ( 0.000000000000000000, 272.0000000000000000, 0.000000000000000000 ) ) ;
#3586=CARTESIAN_POINT ( 'NONE',  ( 30.90169943749475223, 36.48125000068279888, 42.53254041760199300 ) ) ;
#3591=CARTESIAN_POINT ( 'NONE',  ( 50.00000000000000711, 28.89999999999999858, 16.24598481164530739 ) ) ;
#3593=CARTESIAN_POINT ( 'NONE',  ( 7.513064459987437071E-14, 42.50000000000000000, 50.00000000000000000 ) ) ;
#3594=CARTESIAN_POINT ( 'NONE',  ( 30.81806926056964002, 46.55937500034139020, 42.41743335407647209 ) ) ;
#3595=ORIENTED_EDGE ( 'NONE', *, *, #2982, .T. ) ;
#3599=CARTESIAN_POINT ( 'NONE',  ( 30.81806926056964002, 36.55937500034139731, 42.41743335407647209 ) ) ;
#3600=CIRCLE ( 'NONE', #1192, 79.49773270518484480 ) ;
#3601=CARTESIAN_POINT ( 'NONE',  ( 30.90169943749475223, 40.48125000068279888, 42.53254041760199300 ) ) ;
#3604=CARTESIAN_POINT ( 'NONE',  ( 0.000000000000000000, 52.26146722824297797, 62.01141590572476758 ) ) ;
#3614=CARTESIAN_POINT ( 'NONE',  ( -40.34137639590981195, 36.12187500034139731, 29.30972558990012189 ) ) ;
#3619=CARTESIAN_POINT ( 'NONE',  ( 49.86468353125001585, 40.75937500034138594, 16.20201782572375038 ) ) ;
#3622=CARTESIAN_POINT ( 'NONE',  ( 50.00000000000000711, 26.68125000068279462, 16.24598481164530739 ) ) ;
#3623=DIRECTION ( 'NONE',  ( 0.000000000000000000, 1.000000000000000000, 0.000000000000000000 ) ) ;
#3628=CARTESIAN_POINT ( 'NONE',  ( -40.45084971874737789, 35.79999999999999716, -29.38926261462365730 ) ) ;
#3632=EDGE_CURVE ( 'NONE', #436, #11764, #1979, .T. ) ;
#3633=CARTESIAN_POINT ( 'NONE',  ( 15.40903463028481113, 21.32187500034139660, -47.42413220539094709 ) ) ;
#3634=EDGE_CURVE ( 'NONE', #11764, #8121, #4104, .T. ) ;
#3641=CARTESIAN_POINT ( 'NONE',  ( 49.86468353125000164, 34.92187500034140157, -6.106662507704105588E-15 ) ) ;
#3642=CARTESIAN_POINT ( 'NONE',  ( -30.90169943749474513, 41.48125000068279178, -42.53254041760200721 ) ) ;
#3644=VERTEX_POINT ( 'NONE', #61 ) ;
#3649=VECTOR ( 'NONE', #15870, 1000.000000000000000 ) ;
#3653=CYLINDRICAL_SURFACE ( 'NONE', #5764, 42.00000000000000711 ) ;
#3655=CARTESIAN_POINT ( 'NONE',  ( -7.919222016226816763, 35.33250428222964246, -49.99999999999999289 ) ) ;
#3658=CARTESIAN_POINT ( 'NONE',  ( 49.86468353125001585, 26.75937500034139660, 16.20201782572375038 ) ) ;
#3662=CARTESIAN_POINT ( 'NONE',  ( 50.00000000000000000, 34.78125000068280315, -6.123233995736766085E-15 ) ) ;
#3664=DIRECTION ( 'NONE',  ( -0.000000000000000000, -1.000000000000000000, -0.000000000000000000 ) ) ;
#3670=FACE_OUTER_BOUND ( 'NONE', #12240, .T. ) ;
#3678=CARTESIAN_POINT ( 'NONE',  ( 15.45084971874736723, 31.39999999999999858, -47.55282581475768211 ) ) ;
#3683=CARTESIAN_POINT ( 'NONE',  ( -30.81806926056963292, 43.55937500034139731, -42.41743335407647209 ) ) ;
#3689=CARTESIAN_POINT ( 'NONE',  ( 40.34137639590981195, 35.05937500034139731, -29.30972558990011834 ) ) ;
#3692=CARTESIAN_POINT ( 'NONE',  ( 46.91068958262674471, 25.00000000000000711, -16.90862634959390931 ) ) ;
#3693=EDGE_CURVE ( 'NONE', #12352, #305, #15615, .T. ) ;
#3699=CARTESIAN_POINT ( 'NONE',  ( -3.111920190527341144E-15, 29.28125000068279604, -50.00000000000000000 ) ) ;
#3702=CARTESIAN_POINT ( 'NONE',  ( -40.34137639590981195, 30.12187500034139731, 29.30972558990012189 ) ) ;
#3705=CARTESIAN_POINT ( 'NONE',  ( 49.86468353125001585, 36.75937500034139305, 16.20201782572375038 ) ) ;
#3707=CARTESIAN_POINT ( 'NONE',  ( 30.90169943749474157, 25.08125000068279675, -42.53254041760200721 ) ) ;
#3711=CARTESIAN_POINT ( 'NONE',  ( -40.34137639590981905, 25.72187500034139518, -29.30972558990011478 ) ) ;
#3714=CARTESIAN_POINT ( 'NONE',  ( -40.45084971874737079, 48.20000000000000284, 29.38926261462367151 ) ) ;
#3718=DIRECTION ( 'NONE',  ( -0.000000000000000000, -1.000000000000000000, -0.000000000000000000 ) ) ;
#3719=CARTESIAN_POINT ( 'NONE',  ( -49.86468353125000164, 37.92187500034140157, 0.000000000000000000 ) ) ;
#3720=CARTESIAN_POINT ( 'NONE',  ( -40.45084971874737789, 31.58125000068280031, -29.38926261462365730 ) ) ;
#3730=CARTESIAN_POINT ( 'NONE',  ( -49.99999999999999289, 39.90000000000000568, -16.24598481164531449 ) ) ;
#3734=CARTESIAN_POINT ( 'NONE',  ( -49.86468353124999453, 23.75937500034140015, -16.20201782572375393 ) ) ;
#3736=CARTESIAN_POINT ( 'NONE',  ( 2.978552182361884590E-14, 47.28125000068279604, -50.00000000000000000 ) ) ;
#3741=CARTESIAN_POINT ( 'NONE',  ( 30.90169943749475223, 38.48125000068279888, 42.53254041760199300 ) ) ;
#3742=CARTESIAN_POINT ( 'NONE',  ( -2.547328955960238000E-13, 32.28125000068278894, 49.99999999999999289 ) ) ;
#3754=EDGE_CURVE ( 'NONE', #10886, #4817, #8133, .T. ) ;
#3756=CARTESIAN_POINT ( 'NONE',  ( -49.99999999999999289, 43.89999999999999858, -16.24598481164531449 ) ) ;
#3757=CARTESIAN_POINT ( 'NONE',  ( -49.86468353124999453, 41.75937500034139305, -16.20201782572375393 ) ) ;
#3762=CARTESIAN_POINT ( 'NONE',  ( -30.81806926056963292, 27.55937500034139376, -42.41743335407647209 ) ) ;
#3765=EDGE_CURVE ( 'NONE', #5291, #10026, #10627, .T. ) ;
#3766=CARTESIAN_POINT ( 'NONE',  ( 48.32661496269174961, 25.00000000000000000, -12.28922088333727558 ) ) ;
#3767=CARTESIAN_POINT ( 'NONE',  ( 30.81806926056964002, 32.62187500034140442, 42.41743335407646498 ) ) ;
#3776=CARTESIAN_POINT ( 'NONE',  ( 30.81806926056964002, 32.62187500034140442, 42.41743335407647209 ) ) ;
#3778=ORIENTED_EDGE ( 'NONE', *, *, #4233, .F. ) ;
#3780=CARTESIAN_POINT ( 'NONE',  ( -3.210462471511496205E-15, 35.35937500034140157, -52.43083105670540789 ) ) ;
#3784=CARTESIAN_POINT ( 'NONE',  ( 15.40903463028481113, 47.25937500034140015, -47.42413220539094709 ) ) ;
#3786=CARTESIAN_POINT ( 'NONE',  ( -49.86468353125000164, 21.92187500034139802, 0.000000000000000000 ) ) ;
#3790=CARTESIAN_POINT ( 'NONE',  ( -7.919222016226804328, 26.22999571913594963, 50.00000000000000000 ) ) ;
#3791=CARTESIAN_POINT ( 'NONE',  ( 50.00000000000000711, 48.90000000000000568, 16.24598481164530739 ) ) ;
#3793=ADVANCED_FACE ( 'NONE', ( #14281 ), #10711, .T. ) ;
#3795=CARTESIAN_POINT ( 'NONE',  ( -49.86468353125000164, 47.92187500034139447, 0.000000000000000000 ) ) ;
#3798=DIRECTION ( 'NONE',  ( 0.000000000000000000, 0.000000000000000000, -1.000000000000000000 ) ) ;
#3803=CARTESIAN_POINT ( 'NONE',  ( 7.919222016226791006, 44.55125428154683931, 50.00000000000000711 ) ) ;
#3805=CARTESIAN_POINT ( 'NONE',  ( 0.000000000000000000, 51.99999999999999289, 0.000000000000000000 ) ) ;
#3807=EDGE_CURVE ( 'NONE', #5010, #3492, #13281, .T. ) ;
#3808=FILL_AREA_STYLE_COLOUR ( '', #5324 ) ;
#3815=CARTESIAN_POINT ( 'NONE',  ( 9.631387414534489405E-15, 24.35937500034139802, 52.43083105670540789 ) ) ;
#3816=ORIENTED_EDGE ( 'NONE', *, *, #15445, .F. ) ;
#3817=DIRECTION ( 'NONE',  ( -0.000000000000000000, -1.000000000000000000, -0.000000000000000000 ) ) ;
#3833=CARTESIAN_POINT ( 'NONE',  ( -50.00000000000000000, 24.00000000000000000, 0.000000000000000000 ) ) ;
#3837=CARTESIAN_POINT ( 'NONE',  ( 49.86468353124999453, 40.95937500034140299, -16.20201782572376459 ) ) ;
#3840=( BOUNDED_CURVE ( )  B_SPLINE_CURVE ( 2, ( #5636, #4553, #4475, #13110, #4309, #1952, #9453, #3212, #1801, #2969, #15853, #13197, #8037 ),
 .UNSPECIFIED., .F., .F. ) 
 B_SPLINE_CURVE_WITH_KNOTS ( ( 3, 2, 2, 2, 2, 2, 3 ),
 ( 0.1166666666666666685, 0.1199999999999999956, 0.1266666666666666774, 0.1333333333333333315, 0.1400000000000000133, 0.1466666666666666674, 0.1499999999999999944 ),
 .UNSPECIFIED. ) 
 CURVE ( )  GEOMETRIC_REPRESENTATION_ITEM ( )  RATIONAL_B_SPLINE_CURVE ( ( 0.9755282581475768211, 0.9755282581475768211, 1.000000000000000000, 0.9510565162951535312, 1.000000000000000000, 0.9510565162951535312, 1.000000000000000000, 0.9510565162951535312, 1.000000000000000000, 0.9510565162951535312, 1.000000000000000000, 0.9755282581475768211, 0.9755282581475768211 ) ) 
 REPRESENTATION_ITEM ( '' )  );
#3841=CARTESIAN_POINT ( 'NONE',  ( 9.631387414534489405E-15, 26.35937500034140157, 52.43083105670540789 ) ) ;
#3842=VERTEX_POINT ( 'NONE', #1961 ) ;
#3843=CARTESIAN_POINT ( 'NONE',  ( 40.45084971874737079, 27.20000000000000284, -29.38926261462366440 ) ) ;
#3845=CARTESIAN_POINT ( 'NONE',  ( 48.28553921371819513, 25.00000000000000000, -12.45074877219152576 ) ) ;
#3846=CARTESIAN_POINT ( 'NONE',  ( 40.34137639590981905, 32.72187500034139873, 29.30972558990010768 ) ) ;
#3847=CIRCLE ( 'NONE', #13133, 50.00000000000000000 ) ;
#3848=CARTESIAN_POINT ( 'NONE',  ( 7.919222016226940219, 31.22999571913595673, -49.99999999999996447 ) ) ;
#3850=CARTESIAN_POINT ( 'NONE',  ( 9.735664389687646693E-15, 272.0000000000000000, 79.49773270518484480 ) ) ;
#3855=CARTESIAN_POINT ( 'NONE',  ( -15.40903463028481646, 29.52187500034139589, -47.42413220539093999 ) ) ;
#3860=CARTESIAN_POINT ( 'NONE',  ( 9.631387414534489405E-15, 34.35937500034140157, 52.43083105670540789 ) ) ;
#3862=ORIENTED_EDGE ( 'NONE', *, *, #12206, .F. ) ;
#3864=CARTESIAN_POINT ( 'NONE',  ( -15.40903463028480580, 48.25937500034140015, 47.42413220539094709 ) ) ;
#3865=CARTESIAN_POINT ( 'NONE',  ( -49.93234176562499727, 49.96093750017070079, 0.000000000000000000 ) ) ;
#3866=CARTESIAN_POINT ( 'NONE',  ( 30.81806926056962936, 21.22187500034139518, -42.41743335407647209 ) ) ;
#3870=AXIS2_PLACEMENT_3D ( 'NONE', #13443, #1882, #6975 ) ;
#3872=CARTESIAN_POINT ( 'NONE',  ( 50.00000000000000711, 44.90000000000000568, 16.24598481164530739 ) ) ;
#3900=CARTESIAN_POINT ( 'NONE',  ( -49.86468353125000164, 49.92187500034140157, 0.000000000000000000 ) ) ;
#3908=CARTESIAN_POINT ( 'NONE',  ( 50.00000000000000711, 28.89999999999999858, 16.24598481164530739 ) ) ;
#3912=CARTESIAN_POINT ( 'NONE',  ( -6.668400408272873429E-15, 49.28125000068279604, -50.00000000000000000 ) ) ;
#3920=CARTESIAN_POINT ( 'NONE',  ( 15.40903463028482356, 44.45937500034139589, 47.42413220539093999 ) ) ;
#3924=CARTESIAN_POINT ( 'NONE',  ( -15.40903463028481646, 29.45937500034139589, -47.42413220539093999 ) ) ;
#3926=EDGE_CURVE ( 'NONE', #2810, #15172, #9719, .T. ) ;
#3929=CARTESIAN_POINT ( 'NONE',  ( 48.15826639445412383, 25.00000000000000000, -12.93428853971252401 ) ) ;
#3930=CARTESIAN_POINT ( 'NONE',  ( 9.631387414534489405E-15, 32.42187500034139447, 52.43083105670540789 ) ) ;
#3931=CARTESIAN_POINT ( 'NONE',  ( 30.90169943749473802, 31.08125000068280031, -42.53254041760200721 ) ) ;
#3933=CARTESIAN_POINT ( 'NONE',  ( 40.45084971874737789, 42.80000000000000426, 29.38926261462365375 ) ) ;
#3938=CARTESIAN_POINT ( 'NONE',  ( 49.86468353124999453, 33.02187500034139589, -16.20201782572376459 ) ) ;
#3940=ORIENTED_EDGE ( 'NONE', *, *, #1818, .T. ) ;
#3943=CARTESIAN_POINT ( 'NONE',  ( 30.81806926056962936, 33.15937500034139873, -42.41743335407646498 ) ) ;
#3946=CARTESIAN_POINT ( 'NONE',  ( 9.631387414534489405E-15, 48.35937500034140157, 52.43083105670540789 ) ) ;
#3948=CARTESIAN_POINT ( 'NONE',  ( -15.40903463028480580, 22.32187500034139660, 47.42413220539094709 ) ) ;
#3953=CARTESIAN_POINT ( 'NONE',  ( -40.45084971874737079, 46.20000000000000284, 29.38926261462367151 ) ) ;
#3959=CARTESIAN_POINT ( 'NONE',  ( -49.99999999999999289, 39.68125000068280173, -16.24598481164531449 ) ) ;
#3962=CARTESIAN_POINT ( 'NONE',  ( -30.90169943749474513, 31.70000000000000639, -42.53254041760200721 ) ) ;
#3965=CARTESIAN_POINT ( 'NONE',  ( 30.81806926056962936, 47.22187500034139873, -42.41743335407646498 ) ) ;
#3973=CARTESIAN_POINT ( 'NONE',  ( 0.000000000000000000, 193.4213562373095385, 0.000000000000000000 ) ) ;
#3976=CARTESIAN_POINT ( 'NONE',  ( 50.00000000000000711, 28.68125000068279462, 16.24598481164530739 ) ) ;
#3978=CARTESIAN_POINT ( 'NONE',  ( 40.34137639590981905, 46.72187500034139873, 29.30972558990010768 ) ) ;
#3980=CARTESIAN_POINT ( 'NONE',  ( -7.919222016226816763, 25.55125428154684641, -49.99999999999999289 ) ) ;
#3982=EDGE_LOOP ( 'NONE', ( #11827, #985 ) ) ;
#3987=CARTESIAN_POINT ( 'NONE',  ( 40.45084971874737079, 29.19999999999999929, -29.38926261462366440 ) ) ;
#3997=ADVANCED_FACE ( 'NONE', ( #3558 ), #4899, .T. ) ;
#3998=CARTESIAN_POINT ( 'NONE',  ( -40.45084971874737079, 20.20000000000000284, 29.38926261462367151 ) ) ;
#4000=ORIENTED_EDGE ( 'NONE', *, *, #5282, .T. ) ;
#4001=CARTESIAN_POINT ( 'NONE',  ( 40.34137639590981905, 34.65937500034139873, 29.30972558990010768 ) ) ;
#4003=EDGE_CURVE ( 'NONE', #3234, #15272, #9864, .T. ) ;
#4006=CARTESIAN_POINT ( 'NONE',  ( -40.34137639590981195, 30.05937500034139731, 29.30972558990012189 ) ) ;
#4011=CARTESIAN_POINT ( 'NONE',  ( 46.31917516190732442, 25.00000000000000000, -18.46674513801128370 ) ) ;
#4012=CARTESIAN_POINT ( 'NONE',  ( 49.86468353125000164, 36.92187500034140157, -6.106662507704105588E-15 ) ) ;
#4021=CARTESIAN_POINT ( 'NONE',  ( -3.210462471511496205E-15, 31.42187500034139447, -52.43083105670540789 ) ) ;
#4023=CARTESIAN_POINT ( 'NONE',  ( -49.86468353124999453, 33.75937500034140015, -16.20201782572375393 ) ) ;
#4024=VERTEX_POINT ( 'NONE', #7305 ) ;
#4027=CARTESIAN_POINT ( 'NONE',  ( -3.210462471511496205E-15, 45.35937500034139447, -52.43083105670540789 ) ) ;
#4029=CARTESIAN_POINT ( 'NONE',  ( -15.40903463028480580, 26.32187500034140015, 47.42413220539094709 ) ) ;
#4033=CARTESIAN_POINT ( 'NONE',  ( -7.919222016226816763, 25.33250428222964246, -49.99999999999999289 ) ) ;
#4034=CARTESIAN_POINT ( 'NONE',  ( 50.00000000000000000, 45.00000000000000711, -6.123233995736766085E-15 ) ) ;
#4036=CARTESIAN_POINT ( 'NONE',  ( -49.86468353124999453, 49.82187500034140015, -16.20201782572375393 ) ) ;
#4042=CARTESIAN_POINT ( 'NONE',  ( -40.45084971874737789, 35.58125000068279320, -29.38926261462365730 ) ) ;
#4053=CYLINDRICAL_SURFACE ( 'NONE', #11528, 50.00000000000000000 ) ;
#4057=CARTESIAN_POINT ( 'NONE',  ( 15.40903463028481113, 47.32187500034140015, -47.42413220539094709 ) ) ;
#4071=CARTESIAN_POINT ( 'NONE',  ( 8.446640517145639571E-15, 48.49999999999999289, 50.00000000000000000 ) ) ;
#4078=CARTESIAN_POINT ( 'NONE',  ( 30.81806926056962936, 37.15937500034139873, -42.41743335407647209 ) ) ;
#4082=AXIS2_PLACEMENT_3D ( 'NONE', #7167, #13470, #5919 ) ;
#4085=CARTESIAN_POINT ( 'NONE',  ( 49.86468353125001585, 20.75937500034140015, 16.20201782572375038 ) ) ;
#4087=EDGE_CURVE ( 'NONE', #495, #4982, #7343, .T. ) ;
#4088=CARTESIAN_POINT ( 'NONE',  ( 50.00000000000000000, 27.00000000000000355, -6.123233995736766085E-15 ) ) ;
#4091=CARTESIAN_POINT ( 'NONE',  ( 30.81806926056962936, 37.22187500034139163, -42.41743335407646498 ) ) ;
#4097=VECTOR ( 'NONE', #12557, 1000.000000000000000 ) ;
#4100=CARTESIAN_POINT ( 'NONE',  ( -3.210462471511496205E-15, 27.42187500034139092, -52.43083105670540789 ) ) ;
#4104=( BOUNDED_CURVE ( )  B_SPLINE_CURVE ( 2, ( #14112, #14035, #1395, #11542, #1483, #4156, #14195, #5338, #5088, #6580, #10141, #6404, #7649 ),
 .UNSPECIFIED., .F., .T. ) 
 B_SPLINE_CURVE_WITH_KNOTS ( ( 3, 2, 2, 2, 2, 2, 3 ),
 ( 0.7166666666666666741, 0.7199999999999999734, 0.7266666666666666829, 0.7333333333333332815, 0.7399999999999999911, 0.7466666666666667007, 0.7500000000000000000 ),
 .UNSPECIFIED. ) 
 CURVE ( )  GEOMETRIC_REPRESENTATION_ITEM ( )  RATIONAL_B_SPLINE_CURVE ( ( 0.9755282581475768211, 0.9755282581475768211, 1.000000000000000000, 0.9510565162951535312, 1.000000000000000000, 0.9510565162951535312, 1.000000000000000000, 0.9510565162951535312, 1.000000000000000000, 0.9510565162951535312, 1.000000000000000000, 0.9755282581475768211, 0.9755282581475768211 ) ) 
 REPRESENTATION_ITEM ( '' )  );
#4105=CARTESIAN_POINT ( 'NONE',  ( -40.34137639590981195, 32.05937500034139731, 29.30972558990012189 ) ) ;
#4109=CARTESIAN_POINT ( 'NONE',  ( 9.657523855033129090E-15, 20.28125000068279959, 52.57311121191334990 ) ) ;
#4110=CIRCLE ( 'NONE', #15509, 82.49773270518484480 ) ;
#4118=CARTESIAN_POINT ( 'NONE',  ( 40.45084971874737079, 41.20000000000000284, -29.38926261462366440 ) ) ;
#4125=CARTESIAN_POINT ( 'NONE',  ( -49.99999999999999289, 39.88125000068279746, 16.24598481164533226 ) ) ;
#4132=CARTESIAN_POINT ( 'NONE',  ( -30.81806926056963292, 45.62187500034139020, -42.41743335407646498 ) ) ;
#4136=CARTESIAN_POINT ( 'NONE',  ( 0.000000000000000000, 193.4213562373095385, 0.000000000000000000 ) ) ;
#4137=( BOUNDED_CURVE ( )  B_SPLINE_CURVE ( 2, ( #8645, #2332, #7413, #12483, #11240, #6832, #5504, #11882, #2734, #14439, #4166, #10644, #4071 ),
 .UNSPECIFIED., .F., .F. ) 
 B_SPLINE_CURVE_WITH_KNOTS ( ( 3, 2, 2, 2, 2, 2, 3 ),
 ( 0.01666666666666666644, 0.02000000000000000042, 0.02666666666666666838, 0.03333333333333333287, 0.04000000000000000083, 0.04666666666666666879, 0.05000000000000000278 ),
 .UNSPECIFIED. ) 
 CURVE ( )  GEOMETRIC_REPRESENTATION_ITEM ( )  RATIONAL_B_SPLINE_CURVE ( ( 0.9755282581475768211, 0.9755282581475768211, 1.000000000000000000, 0.9510565162951535312, 1.000000000000000000, 0.9510565162951535312, 1.000000000000000000, 0.9510565162951535312, 1.000000000000000000, 0.9510565162951535312, 1.000000000000000000, 0.9755282581475768211, 0.9755282581475768211 ) ) 
 REPRESENTATION_ITEM ( '' )  );
#4140=CARTESIAN_POINT ( 'NONE',  ( 30.90169943749473802, 35.08125000068278609, -42.53254041760200721 ) ) ;
#4147=CARTESIAN_POINT ( 'NONE',  ( -40.34137639590981905, 47.72187500034139873, -29.30972558990011478 ) ) ;
#4154=CARTESIAN_POINT ( 'NONE',  ( 6.123233995736766085E-15, 193.4213562373095385, 50.00000000000000000 ) ) ;
#4156=CARTESIAN_POINT ( 'NONE',  ( -49.99999999999999289, 28.10000000000000497, 16.24598481164533226 ) ) ;
#4162=CARTESIAN_POINT ( 'NONE',  ( 1.010305842943185372E-14, 252.0000000000000000, -82.49773270518484480 ) ) ;
#4164=CARTESIAN_POINT ( 'NONE',  ( -2.445080149700054274E-14, 46.50000000000000711, 50.00000000000000000 ) ) ;
#4166=CARTESIAN_POINT ( 'NONE',  ( 15.45084971874737789, 48.60000000000000142, 47.55282581475767500 ) ) ;
#4171=ORIENTED_EDGE ( 'NONE', *, *, #9269, .F. ) ;
#4172=CARTESIAN_POINT ( 'NONE',  ( 15.40903463028481113, 35.25937500034139305, -47.42413220539094709 ) ) ;
#4177=CARTESIAN_POINT ( 'NONE',  ( 50.00000000000000711, 48.68125000068279462, 16.24598481164530739 ) ) ;
#4185=CARTESIAN_POINT ( 'NONE',  ( 15.40903463028482356, 28.52187500034139589, 47.42413220539093999 ) ) ;
#4194=CARTESIAN_POINT ( 'NONE',  ( 9.657523855033129090E-15, 34.50000000000000711, 52.57311121191334990 ) ) ;
#4199=CARTESIAN_POINT ( 'NONE',  ( 30.81806926056964002, 32.55937500034139731, 42.41743335407646498 ) ) ;
#4202=CARTESIAN_POINT ( 'NONE',  ( -40.34137639590981905, 41.65937500034139873, -29.30972558990011478 ) ) ;
#4203=EDGE_CURVE ( 'NONE', #13411, #7884, #10541, .T. ) ;
#4210=CARTESIAN_POINT ( 'NONE',  ( -15.45084971874736368, 42.39999999999999858, 47.55282581475768211 ) ) ;
#4212=CARTESIAN_POINT ( 'NONE',  ( -30.81806926056962226, 46.22187500034139163, 42.41743335407647919 ) ) ;
#4216=CARTESIAN_POINT ( 'NONE',  ( 15.45084971874736723, 29.18125000068279817, -47.55282581475768211 ) ) ;
#4222=CARTESIAN_POINT ( 'NONE',  ( 9.631387414534489405E-15, 48.42187500034139447, 52.43083105670540789 ) ) ;
#4224=CARTESIAN_POINT ( 'NONE',  ( -15.45084971874737256, 39.38125000068279746, -47.55282581475767500 ) ) ;
#4227=CARTESIAN_POINT ( 'NONE',  ( 49.99999999999999289, 34.88125000068280457, -16.24598481164532160 ) ) ;
#4232=CARTESIAN_POINT ( 'NONE',  ( 49.86468353125000164, 20.85937500034139802, -6.106662507704105588E-15 ) ) ;
#4233=EDGE_CURVE ( 'NONE', #10949, #3473, #15054, .T. ) ;
#4245=DIRECTION ( 'NONE',  ( -0.000000000000000000, -1.000000000000000000, -0.000000000000000000 ) ) ;
#4250=CARTESIAN_POINT ( 'NONE',  ( -30.90169943749473447, 38.08125000068280031, 42.53254041760200721 ) ) ;
#4254=CARTESIAN_POINT ( 'NONE',  ( 49.86468353125000164, 34.85937500034140157, -6.106662507704105588E-15 ) ) ;
#4260=CARTESIAN_POINT ( 'NONE',  ( -3.210462471511496205E-15, 25.35937500034139802, -52.43083105670540789 ) ) ;
#4262=CARTESIAN_POINT ( 'NONE',  ( 49.99999999999999289, 35.10000000000000853, -16.24598481164532160 ) ) ;
#4263=CARTESIAN_POINT ( 'NONE',  ( 0.000000000000000000, 193.4213562373095385, -47.00000000000000000 ) ) ;
#4264=CARTESIAN_POINT ( 'NONE',  ( -15.40903463028481646, 27.52187500034139944, -47.42413220539093999 ) ) ;
#4267=EDGE_CURVE ( 'NONE', #1767, #15481, #10774, .T. ) ;
#4272=CARTESIAN_POINT ( 'NONE',  ( -30.90169943749473802, 34.29999999999998295, 42.53254041760200721 ) ) ;
#4276=CARTESIAN_POINT ( 'NONE',  ( 40.34137639590981905, 32.65937500034139873, 29.30972558990010768 ) ) ;
#4281=CARTESIAN_POINT ( 'NONE',  ( 9.631387414534489405E-15, 40.35937500034139447, 52.43083105670540789 ) ) ;
#4283=FACE_BOUND ( 'NONE', #15883, .T. ) ;
#4289=CARTESIAN_POINT ( 'NONE',  ( 30.90169943749474157, 41.30000000000001137, -42.53254041760200721 ) ) ;
#4291=CARTESIAN_POINT ( 'NONE',  ( 40.34137639590981905, 42.72187500034139873, 29.30972558990010768 ) ) ;
#4295=ORIENTED_EDGE ( 'NONE', *, *, #657, .T. ) ;
#4296=CARTESIAN_POINT ( 'NONE',  ( -3.219174618344376363E-15, 31.28125000068279604, -52.57311121191334990 ) ) ;
#4303=CARTESIAN_POINT ( 'NONE',  ( 49.86468353125000164, 46.92187500034139447, -6.106662507704105588E-15 ) ) ;
#4309=CARTESIAN_POINT ( 'NONE',  ( -40.45084971874737079, 45.98125000068279888, 29.38926261462367151 ) ) ;
#4311=CARTESIAN_POINT ( 'NONE',  ( 49.86468353124999453, 41.02187500034139589, -16.20201782572376459 ) ) ;
#4323=FACE_OUTER_BOUND ( 'NONE', #5068, .T. ) ;
#4331=CARTESIAN_POINT ( 'NONE',  ( -49.86468353124999453, 37.75937500034140015, -16.20201782572375393 ) ) ;
#4335=CARTESIAN_POINT ( 'NONE',  ( -30.90169943749474868, 49.48125000068279178, -42.53254041760200721 ) ) ;
#4336=EDGE_CURVE ( 'NONE', #1001, #11210, #12057, .T. ) ;
#4338=CARTESIAN_POINT ( 'NONE',  ( 49.86468353125001585, 22.75937500034139660, 16.20201782572375038 ) ) ;
#4344=CARTESIAN_POINT ( 'NONE',  ( 49.86468353125001585, 30.82187500034139660, 16.20201782572375038 ) ) ;
#4348=DIRECTION ( 'NONE',  ( -0.000000000000000000, -1.000000000000000000, -0.000000000000000000 ) ) ;
#4351=CARTESIAN_POINT ( 'NONE',  ( 50.00000000000000000, 33.00000000000000000, -6.123233995736766085E-15 ) ) ;
#4356=CARTESIAN_POINT ( 'NONE',  ( 40.34137639590981905, 28.65937500034139873, 29.30972558990010768 ) ) ;
#4357=ORIENTED_EDGE ( 'NONE', *, *, #626, .T. ) ;
#4359=CARTESIAN_POINT ( 'NONE',  ( 30.81806926056964002, 40.55937500034139731, 42.41743335407647209 ) ) ;
#4366=CARTESIAN_POINT ( 'NONE',  ( -15.40903463028481646, 29.52187500034139589, -47.42413220539093999 ) ) ;
#4367=CARTESIAN_POINT ( 'NONE',  ( 50.00000000000000711, 40.89999999999999858, 16.24598481164530739 ) ) ;
#4369=CARTESIAN_POINT ( 'NONE',  ( 15.40903463028482356, 46.52187500034139589, 47.42413220539093999 ) ) ;
#4372=CARTESIAN_POINT ( 'NONE',  ( -30.81806926056962226, 48.15937500034139873, 42.41743335407647209 ) ) ;
#4374=CARTESIAN_POINT ( 'NONE',  ( 50.00000000000000711, 32.68125000068279462, 16.24598481164530739 ) ) ;
#4376=CARTESIAN_POINT ( 'NONE',  ( -7.919222016226818539, 49.33250428222964956, -49.99999999999999289 ) ) ;
#4380=CARTESIAN_POINT ( 'NONE',  ( 9.631387414534489405E-15, 40.42187500034138736, 52.43083105670540789 ) ) ;
#4383=VECTOR ( 'NONE', #4923, 1000.000000000000000 ) ;
#4390=CARTESIAN_POINT ( 'NONE',  ( -40.34137639590981195, 44.12187500034139731, 29.30972558990012189 ) ) ;
#4395=DIRECTION ( 'NONE',  ( 0.000000000000000000, 1.000000000000000000, 0.000000000000000000 ) ) ;
#4402=FACE_OUTER_BOUND ( 'NONE', #3434, .T. ) ;
#4405=LINE ( 'NONE', #7226, #3649 ) ;
#4409=ORIENTED_EDGE ( 'NONE', *, *, #3632, .T. ) ;
#4410=CARTESIAN_POINT ( 'NONE',  ( 40.34137639590981195, 29.05937500034139376, -29.30972558990011834 ) ) ;
#4419=CARTESIAN_POINT ( 'NONE',  ( 15.40903463028481113, 21.25937500034139660, -47.42413220539094709 ) ) ;
#4424=CARTESIAN_POINT ( 'NONE',  ( -50.00000000000000000, 49.78125000068280315, 0.000000000000000000 ) ) ;
#4428=CARTESIAN_POINT ( 'NONE',  ( -15.40903463028480580, 30.32187500034140015, 47.42413220539094709 ) ) ;
#4431=CARTESIAN_POINT ( 'NONE',  ( 0.000000000000000000, 272.0000000000000000, 0.000000000000000000 ) ) ;
#4434=CARTESIAN_POINT ( 'NONE',  ( -30.90169943749474868, 33.69999999999998863, -42.53254041760200721 ) ) ;
#4440=EDGE_LOOP ( 'NONE', ( #13781, #2936, #8530, #15266 ) ) ;
#4442=CARTESIAN_POINT ( 'NONE',  ( -30.81806926056963292, 31.55937500034139376, -42.41743335407646498 ) ) ;
#4444=ORIENTED_EDGE ( 'NONE', *, *, #5655, .F. ) ;
#4445=CYLINDRICAL_SURFACE ( 'NONE', #14482, 50.00000000000000000 ) ;
#4446=CARTESIAN_POINT ( 'NONE',  ( 15.40903463028481113, 39.25937500034140015, -47.42413220539094709 ) ) ;
#4449=CARTESIAN_POINT ( 'NONE',  ( -40.34137639590981195, 20.12187500034139731, 29.30972558990012189 ) ) ;
#4455=CARTESIAN_POINT ( 'NONE',  ( 40.34137639590981905, 28.72187500034139873, 29.30972558990010768 ) ) ;
#4456=CARTESIAN_POINT ( 'NONE',  ( 49.99999999999999289, 43.10000000000000142, -16.24598481164532160 ) ) ;
#4458=CARTESIAN_POINT ( 'NONE',  ( -49.86468353124999453, 45.82187500034140015, -16.20201782572375393 ) ) ;
#4461=CARTESIAN_POINT ( 'NONE',  ( -40.34137639590981905, 49.65937500034139873, -29.30972558990011478 ) ) ;
#4463=ORIENTED_EDGE ( 'NONE', *, *, #7428, .F. ) ;
#4464=CARTESIAN_POINT ( 'NONE',  ( 9.657523855033129090E-15, 32.28125000068279604, 52.57311121191334990 ) ) ;
#4467=CARTESIAN_POINT ( 'NONE',  ( 15.45084971874737789, 32.38125000068280457, 47.55282581475767500 ) ) ;
#4468=CARTESIAN_POINT ( 'NONE',  ( -49.86468353124999453, 37.82187500034139305, -16.20201782572375393 ) ) ;
#4471=ADVANCED_FACE ( 'NONE', ( #5301 ), #16343, .T. ) ;
#4475=CARTESIAN_POINT ( 'NONE',  ( -15.45084971874736368, 46.18125000068280173, 47.55282581475768211 ) ) ;
#4476=VERTEX_POINT ( 'NONE', #10274 ) ;
#4477=CARTESIAN_POINT ( 'NONE',  ( -40.34137639590981195, 40.12187500034139731, 29.30972558990012189 ) ) ;
#4483=DIRECTION ( 'NONE',  ( 0.000000000000000000, 0.000000000000000000, -1.000000000000000000 ) ) ;
#4489=CARTESIAN_POINT ( 'NONE',  ( -40.45084971874737079, 33.98125000068279888, 29.38926261462367151 ) ) ;
#4494=CARTESIAN_POINT ( 'NONE',  ( 7.919222016226854954, 42.33250428222964246, 49.99999999999998579 ) ) ;
#4498=CARTESIAN_POINT ( 'NONE',  ( -15.40903463028481646, 33.45937500034139589, -47.42413220539093999 ) ) ;
#4501=ORIENTED_EDGE ( 'NONE', *, *, #6710, .F. ) ;
#4502=CARTESIAN_POINT ( 'NONE',  ( -49.99999999999999289, 43.88125000068279746, 16.24598481164533226 ) ) ;
#4505=CARTESIAN_POINT ( 'NONE',  ( 0.000000000000000000, 52.26146722824297797, 0.000000000000000000 ) ) ;
#4519=CARTESIAN_POINT ( 'NONE',  ( -40.45084971874737789, 33.80000000000000426, -29.38926261462365730 ) ) ;
#4522=CARTESIAN_POINT ( 'NONE',  ( -49.86468353125000164, 49.85937500034139447, 0.000000000000000000 ) ) ;
#4524=CARTESIAN_POINT ( 'NONE',  ( 45.11452830843730766, 25.00000000000000355, -21.24066852005663719 ) ) ;
#4527=CARTESIAN_POINT ( 'NONE',  ( 40.34137639590981905, 38.65937500034139873, 29.30972558990010768 ) ) ;
#4534=CARTESIAN_POINT ( 'NONE',  ( -40.34137639590981195, 32.12187500034140442, 29.30972558990012189 ) ) ;
#4537=CARTESIAN_POINT ( 'NONE',  ( -15.40903463028481646, 45.52187500034139589, -47.42413220539093999 ) ) ;
#4539=ORIENTED_EDGE ( 'NONE', *, *, #2349, .F. ) ;
#4540=CARTESIAN_POINT ( 'NONE',  ( -40.34137639590981195, 48.05937500034139731, 29.30972558990012189 ) ) ;
#4543=CARTESIAN_POINT ( 'NONE',  ( -40.45084971874737079, 33.98125000068279888, 29.38926261462367151 ) ) ;
#4546=CARTESIAN_POINT ( 'NONE',  ( 30.81806926056964002, 40.62187500034139731, 42.41743335407646498 ) ) ;
#4549=CARTESIAN_POINT ( 'NONE',  ( -40.34137639590981195, 22.12187500034139731, 29.30972558990012189 ) ) ;
#4553=CARTESIAN_POINT ( 'NONE',  ( -7.919222016226822092, 46.22999571913594963, 50.00000000000000000 ) ) ;
#4555=CARTESIAN_POINT ( 'NONE',  ( 15.40903463028481113, 39.32187500034140015, -47.42413220539094709 ) ) ;
#4559=FACE_OUTER_BOUND ( 'NONE', #12107, .T. ) ;
#4570=CARTESIAN_POINT ( 'NONE',  ( 7.919222016226758143, 36.55125428154683931, 50.00000000000000711 ) ) ;
#4573=CARTESIAN_POINT ( 'NONE',  ( -40.34137639590981195, 28.05937500034139731, 29.30972558990012189 ) ) ;
#4574=ORIENTED_EDGE ( 'NONE', *, *, #13150, .T. ) ;
#4576=ORIENTED_EDGE ( 'NONE', *, *, #204, .T. ) ;
#4577=CARTESIAN_POINT ( 'NONE',  ( 40.45084971874737789, 42.58125000068280031, 29.38926261462365375 ) ) ;
#4578=CARTESIAN_POINT ( 'NONE',  ( -49.86468353125000164, 49.92187500034140157, 0.000000000000000000 ) ) ;
#4580=VERTEX_POINT ( 'NONE', #12685 ) ;
#4593=CARTESIAN_POINT ( 'NONE',  ( 50.00000000000000000, 27.00000000000000355, -6.123233995736766085E-15 ) ) ;
#4605=CARTESIAN_POINT ( 'NONE',  ( -15.40903463028481646, 33.45937500034139589, -47.42413220539093999 ) ) ;
#4612=CARTESIAN_POINT ( 'NONE',  ( 49.86468353125001585, 28.82187500034139305, 16.20201782572375038 ) ) ;
#4614=CIRCLE ( 'NONE', #6994, 2.000000000000001776 ) ;
#4616=CARTESIAN_POINT ( 'NONE',  ( 49.86468353124999453, 35.02187500034139589, -16.20201782572376459 ) ) ;
#4620=CARTESIAN_POINT ( 'NONE',  ( -15.40903463028481646, 45.45937500034139589, -47.42413220539093999 ) ) ;
#4623=CARTESIAN_POINT ( 'NONE',  ( -15.45084971874737256, 27.38125000068280102, -47.55282581475767500 ) ) ;
#4627=CARTESIAN_POINT ( 'NONE',  ( 49.86468353125001585, 42.82187500034139305, 16.20201782572375038 ) ) ;
#4630=CARTESIAN_POINT ( 'NONE',  ( 40.34137639590981905, 22.72187500034139518, 29.30972558990010768 ) ) ;
#4637=CARTESIAN_POINT ( 'NONE',  ( 30.81806926056964002, 42.62187500034139731, 42.41743335407647209 ) ) ;
#4638=CARTESIAN_POINT ( 'NONE',  ( -49.99999999999999289, 41.68125000068280173, -16.24598481164531449 ) ) ;
#4640=ORIENTED_EDGE ( 'NONE', *, *, #14631, .T. ) ;
#4655=CARTESIAN_POINT ( 'NONE',  ( -2.547328955960238000E-13, 34.50000000000000000, 49.99999999999999289 ) ) ;
#4659=CARTESIAN_POINT ( 'NONE',  ( 40.34137639590981195, 31.05937500034139731, -29.30972558990011834 ) ) ;
#4663=CARTESIAN_POINT ( 'NONE',  ( -40.45084971874737789, 43.58125000068280031, -29.38926261462365730 ) ) ;
#4668=CARTESIAN_POINT ( 'NONE',  ( 8.446640517145639571E-15, 28.28125000068279959, 50.00000000000000000 ) ) ;
#4675=CARTESIAN_POINT ( 'NONE',  ( 49.99999999999999289, 36.88125000068279036, -16.24598481164532160 ) ) ;
#4682=CARTESIAN_POINT ( 'NONE',  ( 15.45084971874737789, 30.60000000000000142, 47.55282581475767500 ) ) ;
#4686=ORIENTED_EDGE ( 'NONE', *, *, #4087, .F. ) ;
#4689=CARTESIAN_POINT ( 'NONE',  ( -30.81806926056963292, 25.55937500034139376, -42.41743335407646498 ) ) ;
#4691=LINE ( 'NONE', #15133, #16373 ) ;
#4692=CARTESIAN_POINT ( 'NONE',  ( 40.34137639590981905, 36.65937500034139873, 29.30972558990010768 ) ) ;
#4693=CARTESIAN_POINT ( 'NONE',  ( 50.00000000000000000, 40.78125000068279604, -6.123233995736766085E-15 ) ) ;
#4701=AXIS2_PLACEMENT_3D ( 'NONE', #7750, #8667, #10168 ) ;
#4702=AXIS2_PLACEMENT_3D ( 'NONE', #8053, #1966, #13365 ) ;
#4704=CARTESIAN_POINT ( 'NONE',  ( -15.40903463028480580, 28.32187500034139660, 47.42413220539094709 ) ) ;
#4706=CARTESIAN_POINT ( 'NONE',  ( 50.00000000000000711, 32.89999999999999858, 16.24598481164530739 ) ) ;
#4709=CARTESIAN_POINT ( 'NONE',  ( -49.86468353124999453, 37.82187500034139305, -16.20201782572375393 ) ) ;
#4714=CARTESIAN_POINT ( 'NONE',  ( -40.34137639590981905, 43.65937500034139163, -29.30972558990011478 ) ) ;
#4720=CARTESIAN_POINT ( 'NONE',  ( 40.45084971874737079, 26.98125000068279888, -29.38926261462366440 ) ) ;
#4722=CARTESIAN_POINT ( 'NONE',  ( -7.919222016226816763, 35.55125428154684641, -49.99999999999999289 ) ) ;
#4723=CARTESIAN_POINT ( 'NONE',  ( 40.34137639590981905, 38.72187500034139873, 29.30972558990010768 ) ) ;
#4725=CARTESIAN_POINT ( 'NONE',  ( 50.00000000000000000, 41.00000000000000000, -6.123233995736766085E-15 ) ) ;
#4726=CARTESIAN_POINT ( 'NONE',  ( 49.86468353125001585, 20.82187500034140015, 16.20201782572375038 ) ) ;
#4734=ADVANCED_FACE ( 'NONE', ( #7109 ), #7019, .T. ) ;
#4735=CARTESIAN_POINT ( 'NONE',  ( 30.81806926056964002, 34.62187500034139731, 42.41743335407647209 ) ) ;
#4739=ORIENTED_EDGE ( 'NONE', *, *, #5282, .F. ) ;
#4750=CARTESIAN_POINT ( 'NONE',  ( -7.919222016226934890, 34.44874571845316069, 49.99999999999996447 ) ) ;
#4754=CARTESIAN_POINT ( 'NONE',  ( 15.40903463028482356, 30.45937500034139589, 47.42413220539093999 ) ) ;
#4757=ORIENTED_EDGE ( 'NONE', *, *, #3754, .F. ) ;
#4758=CARTESIAN_POINT ( 'NONE',  ( 49.99999999999999289, 42.88125000068278325, -16.24598481164532160 ) ) ;
#4763=CARTESIAN_POINT ( 'NONE',  ( -50.00000000000000000, 27.78125000068279959, 0.000000000000000000 ) ) ;
#4773=CARTESIAN_POINT ( 'NONE',  ( 9.657523855033129090E-15, 26.50000000000000355, 52.57311121191334990 ) ) ;
#4775=CARTESIAN_POINT ( 'NONE',  ( -40.45084971874737789, 43.80000000000000426, -29.38926261462365730 ) ) ;
#4781=CARTESIAN_POINT ( 'NONE',  ( 49.86468353125001585, 36.75937500034138594, 16.20201782572375038 ) ) ;
#4795=CARTESIAN_POINT ( 'NONE',  ( 30.81806926056962936, 37.22187500034139873, -42.41743335407647209 ) ) ;
#4801=CARTESIAN_POINT ( 'NONE',  ( -30.81806926056963292, 41.55937500034139731, -42.41743335407646498 ) ) ;
#4803=CARTESIAN_POINT ( 'NONE',  ( -30.90169943749474868, 23.48125000068279888, -42.53254041760200721 ) ) ;
#4804=ORIENTED_EDGE ( 'NONE', *, *, #3372, .T. ) ;
#4806=CARTESIAN_POINT ( 'NONE',  ( -49.86468353124999453, 36.02187500034139589, 16.20201782572377169 ) ) ;
#4808=CARTESIAN_POINT ( 'NONE',  ( 15.45084971874736723, 31.39999999999999858, -47.55282581475768211 ) ) ;
#4810=CARTESIAN_POINT ( 'NONE',  ( 49.86468353124999453, 25.02187500034139589, -16.20201782572376459 ) ) ;
#4815=CARTESIAN_POINT ( 'NONE',  ( -49.86468353124999453, 35.82187500034139305, -16.20201782572375393 ) ) ;
#4816=CARTESIAN_POINT ( 'NONE',  ( -15.45084971874737256, 43.38125000068279746, -47.55282581475767500 ) ) ;
#4817=VERTEX_POINT ( 'NONE', #12164 ) ;
#4819=EDGE_CURVE ( 'NONE', #15674, #12352, #15456, .T. ) ;
#4829=CARTESIAN_POINT ( 'NONE',  ( -50.00000000000000000, 40.00000000000000000, 0.000000000000000000 ) ) ;
#4830=CARTESIAN_POINT ( 'NONE',  ( 7.919222016226809657, 43.22999571913594963, -50.00000000000000000 ) ) ;
#4832=CARTESIAN_POINT ( 'NONE',  ( -40.34137639590981195, 26.05937500034139731, 29.30972558990012189 ) ) ;
#4836=ADVANCED_FACE ( 'NONE', ( #5776 ), #14721, .T. ) ;
#4838=CARTESIAN_POINT ( 'NONE',  ( 50.00000000000000711, 40.68125000068280173, 16.24598481164530739 ) ) ;
#4843=CARTESIAN_POINT ( 'NONE',  ( -40.45084971874737079, 27.98125000068279888, 29.38926261462367151 ) ) ;
#4846=CARTESIAN_POINT ( 'NONE',  ( 49.99999999999999289, 26.88125000068280102, -16.24598481164532160 ) ) ;
#4848=CARTESIAN_POINT ( 'NONE',  ( 0.000000000000000000, 193.4213562373095385, 0.000000000000000000 ) ) ;
#4853=CARTESIAN_POINT ( 'NONE',  ( -30.90169943749474868, 29.70000000000000284, -42.53254041760200721 ) ) ;
#4857=CARTESIAN_POINT ( 'NONE',  ( 15.40903463028481113, 45.25937500034140015, -47.42413220539094709 ) ) ;
#4863=CARTESIAN_POINT ( 'NONE',  ( 9.631387414534489405E-15, 36.35937500034140157, 52.43083105670540789 ) ) ;
#4868=CARTESIAN_POINT ( 'NONE',  ( 15.45084971874737789, 44.38125000068279746, 47.55282581475767500 ) ) ;
#4875=CARTESIAN_POINT ( 'NONE',  ( 30.81806926056964002, 38.62187500034139731, 42.41743335407647209 ) ) ;
#4878=CARTESIAN_POINT ( 'NONE',  ( 49.86468353125000164, 44.85937500034140157, -6.106662507704105588E-15 ) ) ;
#4880=CARTESIAN_POINT ( 'NONE',  ( 30.90169943749474157, 23.08125000068279320, -42.53254041760200721 ) ) ;
#4884=CARTESIAN_POINT ( 'NONE',  ( -7.919222016226870942, 36.44874571845315359, 49.99999999999997158 ) ) ;
#4887=CARTESIAN_POINT ( 'NONE',  ( 40.34137639590981195, 21.12187500034139376, -29.30972558990011834 ) ) ;
#4891=CARTESIAN_POINT ( 'NONE',  ( 49.86468353124999453, 35.02187500034139589, -16.20201782572376459 ) ) ;
#4892=CARTESIAN_POINT ( 'NONE',  ( -2.547328955960238000E-13, 32.28125000068278894, 49.99999999999999289 ) ) ;
#4895=ADVANCED_FACE ( 'NONE', ( #6183 ), #14978, .T. ) ;
#4899=CYLINDRICAL_SURFACE ( 'NONE', #2278, 50.00000000000000000 ) ;
#4910=DIRECTION ( 'NONE',  ( 0.000000000000000000, 1.000000000000000000, 0.000000000000000000 ) ) ;
#4911=CARTESIAN_POINT ( 'NONE',  ( -40.45084971874737789, 35.58125000068279320, -29.38926261462365730 ) ) ;
#4915=CARTESIAN_POINT ( 'NONE',  ( -49.86468353125000164, 25.85937500034139802, 0.000000000000000000 ) ) ;
#4918=ORIENTED_EDGE ( 'NONE', *, *, #12310, .T. ) ;
#4921=CARTESIAN_POINT ( 'NONE',  ( -15.45084971874737256, 35.38125000068279746, -47.55282581475767500 ) ) ;
#4923=DIRECTION ( 'NONE',  ( -0.000000000000000000, -1.000000000000000000, -0.000000000000000000 ) ) ;
#4925=DIRECTION ( 'NONE',  ( 0.000000000000000000, 0.000000000000000000, 1.000000000000000000 ) ) ;
#4937=CARTESIAN_POINT ( 'NONE',  ( -49.99999999999999289, 27.89999999999999858, -16.24598481164531449 ) ) ;
#4939=CARTESIAN_POINT ( 'NONE',  ( -15.45084971874737256, 43.60000000000000142, -47.55282581475767500 ) ) ;
#4940=CARTESIAN_POINT ( 'NONE',  ( -40.34137639590981195, 46.05937500034139731, 29.30972558990012189 ) ) ;
#4945=CARTESIAN_POINT ( 'NONE',  ( 49.86468353125000164, 34.85937500034140157, -6.106662507704105588E-15 ) ) ;
#4949=CARTESIAN_POINT ( 'NONE',  ( 45.93954244148165600, 24.99999999999998579, -19.39188242381383276 ) ) ;
#4950=CARTESIAN_POINT ( 'NONE',  ( 50.00000000000000711, 46.68125000068279462, 16.24598481164530739 ) ) ;
#4953=CARTESIAN_POINT ( 'NONE',  ( 49.99999999999999289, 43.10000000000000142, -16.24598481164532160 ) ) ;
#4955=CARTESIAN_POINT ( 'NONE',  ( -40.45084971874737079, 29.98125000068279888, 29.38926261462367151 ) ) ;
#4959=CARTESIAN_POINT ( 'NONE',  ( 30.81806926056962936, 29.22187500034139873, -42.41743335407647209 ) ) ;
#4962=EDGE_CURVE ( 'NONE', #13481, #15793, #13880, .T. ) ;
#4964=CARTESIAN_POINT ( 'NONE',  ( 15.40903463028482356, 40.45937500034139589, 47.42413220539093999 ) ) ;
#4966=CARTESIAN_POINT ( 'NONE',  ( 50.00000000000000000, 24.78125000068279959, -6.123233995736766085E-15 ) ) ;
#4970=CARTESIAN_POINT ( 'NONE',  ( 15.40903463028482356, 22.52187500034139589, 47.42413220539093999 ) ) ;
#4975=CARTESIAN_POINT ( 'NONE',  ( -15.45084971874737256, 49.60000000000000853, -47.55282581475767500 ) ) ;
#4980=CARTESIAN_POINT ( 'NONE',  ( -40.34137639590981905, 35.72187500034139163, -29.30972558990011478 ) ) ;
#4981=CARTESIAN_POINT ( 'NONE',  ( -7.919222016226934890, 32.22999571913595673, 49.99999999999996447 ) ) ;
#4982=VERTEX_POINT ( 'NONE', #13977 ) ;
#4983=EDGE_LOOP ( 'NONE', ( #8353, #209, #490, #453 ) ) ;
#4989=VECTOR ( 'NONE', #3403, 1000.000000000000000 ) ;
#5000=CARTESIAN_POINT ( 'NONE',  ( -30.81806926056962226, 24.15937500034139873, 42.41743335407647919 ) ) ;
#5004=EDGE_CURVE ( 'NONE', #15357, #9775, #15592, .T. ) ;
#5007=CARTESIAN_POINT ( 'NONE',  ( -49.99999999999999289, 37.68125000068278752, -16.24598481164531449 ) ) ;
#5009=LINE ( 'NONE', #5087, #13407 ) ;
#5010=VERTEX_POINT ( 'NONE', #10091 ) ;
#5011=CARTESIAN_POINT ( 'NONE',  ( 49.99999999999999289, 38.88125000068279036, -16.24598481164532160 ) ) ;
#5022=CARTESIAN_POINT ( 'NONE',  ( 49.99999999999999289, 21.09999999999999787, -16.24598481164532160 ) ) ;
#5024=CARTESIAN_POINT ( 'NONE',  ( -49.99999999999999289, 44.09999999999999432, 16.24598481164533226 ) ) ;
#5025=CARTESIAN_POINT ( 'NONE',  ( -3.210462471511496205E-15, 45.35937500034139447, -52.43083105670540789 ) ) ;
#5032=CARTESIAN_POINT ( 'NONE',  ( 40.34137639590981905, 28.65937500034139873, 29.30972558990010768 ) ) ;
#5036=CARTESIAN_POINT ( 'NONE',  ( 45.33038492356498494, 25.00000000000000000, -20.77601661419118173 ) ) ;
#5046=CARTESIAN_POINT ( 'NONE',  ( 30.81806926056964002, 28.62187500034140086, 42.41743335407647209 ) ) ;
#5050=CARTESIAN_POINT ( 'NONE',  ( -40.34137639590981195, 38.05937500034139731, 29.30972558990012189 ) ) ;
#5051=ORIENTED_EDGE ( 'NONE', *, *, #9009, .F. ) ;
#5055=CARTESIAN_POINT ( 'NONE',  ( 30.90169943749475578, 20.48125000068279178, 42.53254041760200010 ) ) ;
#5058=CARTESIAN_POINT ( 'NONE',  ( -40.34137639590981195, 22.12187500034139731, 29.30972558990012189 ) ) ;
#5062=CARTESIAN_POINT ( 'NONE',  ( -15.45084971874737256, 45.60000000000000142, -47.55282581475767500 ) ) ;
#5064=CARTESIAN_POINT ( 'NONE',  ( 49.86468353125001585, 48.82187500034139305, 16.20201782572375038 ) ) ;
#5066=DIRECTION ( 'NONE',  ( -0.000000000000000000, -1.000000000000000000, -0.000000000000000000 ) ) ;
#5068=EDGE_LOOP ( 'NONE', ( #14822, #4576 ) ) ;
#5071=CARTESIAN_POINT ( 'NONE',  ( 40.45084971874737789, 44.79999999999999716, 29.38926261462365375 ) ) ;
#5080=VERTEX_POINT ( 'NONE', #421 ) ;
#5081=CARTESIAN_POINT ( 'NONE',  ( 9.631387414534489405E-15, 26.35937500034140157, 52.43083105670540789 ) ) ;
#5082=ORIENTED_EDGE ( 'NONE', *, *, #6849, .F. ) ;
#5083=CARTESIAN_POINT ( 'NONE',  ( 8.446640517145639571E-15, 26.50000000000000000, 50.00000000000000000 ) ) ;
#5087=CARTESIAN_POINT ( 'NONE',  ( 6.123233995736766085E-15, 193.4213562373095385, 50.00000000000000000 ) ) ;
#5088=CARTESIAN_POINT ( 'NONE',  ( -40.45084971874737789, 27.80000000000000071, -29.38926261462365730 ) ) ;
#5098=CARTESIAN_POINT ( 'NONE',  ( -40.45084971874737079, 22.19999999999999929, 29.38926261462367151 ) ) ;
#5101=CARTESIAN_POINT ( 'NONE',  ( 40.34137639590981195, 47.05937500034140442, -29.30972558990011834 ) ) ;
#5106=CARTESIAN_POINT ( 'NONE',  ( -15.40903463028481646, 27.45937500034139944, -47.42413220539093999 ) ) ;
#5111=CARTESIAN_POINT ( 'NONE',  ( 46.73878613316200870, 24.99999999999999289, -17.37815620099810587 ) ) ;
#5112=CARTESIAN_POINT ( 'NONE',  ( 15.40903463028482356, 34.52187500034140299, 47.42413220539093999 ) ) ;
#5113=CARTESIAN_POINT ( 'NONE',  ( 7.919222016226827421, 47.22999571913595673, -50.00000000000000000 ) ) ;
#5118=CARTESIAN_POINT ( 'NONE',  ( -49.99999999999999289, 29.88125000068279391, 16.24598481164533226 ) ) ;
#5122=CARTESIAN_POINT ( 'NONE',  ( -49.86468353125000164, 33.92187500034139447, 0.000000000000000000 ) ) ;
#5126=( BOUNDED_CURVE ( )  B_SPLINE_CURVE ( 2, ( #4892, #4981, #13595, #3551, #14920, #7381, #16258, #15093, #3720, #6056, #2202, #16012, #10947 ),
 .UNSPECIFIED., .F., .F. ) 
 B_SPLINE_CURVE_WITH_KNOTS ( ( 3, 2, 2, 2, 2, 2, 3 ),
 ( 0.5833333333333333703, 0.5866666666666666696, 0.5933333333333333792, 0.5999999999999999778, 0.6066666666666666874, 0.6133333333333332860, 0.6166666666666666963 ),
 .UNSPECIFIED. ) 
 CURVE ( )  GEOMETRIC_REPRESENTATION_ITEM ( )  RATIONAL_B_SPLINE_CURVE ( ( 0.9755282581475768211, 0.9755282581475771542, 1.000000000000000000, 0.9510565162951535312, 1.000000000000000000, 0.9510565162951535312, 1.000000000000000000, 0.9510565162951535312, 1.000000000000000000, 0.9510565162951535312, 1.000000000000000000, 0.9755282581475763770, 0.9755282581475768211 ) ) 
 REPRESENTATION_ITEM ( '' )  );
#5127=VERTEX_POINT ( 'NONE', #9410 ) ;
#5128=CARTESIAN_POINT ( 'NONE',  ( 15.40903463028481113, 35.25937500034139305, -47.42413220539094709 ) ) ;
#5132=CARTESIAN_POINT ( 'NONE',  ( -3.210462471511496205E-15, 47.35937500034138736, -52.43083105670540789 ) ) ;
#5134=CARTESIAN_POINT ( 'NONE',  ( 49.86468353125000164, 26.92187500034139802, -6.106662507704105588E-15 ) ) ;
#5135=DIRECTION ( 'NONE',  ( 0.000000000000000000, 0.000000000000000000, 1.000000000000000000 ) ) ;
#5137=CARTESIAN_POINT ( 'NONE',  ( 38.60409515610501074, 25.00000000000000000, -31.77615201968907144 ) ) ;
#5138=CARTESIAN_POINT ( 'NONE',  ( 40.45084971874737079, 49.20000000000000284, -29.38926261462366440 ) ) ;
#5140=CARTESIAN_POINT ( 'NONE',  ( -49.86468353125000164, 49.92187500034140157, 0.000000000000000000 ) ) ;
#5146=CARTESIAN_POINT ( 'NONE',  ( -2.547328955960238000E-13, 32.50000000000000000, 49.99999999999999289 ) ) ;
#5155=CARTESIAN_POINT ( 'NONE',  ( -7.919222016226870942, 36.22999571913594963, 49.99999999999997158 ) ) ;
#5158=CARTESIAN_POINT ( 'NONE',  ( -49.86468353124999453, 23.95937500034138878, 16.20201782572377525 ) ) ;
#5162=VERTEX_POINT ( 'NONE', #5361 ) ;
#5164=CYLINDRICAL_SURFACE ( 'NONE', #15546, 50.00000000000000000 ) ;
#5177=CARTESIAN_POINT ( 'NONE',  ( 50.00000000000000711, 20.90000000000000213, 16.24598481164530739 ) ) ;
#5181=CARTESIAN_POINT ( 'NONE',  ( -15.40903463028481646, 45.45937500034139589, -47.42413220539093999 ) ) ;
#5185=CARTESIAN_POINT ( 'NONE',  ( -30.81806926056962226, 30.15937500034139163, 42.41743335407647919 ) ) ;
#5187=CARTESIAN_POINT ( 'NONE',  ( 30.90169943749473802, 27.29999999999999716, -42.53254041760200721 ) ) ;
#5191=CARTESIAN_POINT ( 'NONE',  ( -49.86468353124999453, 34.02187500034140299, 16.20201782572377169 ) ) ;
#5196=CARTESIAN_POINT ( 'NONE',  ( -30.90169943749474513, 29.48125000068279888, -42.53254041760200721 ) ) ;
#5199=CARTESIAN_POINT ( 'NONE',  ( 15.40903463028482356, 34.52187500034140299, 47.42413220539093999 ) ) ;
#5204=CARTESIAN_POINT ( 'NONE',  ( 40.34137639590981905, 34.65937500034139873, 29.30972558990010768 ) ) ;
#5209=CARTESIAN_POINT ( 'NONE',  ( 30.90169943749474157, 21.08125000068279675, -42.53254041760200721 ) ) ;
#5212=CARTESIAN_POINT ( 'NONE',  ( 15.40903463028481113, 23.32187500034139660, -47.42413220539094709 ) ) ;
#5218=AXIS2_PLACEMENT_3D ( 'NONE', #15750, #14342, #13023 ) ;
#5219=CARTESIAN_POINT ( 'NONE',  ( 30.90169943749475578, 44.69999999999999574, 42.53254041760200010 ) ) ;
#5222=CARTESIAN_POINT ( 'NONE',  ( 40.34137639590981195, 49.12187500034139731, -29.30972558990011834 ) ) ;
#5224=EDGE_CURVE ( 'NONE', #3644, #7740, #7248, .T. ) ;
#5234=CARTESIAN_POINT ( 'NONE',  ( -49.99999999999999289, 31.89999999999999858, -16.24598481164531449 ) ) ;
#5235=CARTESIAN_POINT ( 'NONE',  ( 15.45084971874736723, 45.40000000000000568, -47.55282581475768211 ) ) ;
#5238=CARTESIAN_POINT ( 'NONE',  ( -40.34137639590981195, 46.12187500034139731, 29.30972558990012189 ) ) ;
#5242=VECTOR ( 'NONE', #15, 1000.000000000000000 ) ;
#5247=CARTESIAN_POINT ( 'NONE',  ( 0.000000000000000000, 51.99999999999999289, 0.000000000000000000 ) ) ;
#5250=CARTESIAN_POINT ( 'NONE',  ( -49.86468353125000164, 19.85937500034139447, 0.000000000000000000 ) ) ;
#5251=VERTEX_POINT ( 'NONE', #12229 ) ;
#5263=CARTESIAN_POINT ( 'NONE',  ( -6.668400408272873429E-15, 49.28125000068279604, -50.00000000000000000 ) ) ;
#5268=CARTESIAN_POINT ( 'NONE',  ( 49.99999999999999289, 25.10000000000000142, -16.24598481164532160 ) ) ;
#5271=CARTESIAN_POINT ( 'NONE',  ( 49.86468353125001585, 36.75937500034138594, 16.20201782572375038 ) ) ;
#5276=CARTESIAN_POINT ( 'NONE',  ( -15.40903463028481646, 31.45937500034139944, -47.42413220539093999 ) ) ;
#5277=ORIENTED_EDGE ( 'NONE', *, *, #8180, .F. ) ;
#5280=CARTESIAN_POINT ( 'NONE',  ( 46.50201513659349217, 25.00000000000000000, -18.00136805656013905 ) ) ;
#5281=CARTESIAN_POINT ( 'NONE',  ( -3.210462471511496205E-15, 31.42187500034139447, -52.43083105670540789 ) ) ;
#5282=EDGE_CURVE ( 'NONE', #1352, #16058, #13069, .T. ) ;
#5286=LINE ( 'NONE', #2680, #5242 ) ;
#5289=CARTESIAN_POINT ( 'NONE',  ( 15.40903463028482356, 30.52187500034139589, 47.42413220539093999 ) ) ;
#5290=AXIS2_PLACEMENT_3D ( 'NONE', #15024, #6475, #8712 ) ;
#5291=VERTEX_POINT ( 'NONE', #7087 ) ;
#5293=CARTESIAN_POINT ( 'NONE',  ( -49.86468353125000164, 33.85937500034139447, 0.000000000000000000 ) ) ;
#5298=CARTESIAN_POINT ( 'NONE',  ( -15.40903463028481646, 45.45937500034139589, -47.42413220539093999 ) ) ;
#5300=CARTESIAN_POINT ( 'NONE',  ( -15.40903463028480580, 24.32187500034139660, 47.42413220539094709 ) ) ;
#5301=FACE_OUTER_BOUND ( 'NONE', #980, .T. ) ;
#5305=CARTESIAN_POINT ( 'NONE',  ( -3.219174618344376363E-15, 45.49999999999999289, -52.57311121191334990 ) ) ;
#5308=CARTESIAN_POINT ( 'NONE',  ( -40.34137639590981905, 49.72187500034139873, -29.30972558990011478 ) ) ;
#5312=CARTESIAN_POINT ( 'NONE',  ( 15.45084971874736723, 39.18125000068280173, -47.55282581475768211 ) ) ;
#5318=CARTESIAN_POINT ( 'NONE',  ( 15.40903463028482356, 44.52187500034139589, 47.42413220539093999 ) ) ;
#5323=ADVANCED_FACE ( 'NONE', ( #3424 ), #2157, .T. ) ;
#5324=COLOUR_RGB ( '', 0.09019608, 0.27058824, 0.51372549) ;
#5329=ORIENTED_EDGE ( 'NONE', *, *, #5224, .F. ) ;
#5331=CARTESIAN_POINT ( 'NONE',  ( -49.86468353124999453, 45.82187500034140015, -16.20201782572375393 ) ) ;
#5333=DIRECTION ( 'NONE',  ( 0.000000000000000000, 0.000000000000000000, 1.000000000000000000 ) ) ;
#5338=CARTESIAN_POINT ( 'NONE',  ( -49.99999999999999289, 27.89999999999999858, -16.24598481164531449 ) ) ;
#5347=CARTESIAN_POINT ( 'NONE',  ( 30.90169943749474157, 23.29999999999999716, -42.53254041760200721 ) ) ;
#5350=CARTESIAN_POINT ( 'NONE',  ( -49.86468353124999453, 39.75937500034139305, -16.20201782572375393 ) ) ;
#5354=CARTESIAN_POINT ( 'NONE',  ( 9.631387414534489405E-15, 28.35937500034139802, 52.43083105670540789 ) ) ;
#5360=CARTESIAN_POINT ( 'NONE',  ( 40.34137639590981195, 35.12187500034139731, -29.30972558990011834 ) ) ;
#5361=CARTESIAN_POINT ( 'NONE',  ( 0.000000000000000000, 51.99999999999999289, -47.00000000000000000 ) ) ;
#5368=CARTESIAN_POINT ( 'NONE',  ( -49.86468353124999453, 27.82187500034139305, -16.20201782572375393 ) ) ;
#5372=CARTESIAN_POINT ( 'NONE',  ( 49.86468353124999453, 36.95937500034139589, -16.20201782572376104 ) ) ;
#5376=CARTESIAN_POINT ( 'NONE',  ( -49.99999999999999289, 19.88125000068279746, 16.24598481164533226 ) ) ;
#5377=DIRECTION ( 'NONE',  ( -0.8660254037844320463, 0.5000000000000113243, 0.000000000000000000 ) ) ;
#5382=CARTESIAN_POINT ( 'NONE',  ( -15.45084971874736368, 44.39999999999999858, 47.55282581475768211 ) ) ;
#5386=CARTESIAN_POINT ( 'NONE',  ( -3.219174618344376363E-15, 37.28125000068280315, -52.57311121191334990 ) ) ;
#5391=CARTESIAN_POINT ( 'NONE',  ( -30.81806926056962226, 46.22187500034139163, 42.41743335407647209 ) ) ;
#5396=CARTESIAN_POINT ( 'NONE',  ( 49.95625437244530787, 25.00000000000000000, -4.103175251694326953 ) ) ;
#5398=CARTESIAN_POINT ( 'NONE',  ( 49.99999999999999289, 28.88125000068279391, -16.24598481164532160 ) ) ;
#5402=CARTESIAN_POINT ( 'NONE',  ( -15.40903463028481646, 49.52187500034140299, -47.42413220539093999 ) ) ;
#5404=CARTESIAN_POINT ( 'NONE',  ( -15.45084971874737256, 25.60000000000000142, -47.55282581475767500 ) ) ;
#5417=DIRECTION ( 'NONE',  ( 0.000000000000000000, 1.000000000000000000, 0.000000000000000000 ) ) ;
#5423=ADVANCED_FACE ( 'NONE', ( #9987 ), #1240, .T. ) ;
#5424=CARTESIAN_POINT ( 'NONE',  ( -15.40903463028480580, 36.25937500034140015, 47.42413220539094709 ) ) ;
#5427=AXIS2_PLACEMENT_3D ( 'NONE', #3582, #2575, #11396 ) ;
#5428=CARTESIAN_POINT ( 'NONE',  ( 9.657523855033129090E-15, 48.28125000068279604, 52.57311121191334990 ) ) ;
#5430=CARTESIAN_POINT ( 'NONE',  ( -49.86468353124999453, 21.95937500034138878, 16.20201782572377525 ) ) ;
#5431=EDGE_LOOP ( 'NONE', ( #9971, #3138, #7314, #7575 ) ) ;
#5432=CARTESIAN_POINT ( 'NONE',  ( -15.45084971874736368, 48.40000000000000568, 47.55282581475768211 ) ) ;
#5435=CARTESIAN_POINT ( 'NONE',  ( 40.34137639590981905, 26.72187500034139518, 29.30972558990010768 ) ) ;
#5442=CARTESIAN_POINT ( 'NONE',  ( 40.45084971874737079, 35.20000000000000284, -29.38926261462366440 ) ) ;
#5444=ADVANCED_FACE ( 'NONE', ( #992 ), #9210, .T. ) ;
#5447=CARTESIAN_POINT ( 'NONE',  ( 49.86468353125000164, 26.85937500034139802, -6.106662507704105588E-15 ) ) ;
#5450=CARTESIAN_POINT ( 'NONE',  ( -49.86468353124999453, 41.95937500034138878, 16.20201782572377525 ) ) ;
#5458=( BOUNDED_CURVE ( )  B_SPLINE_CURVE ( 2, ( #6911, #12129, #5736, #13291, #11965, #1892, #10885, #10964, #561, #7153, #5903, #4570, #14686 ),
 .UNSPECIFIED., .F., .F. ) 
 B_SPLINE_CURVE_WITH_KNOTS ( ( 3, 2, 2, 2, 2, 2, 3 ),
 ( 0.4166666666666666852, 0.4199999999999999845, 0.4266666666666666941, 0.4333333333333333481, 0.4400000000000000022, 0.4466666666666666563, 0.4500000000000000111 ),
 .UNSPECIFIED. ) 
 CURVE ( )  GEOMETRIC_REPRESENTATION_ITEM ( )  RATIONAL_B_SPLINE_CURVE ( ( 0.9755282581475768211, 0.9755282581475770431, 1.000000000000000000, 0.9510565162951535312, 1.000000000000000000, 0.9510565162951535312, 1.000000000000000000, 0.9510565162951535312, 1.000000000000000000, 0.9510565162951535312, 1.000000000000000000, 0.9755282581475765991, 0.9755282581475768211 ) ) 
 REPRESENTATION_ITEM ( '' )  );
#5459=CARTESIAN_POINT ( 'NONE',  ( -40.45084971874737789, 41.80000000000000426, -29.38926261462365730 ) ) ;
#5462=CARTESIAN_POINT ( 'NONE',  ( -15.40903463028480580, 44.32187500034140015, 47.42413220539094709 ) ) ;
#5465=CARTESIAN_POINT ( 'NONE',  ( -3.210462471511496205E-15, 47.35937500034138736, -52.43083105670540789 ) ) ;
#5467=CARTESIAN_POINT ( 'NONE',  ( 15.45084971874737789, 38.38125000068279746, 47.55282581475767500 ) ) ;
#5470=DIRECTION ( 'NONE',  ( -0.000000000000000000, -1.000000000000000000, -0.000000000000000000 ) ) ;
#5473=CARTESIAN_POINT ( 'NONE',  ( -15.40903463028480580, 44.32187500034140015, 47.42413220539094709 ) ) ;
#5475=CARTESIAN_POINT ( 'NONE',  ( -40.45084971874737789, 39.58125000068280031, -29.38926261462365730 ) ) ;
#5478=DIRECTION ( 'NONE',  ( -0.000000000000000000, -1.000000000000000000, -0.000000000000000000 ) ) ;
#5482=ORIENTED_EDGE ( 'NONE', *, *, #10, .F. ) ;
#5484=CARTESIAN_POINT ( 'NONE',  ( -15.40903463028481646, 21.45937500034139589, -47.42413220539093999 ) ) ;
#5493=DIRECTION ( 'NONE',  ( -0.000000000000000000, -1.000000000000000000, -0.000000000000000000 ) ) ;
#5497=AXIS2_PLACEMENT_3D ( 'NONE', #8426, #13569, #11097 ) ;
#5502=CYLINDRICAL_SURFACE ( 'NONE', #14245, 50.00000000000000000 ) ;
#5504=CARTESIAN_POINT ( 'NONE',  ( 50.00000000000000000, 49.00000000000000000, -6.123233995736766085E-15 ) ) ;
#5506=CARTESIAN_POINT ( 'NONE',  ( -7.919222016226870942, 38.22999571913595673, 49.99999999999997158 ) ) ;
#5511=CARTESIAN_POINT ( 'NONE',  ( 49.86468353125001585, 38.75937500034139305, 16.20201782572375038 ) ) ;
#5512=ORIENTED_EDGE ( 'NONE', *, *, #3926, .F. ) ;
#5515=CARTESIAN_POINT ( 'NONE',  ( 30.90169943749474157, 49.08125000068280031, -42.53254041760200721 ) ) ;
#5517=CARTESIAN_POINT ( 'NONE',  ( 15.40903463028481113, 25.25937500034139660, -47.42413220539094709 ) ) ;
#5520=CARTESIAN_POINT ( 'NONE',  ( 50.00000000000000711, 34.89999999999999858, 16.24598481164530739 ) ) ;
#5522=CARTESIAN_POINT ( 'NONE',  ( 15.40903463028481113, 27.32187500034139660, -47.42413220539094709 ) ) ;
#5531=CARTESIAN_POINT ( 'NONE',  ( -15.45084971874737256, 35.60000000000000142, -47.55282581475767500 ) ) ;
#5536=EDGE_CURVE ( 'NONE', #5162, #1062, #685, .T. ) ;
#5537=CARTESIAN_POINT ( 'NONE',  ( 15.40903463028481113, 29.25937500034139660, -47.42413220539094709 ) ) ;
#5538=VECTOR ( 'NONE', #15538, 1000.000000000000000 ) ;
#5541=CARTESIAN_POINT ( 'NONE',  ( 30.81806926056964002, 44.55937500034139020, 42.41743335407647209 ) ) ;
#5543=CARTESIAN_POINT ( 'NONE',  ( -49.86468353125000164, 19.92187500034139447, 0.000000000000000000 ) ) ;
#5548=CARTESIAN_POINT ( 'NONE',  ( -30.90169943749474868, 41.70000000000000284, -42.53254041760200721 ) ) ;
#5550=CARTESIAN_POINT ( 'NONE',  ( 15.40903463028481113, 45.32187500034140015, -47.42413220539094709 ) ) ;
#5552=ADVANCED_FACE ( 'NONE', ( #540 ), #3040, .T. ) ;
#5555=CARTESIAN_POINT ( 'NONE',  ( -50.00000000000000000, 29.78125000068279959, 0.000000000000000000 ) ) ;
#5562=CARTESIAN_POINT ( 'NONE',  ( 30.81806926056964002, 44.62187500034139731, 42.41743335407646498 ) ) ;
#5572=CARTESIAN_POINT ( 'NONE',  ( -49.86468353125000164, 43.92187500034140157, 0.000000000000000000 ) ) ;
#5581=CARTESIAN_POINT ( 'NONE',  ( 0.000000000000000000, 52.00000000000000711, 0.000000000000000000 ) ) ;
#5582=PLANE ( 'NONE',  #3292 ) ;
#5584=CARTESIAN_POINT ( 'NONE',  ( -40.45084971874737789, 37.58125000068280031, -29.38926261462365730 ) ) ;
#5588=CARTESIAN_POINT ( 'NONE',  ( 30.81806926056964002, 34.55937500034139731, 42.41743335407647209 ) ) ;
#5589=AXIS2_PLACEMENT_3D ( 'NONE', #9549, #631, #389 ) ;
#5592=FACE_BOUND ( 'NONE', #206, .T. ) ;
#5594=CARTESIAN_POINT ( 'NONE',  ( 30.81806926056962936, 23.15937500034139873, -42.41743335407647209 ) ) ;
#5596=CARTESIAN_POINT ( 'NONE',  ( 8.446640517145639571E-15, 48.49999999999999289, 50.00000000000000000 ) ) ;
#5599=CARTESIAN_POINT ( 'NONE',  ( -49.86468353124999453, 30.02187500034139234, 16.20201782572377169 ) ) ;
#5604=CARTESIAN_POINT ( 'NONE',  ( 9.657523855033129090E-15, 32.50000000000000000, 52.57311121191334990 ) ) ;
#5609=CARTESIAN_POINT ( 'NONE',  ( 49.86468353125001585, 32.75937500034140015, 16.20201782572375038 ) ) ;
#5611=CARTESIAN_POINT ( 'NONE',  ( 0.000000000000000000, 53.82568851450475478, 0.000000000000000000 ) ) ;
#5612=CARTESIAN_POINT ( 'NONE',  ( -49.86468353124999453, 43.95937500034138878, 16.20201782572377525 ) ) ;
#5620=CARTESIAN_POINT ( 'NONE',  ( -49.99999999999999289, 39.90000000000001279, -16.24598481164531449 ) ) ;
#5624=CARTESIAN_POINT ( 'NONE',  ( -49.86468353125000164, 43.92187500034140157, 0.000000000000000000 ) ) ;
#5626=CARTESIAN_POINT ( 'NONE',  ( 49.86468353125000164, 46.85937500034139447, -6.106662507704105588E-15 ) ) ;
#5627=VERTEX_POINT ( 'NONE', #6888 ) ;
#5628=CARTESIAN_POINT ( 'NONE',  ( -40.45084971874737789, 29.58125000068279675, -29.38926261462365730 ) ) ;
#5630=FACE_OUTER_BOUND ( 'NONE', #1976, .T. ) ;
#5631=DIRECTION ( 'NONE',  ( 0.000000000000000000, 1.000000000000000000, 0.000000000000000000 ) ) ;
#5632=CARTESIAN_POINT ( 'NONE',  ( -40.34137639590981905, 41.72187500034139873, -29.30972558990011478 ) ) ;
#5634=CARTESIAN_POINT ( 'NONE',  ( -7.919222016226752814, 39.33250428222963535, -50.00000000000000711 ) ) ;
#5636=CARTESIAN_POINT ( 'NONE',  ( -2.445080149700054274E-14, 46.28125000068280315, 50.00000000000000000 ) ) ;
#5638=CARTESIAN_POINT ( 'NONE',  ( -15.40903463028481646, 41.52187500034139589, -47.42413220539093999 ) ) ;
#5650=CARTESIAN_POINT ( 'NONE',  ( -30.90169943749473447, 34.08125000068279320, 42.53254041760200721 ) ) ;
#5655=EDGE_CURVE ( 'NONE', #7759, #7784, #8060, .T. ) ;
#5658=CARTESIAN_POINT ( 'NONE',  ( -49.86468353124999453, 29.75937500034139305, -16.20201782572375393 ) ) ;
#5664=CARTESIAN_POINT ( 'NONE',  ( -30.81806926056963292, 25.55937500034139376, -42.41743335407647209 ) ) ;
#5665=VECTOR ( 'NONE', #3522, 1000.000000000000000 ) ;
#5670=CARTESIAN_POINT ( 'NONE',  ( 30.81806926056962936, 27.22187500034139518, -42.41743335407646498 ) ) ;
#5671=CARTESIAN_POINT ( 'NONE',  ( 7.919222016226875382, 39.44874571845315359, -49.99999999999997158 ) ) ;
#5676=CARTESIAN_POINT ( 'NONE',  ( -3.219174618344376363E-15, 37.50000000000000000, -52.57311121191334990 ) ) ;
#5681=CARTESIAN_POINT ( 'NONE',  ( -49.86468353124999453, 31.95937500034139944, 16.20201782572377169 ) ) ;
#5684=CARTESIAN_POINT ( 'NONE',  ( -15.40903463028481646, 39.45937500034139589, -47.42413220539093999 ) ) ;
#5693=CARTESIAN_POINT ( 'NONE',  ( -49.86468353124999453, 30.02187500034139234, 16.20201782572377525 ) ) ;
#5694=CARTESIAN_POINT ( 'NONE',  ( 40.45084971874737079, 39.19999999999999574, -29.38926261462366440 ) ) ;
#5696=CARTESIAN_POINT ( 'NONE',  ( 49.86468353125001585, 42.82187500034139305, 16.20201782572375038 ) ) ;
#5705=CARTESIAN_POINT ( 'NONE',  ( 40.45084971874737079, 28.98125000068279888, -29.38926261462366440 ) ) ;
#5710=CARTESIAN_POINT ( 'NONE',  ( 49.86468353124999453, 39.02187500034138878, -16.20201782572376104 ) ) ;
#5714=EDGE_CURVE ( 'NONE', #1840, #2524, #13106, .T. ) ;
#5719=CARTESIAN_POINT ( 'NONE',  ( 9.631387414534489405E-15, 44.42187500034140157, 52.43083105670540789 ) ) ;
#5720=ORIENTED_EDGE ( 'NONE', *, *, #2445, .T. ) ;
#5722=EDGE_CURVE ( 'NONE', #10705, #8435, #13587, .T. ) ;
#5726=DIRECTION ( 'NONE',  ( -0.000000000000000000, -1.000000000000000000, -0.000000000000000000 ) ) ;
#5736=CARTESIAN_POINT ( 'NONE',  ( 15.45084971874736723, 37.40000000000000568, -47.55282581475768211 ) ) ;
#5739=CARTESIAN_POINT ( 'NONE',  ( 49.86468353125001585, 32.75937500034140015, 16.20201782572375038 ) ) ;
#5744=CARTESIAN_POINT ( 'NONE',  ( -30.90169943749474868, 45.48125000068279178, -42.53254041760200721 ) ) ;
#5749=CARTESIAN_POINT ( 'NONE',  ( -40.34137639590981195, 22.05937500034139731, 29.30972558990012189 ) ) ;
#5755=DIRECTION ( 'NONE',  ( 0.000000000000000000, 0.000000000000000000, -1.000000000000000000 ) ) ;
#5756=CARTESIAN_POINT ( 'NONE',  ( 49.86468353125000164, 26.92187500034139802, -6.106662507704105588E-15 ) ) ;
#5758=CARTESIAN_POINT ( 'NONE',  ( 7.919222016226875382, 37.22999571913595673, -49.99999999999997158 ) ) ;
#5762=CARTESIAN_POINT ( 'NONE',  ( -30.90169943749474868, 37.70000000000000995, -42.53254041760200721 ) ) ;
#5764=AXIS2_PLACEMENT_3D ( 'NONE', #7468, #6146, #8540 ) ;
#5766=CARTESIAN_POINT ( 'NONE',  ( -40.34137639590981905, 49.65937500034139873, -29.30972558990011478 ) ) ;
#5771=CARTESIAN_POINT ( 'NONE',  ( 40.34137639590981195, 39.05937500034140442, -29.30972558990011834 ) ) ;
#5775=VECTOR ( 'NONE', #13442, 1000.000000000000000 ) ;
#5776=FACE_OUTER_BOUND ( 'NONE', #12710, .T. ) ;
#5780=CARTESIAN_POINT ( 'NONE',  ( 30.81806926056962936, 33.22187500034139163, -42.41743335407647209 ) ) ;
#5782=CARTESIAN_POINT ( 'NONE',  ( 40.34137639590981195, 41.12187500034139731, -29.30972558990011834 ) ) ;
#5785=CARTESIAN_POINT ( 'NONE',  ( 15.40903463028482356, 48.45937500034140299, 47.42413220539093999 ) ) ;
#5786=ORIENTED_EDGE ( 'NONE', *, *, #4962, .F. ) ;
#5787=EDGE_LOOP ( 'NONE', ( #15096, #4539, #2231, #13857, #12431, #7474, #13355, #11479, #15877, #12869, #9128, #16080, #12737, #14862, #4000, #5849, #6759, #14592, #9126, #3940, #3257, #12413, #8782, #304, #4409, #138, #7279, #10652, #6232 ) ) ;
#5788=CARTESIAN_POINT ( 'NONE',  ( -50.00000000000000000, 31.78125000068279959, 0.000000000000000000 ) ) ;
#5789=VERTEX_POINT ( 'NONE', #7127 ) ;
#5791=CARTESIAN_POINT ( 'NONE',  ( 49.86468353124999453, 43.02187500034138878, -16.20201782572376104 ) ) ;
#5798=ORIENTED_EDGE ( 'NONE', *, *, #2349, .T. ) ;
#5799=CARTESIAN_POINT ( 'NONE',  ( -49.86468353125000164, 39.92187500034139447, 0.000000000000000000 ) ) ;
#5814=LINE ( 'NONE', #808, #13967 ) ;
#5820=CARTESIAN_POINT ( 'NONE',  ( 7.919222016226809657, 25.22999571913595318, -50.00000000000000000 ) ) ;
#5822=CARTESIAN_POINT ( 'NONE',  ( -30.81806926056962226, 34.15937500034139163, 42.41743335407647919 ) ) ;
#5826=CARTESIAN_POINT ( 'NONE',  ( -49.99999999999999289, 43.68125000068279462, -16.24598481164531449 ) ) ;
#5827=STYLED_ITEM ( 'NONE', ( #7630 ), #3161 ) ;
#5838=CARTESIAN_POINT ( 'NONE',  ( 15.45084971874736723, 37.18125000068280173, -47.55282581475768211 ) ) ;
#5842=( BOUNDED_SURFACE ( )  B_SPLINE_SURFACE ( 1, 2, ( 
 ( #6677, #8065, #11893, #4335, #2836, #10729, #11807, #5515, #14449, #247, #3074, #4177, #7904, #1585, #15790, #5428, #491, #11727, #9490, #13060, #327, #10654, #14536, #10487, #3162, #15545, #1505, #14297, #2920, #6762, #16207, #12219, #8310, #3494, #2147, #8233, #647, #15880, #8549, #983, #8391, #13463, #5910, #5744, #15956, #9732, #7072, #14613, #13376, #14695, #12138, #12048, #1980, #9893, #10818, #14781, #2070, #10892, #741, #4502, #12295, #5826, #4663, #3412, #16131, #9569, #6082, #7159, #821, #4758, #1898, #14866, #4577, #6991, #3237, #11149, #9641, #7235, #3321, #7320, #10970, #16036, #897, #8477, #13542, #13619, #5993, #14948, #2228, #11061, #9814, #4838, #12386, #13298, #15501, #14170, #3575, #12471, #11227, #4125, #13019, #3959, #9034, #1456, #1063, #11305, #5312, #2398, #9975, #8718, #10288, #7476, #7402, #13784, #5467, #6155, #10362, #10536, #16283, #14089, #2788, #5007, #15422, #2704, #10444, #5386, #15342, #7782, #12544, #8631, #207, #12853, #13701, #6551, #2318, #365, #1140, #11612, #6234, #12942, #2878, #9202, #4042, #1546, #4921, #16367, #14258, #15032, #9111, #7864, #3662, #6638, #11687, #287, #7946, #1621, #6715, #11765, #4543, #2030, #9606, #779, #15921, #1703, #12091, #11853, #3200, #8352, #6957, #14495, #533, #4374, #6880, #7121, #12179, #4464, #3124, #13185, #15839, #14654, #5788, #6799, #3282, #15673, #8196, #4296, #10855, #9530, #15595, #8022, #454, #13415, #5871, #15746, #9441, #13262, #13098, #11933, #609, #14410, #5555, #9360, #5628, #3033, #2955, #8103, #4216, #10617, #5705, #9284, #1789, #1862, #14576, #10690, #10772, #12011, #14338, #699, #8274, #13338, #1942, #7035, #7371, #940, #4623, #3537, #9686, #7518, #4720, #11112, #9778, #3622, #10028, #6199, #16171, #8685, #2109, #14825, #16329, #10933, #16081, #3455, #7196, #8516, #14736, #16247, #7447, #3707, #14908, #3370, #4966, #13828, #15080, #12590, #11271, #13501, #12512, #12259, #14992, #8766, #2275, #9856, #12341, #4803, #2187, #2440, #1186, #4880, #8591, #13581, #11194, #15996, #1104, #861, #8438, #11017, #13664, #7283, #6041, #5954, #13750, #12434, #1027, #6122, #2363, #9938, #15485, #5209, #10267, #14155, #16420, #12923, #13996, #5055, #10106, #4109, #15237, #191, #26, #5376, #1356 ),
 ( #6448, #14240, #8846, #2771, #2526, #10346, #9180, #14075, #15327, #7689, #11507, #2613, #2861, #7930, #11592, #3946, #3864, #6529, #11672, #1529, #13907, #271, #6368, #104, #8934, #5132, #3784, #15410, #10185, #2690, #7765, #7846, #7605, #13003, #9019, #12836, #6619, #15158, #10430, #12759, #12682, #1278, #6283, #1440, #5298, #4027, #11355, #9097, #11434, #10753, #10677, #15656, #1922, #5541, #3263, #12071, #2941, #13161, #9591, #5612, #1687, #13321, #11994, #1607, #10515, #9266, #7016, #10840, #1771, #6869, #15729, #15576, #9345, #3104, #438, #8008, #6784, #8088, #10601, #5450, #11829, #8333, #4202, #8179, #6700, #14322, #11919, #592, #3017, #13246, #517, #8257, #3184, #4359, #9423, #4281, #11750, #14471, #1845, #351, #6941, #13082, #14638, #14396, #5684, #15814, #4446, #673, #5771, #9512, #14560, #15904, #4527, #2344, #13397, #2092, #5936, #9665, #11000, #12161, #2252, #9920, #6179, #922, #5853, #7425, #16310, #12494, #15060, #13731, #13564, #4781, #4692, #3599, #16230, #4863, #7104, #9840, #11251, #763, #11089, #13643, #14973, #14891, #12320, #16060, #9760, #844, #3689, #14716, #4945, #14805, #7264, #3437, #2170, #8662, #1087, #6020, #7181, #10916, #10003, #2007, #7350, #15979, #4605, #12242, #3348, #8419, #13485, #8500, #1006, #16153, #3519, #12415, #8572, #6105, #11175, #11482, #11412, #12896, #6505, #249, #171, #15302, #5276, #12569, #7822, #13971, #10239, #13808, #10409, #10326, #1413, #1507, #15385, #11561, #1164, #5185, #4006, #9077, #14131, #2748, #4, #6599, #3924, #7498, #15134, #11652, #6261, #8996, #2591, #2500, #5032, #10160, #7743, #5354, #2420, #15464, #8743, #12811, #11333, #16398, #10085, #3762, #5106, #8821, #13885, #14054, #7577, #12659, #7666, #1254, #6346, #15212, #2670, #3841, #8906, #12736, #1332, #80, #6424, #11895, #3079, #5664, #1900, #4260, #5517, #2838, #14538, #2922, #13139, #9404, #8235, #6993, #8158, #10656, #3165, #9156, #13300, #14212, #9326, #494, #11809, #10732, #6920, #11973, #7906, #5594, #12050, #12983, #1746, #4338, #570, #15709, #2997, #6764, #412, #7988, #5749, #5430, #649, #10579, #14377, #15636, #8067, #15792, #4419, #6847, #14300, #1587, #10820, #4085, #14451, #6679, #11729, #13062, #330, #10489, #15548, #1665, #13225 ) ),
 .UNSPECIFIED., .F., .F., .F. ) 
 B_SPLINE_SURFACE_WITH_KNOTS ( ( 2, 2 ),
 ( 3, 2, 2, 2, 2, 2, 2, 2, 2, 2, 2, 2, 2, 2, 2, 2, 2, 2, 2, 2, 2, 2, 2, 2, 2, 2, 2, 2, 2, 2, 2, 2, 2, 2, 2, 2, 2, 2, 2, 2, 2, 2, 2, 2, 2, 2, 2, 2, 2, 2, 2, 2, 2, 2, 2, 2, 2, 2, 2, 2, 2, 2, 2, 2, 2, 2, 2, 2, 2, 2, 2, 2, 2, 2, 2, 2, 2, 2, 2, 2, 2, 2, 2, 2, 2, 2, 2, 2, 2, 2, 2, 2, 2, 2, 2, 2, 2, 2, 2, 2, 2, 2, 2, 2, 2, 2, 2, 2, 2, 2, 2, 2, 2, 2, 2, 2, 2, 2, 2, 2, 2, 2, 2, 2, 2, 2, 2, 2, 2, 2, 2, 2, 2, 2, 2, 2, 2, 2, 2, 2, 2, 2, 2, 2, 2, 2, 2, 2, 2, 2, 3 ),
 ( 0.000000000000000000, 1.000000000000000000 ),
 ( 0.000000000000000000, 0.006666666666666667095, 0.01333333333333333419, 0.02000000000000000042, 0.02666666666666666838, 0.03333333333333333287, 0.04000000000000000083, 0.04666666666666666879, 0.05333333333333333676, 0.05999999999999999778, 0.06666666666666666574, 0.07333333333333333370, 0.08000000000000000167, 0.08666666666666666963, 0.09333333333333333759, 0.1000000000000000056, 0.1066666666666666735, 0.1133333333333333276, 0.1199999999999999956, 0.1266666666666666774, 0.1333333333333333315, 0.1400000000000000133, 0.1466666666666666674, 0.1533333333333333215, 0.1600000000000000033, 0.1666666666666666574, 0.1733333333333333393, 0.1799999999999999933, 0.1866666666666666752, 0.1933333333333333293, 0.2000000000000000111, 0.2066666666666666652, 0.2133333333333333470, 0.2200000000000000011, 0.2266666666666666552, 0.2333333333333333370, 0.2399999999999999911, 0.2466666666666666730, 0.2533333333333333548, 0.2600000000000000089, 0.2666666666666666630, 0.2733333333333333171, 0.2800000000000000266, 0.2866666666666666807, 0.2933333333333333348, 0.2999999999999999889, 0.3066666666666666430, 0.3133333333333333526, 0.3200000000000000067, 0.3266666666666666607, 0.3333333333333333148, 0.3400000000000000244, 0.3466666666666666785, 0.3533333333333333326, 0.3599999999999999867, 0.3666666666666666408, 0.3733333333333333504, 0.3800000000000000044, 0.3866666666666666585, 0.3933333333333333126, 0.4000000000000000222, 0.4066666666666666763, 0.4133333333333333304, 0.4199999999999999845, 0.4266666666666666941, 0.4333333333333333481, 0.4400000000000000022, 0.4466666666666666563, 0.4533333333333333104, 0.4600000000000000200, 0.4666666666666666741, 0.4733333333333333282, 0.4799999999999999822, 0.4866666666666666918, 0.4933333333333333459, 0.5000000000000000000, 0.5066666666666667096, 0.5133333333333333082, 0.5200000000000000178, 0.5266666666666666163, 0.5333333333333333259, 0.5400000000000000355, 0.5466666666666666341, 0.5533333333333333437, 0.5600000000000000533, 0.5666666666666666519, 0.5733333333333333615, 0.5799999999999999600, 0.5866666666666666696, 0.5933333333333333792, 0.5999999999999999778, 0.6066666666666666874, 0.6133333333333332860, 0.6199999999999999956, 0.6266666666666667052, 0.6333333333333333037, 0.6400000000000000133, 0.6466666666666666119, 0.6533333333333333215, 0.6600000000000000311, 0.6666666666666666297, 0.6733333333333333393, 0.6800000000000000488, 0.6866666666666666474, 0.6933333333333333570, 0.6999999999999999556, 0.7066666666666666652, 0.7133333333333333748, 0.7199999999999999734, 0.7266666666666666829, 0.7333333333333332815, 0.7399999999999999911, 0.7466666666666667007, 0.7533333333333332993, 0.7600000000000000089, 0.7666666666666667185, 0.7733333333333333171, 0.7800000000000000266, 0.7866666666666666252, 0.7933333333333333348, 0.8000000000000000444, 0.8066666666666666430, 0.8133333333333333526, 0.8199999999999999512, 0.8266666666666666607, 0.8333333333333333703, 0.8399999999999999689, 0.8466666666666666785, 0.8533333333333333881, 0.8599999999999999867, 0.8666666666666666963, 0.8733333333333332948, 0.8800000000000000044, 0.8866666666666667140, 0.8933333333333333126, 0.9000000000000000222, 0.9066666666666666208, 0.9133333333333333304, 0.9200000000000000400, 0.9266666666666666385, 0.9333333333333333481, 0.9399999999999999467, 0.9466666666666666563, 0.9533333333333333659, 0.9599999999999999645, 0.9666666666666666741, 0.9733333333333333837, 0.9799999999999999822, 0.9866666666666666918, 0.9933333333333332904, 1.000000000000000000 ),
 .UNSPECIFIED. ) 
 GEOMETRIC_REPRESENTATION_ITEM ( )  RATIONAL_B_SPLINE_SURFACE ( (
 ( 1.000000000000000000, 0.9510565162951535312, 1.000000000000000000, 0.9510565162951535312, 1.000000000000000000, 0.9510565162951535312, 1.000000000000000000, 0.9510565162951535312, 1.000000000000000000, 0.9510565162951535312, 1.000000000000000000, 0.9510565162951535312, 1.000000000000000000, 0.9510565162951535312, 1.000000000000000000, 0.9510565162951535312, 1.000000000000000000, 0.9510565162951535312, 1.000000000000000000, 0.9510565162951535312, 1.000000000000000000, 0.9510565162951535312, 1.000000000000000000, 0.9510565162951535312, 1.000000000000000000, 0.9510565162951535312, 1.000000000000000000, 0.9510565162951535312, 1.000000000000000000, 0.9510565162951535312, 1.000000000000000000, 0.9510565162951535312, 1.000000000000000000, 0.9510565162951535312, 1.000000000000000000, 0.9510565162951535312, 1.000000000000000000, 0.9510565162951535312, 1.000000000000000000, 0.9510565162951535312, 1.000000000000000000, 0.9510565162951535312, 1.000000000000000000, 0.9510565162951535312, 1.000000000000000000, 0.9510565162951535312, 1.000000000000000000, 0.9510565162951535312, 1.000000000000000000, 0.9510565162951535312, 1.000000000000000000, 0.9510565162951535312, 1.000000000000000000, 0.9510565162951535312, 1.000000000000000000, 0.9510565162951535312, 1.000000000000000000, 0.9510565162951535312, 1.000000000000000000, 0.9510565162951535312, 1.000000000000000000, 0.9510565162951535312, 1.000000000000000000, 0.9510565162951535312, 1.000000000000000000, 0.9510565162951535312, 1.000000000000000000, 0.9510565162951535312, 1.000000000000000000, 0.9510565162951535312, 1.000000000000000000, 0.9510565162951535312, 1.000000000000000000, 0.9510565162951535312, 1.000000000000000000, 0.9510565162951535312, 1.000000000000000000, 0.9510565162951535312, 1.000000000000000000, 0.9510565162951535312, 1.000000000000000000, 0.9510565162951535312, 1.000000000000000000, 0.9510565162951535312, 1.000000000000000000, 0.9510565162951535312, 1.000000000000000000, 0.9510565162951535312, 1.000000000000000000, 0.9510565162951535312, 1.000000000000000000, 0.9510565162951535312, 1.000000000000000000, 0.9510565162951535312, 1.000000000000000000, 0.9510565162951535312, 1.000000000000000000, 0.9510565162951535312, 1.000000000000000000, 0.9510565162951535312, 1.000000000000000000, 0.9510565162951535312, 1.000000000000000000, 0.9510565162951535312, 1.000000000000000000, 0.9510565162951535312, 1.000000000000000000, 0.9510565162951535312, 1.000000000000000000, 0.9510565162951535312, 1.000000000000000000, 0.9510565162951535312, 1.000000000000000000, 0.9510565162951535312, 1.000000000000000000, 0.9510565162951535312, 1.000000000000000000, 0.9510565162951535312, 1.000000000000000000, 0.9510565162951535312, 1.000000000000000000, 0.9510565162951535312, 1.000000000000000000, 0.9510565162951535312, 1.000000000000000000, 0.9510565162951535312, 1.000000000000000000, 0.9510565162951535312, 1.000000000000000000, 0.9510565162951535312, 1.000000000000000000, 0.9510565162951535312, 1.000000000000000000, 0.9510565162951535312, 1.000000000000000000, 0.9510565162951535312, 1.000000000000000000, 0.9510565162951535312, 1.000000000000000000, 0.9510565162951535312, 1.000000000000000000, 0.9510565162951535312, 1.000000000000000000, 0.9510565162951535312, 1.000000000000000000, 0.9510565162951535312, 1.000000000000000000, 0.9510565162951535312, 1.000000000000000000, 0.9510565162951535312, 1.000000000000000000, 0.9510565162951535312, 1.000000000000000000, 0.9510565162951535312, 1.000000000000000000, 0.9510565162951535312, 1.000000000000000000, 0.9510565162951535312, 1.000000000000000000, 0.9510565162951535312, 1.000000000000000000, 0.9510565162951535312, 1.000000000000000000, 0.9510565162951535312, 1.000000000000000000, 0.9510565162951535312, 1.000000000000000000, 0.9510565162951535312, 1.000000000000000000, 0.9510565162951535312, 1.000000000000000000, 0.9510565162951535312, 1.000000000000000000, 0.9510565162951535312, 1.000000000000000000, 0.9510565162951535312, 1.000000000000000000, 0.9510565162951535312, 1.000000000000000000, 0.9510565162951535312, 1.000000000000000000, 0.9510565162951535312, 1.000000000000000000, 0.9510565162951535312, 1.000000000000000000, 0.9510565162951535312, 1.000000000000000000, 0.9510565162951535312, 1.000000000000000000, 0.9510565162951535312, 1.000000000000000000, 0.9510565162951535312, 1.000000000000000000, 0.9510565162951535312, 1.000000000000000000, 0.9510565162951535312, 1.000000000000000000, 0.9510565162951535312, 1.000000000000000000, 0.9510565162951535312, 1.000000000000000000, 0.9510565162951535312, 1.000000000000000000, 0.9510565162951535312, 1.000000000000000000, 0.9510565162951535312, 1.000000000000000000, 0.9510565162951535312, 1.000000000000000000, 0.9510565162951535312, 1.000000000000000000, 0.9510565162951535312, 1.000000000000000000, 0.9510565162951535312, 1.000000000000000000, 0.9510565162951535312, 1.000000000000000000, 0.9510565162951535312, 1.000000000000000000, 0.9510565162951535312, 1.000000000000000000, 0.9510565162951535312, 1.000000000000000000, 0.9510565162951535312, 1.000000000000000000, 0.9510565162951535312, 1.000000000000000000, 0.9510565162951535312, 1.000000000000000000, 0.9510565162951535312, 1.000000000000000000, 0.9510565162951535312, 1.000000000000000000, 0.9510565162951535312, 1.000000000000000000, 0.9510565162951535312, 1.000000000000000000, 0.9510565162951535312, 1.000000000000000000, 0.9510565162951535312, 1.000000000000000000, 0.9510565162951535312, 1.000000000000000000, 0.9510565162951535312, 1.000000000000000000, 0.9510565162951535312, 1.000000000000000000, 0.9510565162951535312, 1.000000000000000000, 0.9510565162951535312, 1.000000000000000000, 0.9510565162951535312, 1.000000000000000000, 0.9510565162951535312, 1.000000000000000000, 0.9510565162951535312, 1.000000000000000000, 0.9510565162951535312, 1.000000000000000000, 0.9510565162951535312, 1.000000000000000000, 0.9510565162951535312, 1.000000000000000000, 0.9510565162951535312, 1.000000000000000000, 0.9510565162951535312, 1.000000000000000000, 0.9510565162951535312, 1.000000000000000000, 0.9510565162951535312, 1.000000000000000000, 0.9510565162951535312, 1.000000000000000000, 0.9510565162951535312, 1.000000000000000000, 0.9510565162951535312, 1.000000000000000000, 0.9510565162951535312, 1.000000000000000000, 0.9510565162951535312, 1.000000000000000000, 0.9510565162951535312, 1.000000000000000000, 0.9510565162951535312, 1.000000000000000000, 0.9510565162951535312, 1.000000000000000000, 0.9510565162951535312, 1.000000000000000000, 0.9510565162951535312, 1.000000000000000000, 0.9510565162951535312, 1.000000000000000000, 0.9510565162951535312, 1.000000000000000000, 0.9510565162951535312, 1.000000000000000000, 0.9510565162951535312, 1.000000000000000000, 0.9510565162951535312, 1.000000000000000000),
 ( 1.000000000000000000, 0.9510565162951535312, 1.000000000000000000, 0.9510565162951535312, 1.000000000000000000, 0.9510565162951535312, 1.000000000000000000, 0.9510565162951535312, 1.000000000000000000, 0.9510565162951535312, 1.000000000000000000, 0.9510565162951535312, 1.000000000000000000, 0.9510565162951535312, 1.000000000000000000, 0.9510565162951535312, 1.000000000000000000, 0.9510565162951535312, 1.000000000000000000, 0.9510565162951535312, 1.000000000000000000, 0.9510565162951535312, 1.000000000000000000, 0.9510565162951535312, 1.000000000000000000, 0.9510565162951535312, 1.000000000000000000, 0.9510565162951535312, 1.000000000000000000, 0.9510565162951535312, 1.000000000000000000, 0.9510565162951535312, 1.000000000000000000, 0.9510565162951535312, 1.000000000000000000, 0.9510565162951535312, 1.000000000000000000, 0.9510565162951535312, 1.000000000000000000, 0.9510565162951535312, 1.000000000000000000, 0.9510565162951535312, 1.000000000000000000, 0.9510565162951535312, 1.000000000000000000, 0.9510565162951535312, 1.000000000000000000, 0.9510565162951535312, 1.000000000000000000, 0.9510565162951535312, 1.000000000000000000, 0.9510565162951535312, 1.000000000000000000, 0.9510565162951535312, 1.000000000000000000, 0.9510565162951535312, 1.000000000000000000, 0.9510565162951535312, 1.000000000000000000, 0.9510565162951535312, 1.000000000000000000, 0.9510565162951535312, 1.000000000000000000, 0.9510565162951535312, 1.000000000000000000, 0.9510565162951535312, 1.000000000000000000, 0.9510565162951535312, 1.000000000000000000, 0.9510565162951535312, 1.000000000000000000, 0.9510565162951535312, 1.000000000000000000, 0.9510565162951535312, 1.000000000000000000, 0.9510565162951535312, 1.000000000000000000, 0.9510565162951535312, 1.000000000000000000, 0.9510565162951535312, 1.000000000000000000, 0.9510565162951535312, 1.000000000000000000, 0.9510565162951535312, 1.000000000000000000, 0.9510565162951535312, 1.000000000000000000, 0.9510565162951535312, 1.000000000000000000, 0.9510565162951535312, 1.000000000000000000, 0.9510565162951535312, 1.000000000000000000, 0.9510565162951535312, 1.000000000000000000, 0.9510565162951535312, 1.000000000000000000, 0.9510565162951535312, 1.000000000000000000, 0.9510565162951535312, 1.000000000000000000, 0.9510565162951535312, 1.000000000000000000, 0.9510565162951535312, 1.000000000000000000, 0.9510565162951535312, 1.000000000000000000, 0.9510565162951535312, 1.000000000000000000, 0.9510565162951535312, 1.000000000000000000, 0.9510565162951535312, 1.000000000000000000, 0.9510565162951535312, 1.000000000000000000, 0.9510565162951535312, 1.000000000000000000, 0.9510565162951535312, 1.000000000000000000, 0.9510565162951535312, 1.000000000000000000, 0.9510565162951535312, 1.000000000000000000, 0.9510565162951535312, 1.000000000000000000, 0.9510565162951535312, 1.000000000000000000, 0.9510565162951535312, 1.000000000000000000, 0.9510565162951535312, 1.000000000000000000, 0.9510565162951535312, 1.000000000000000000, 0.9510565162951535312, 1.000000000000000000, 0.9510565162951535312, 1.000000000000000000, 0.9510565162951535312, 1.000000000000000000, 0.9510565162951535312, 1.000000000000000000, 0.9510565162951535312, 1.000000000000000000, 0.9510565162951535312, 1.000000000000000000, 0.9510565162951535312, 1.000000000000000000, 0.9510565162951535312, 1.000000000000000000, 0.9510565162951535312, 1.000000000000000000, 0.9510565162951535312, 1.000000000000000000, 0.9510565162951535312, 1.000000000000000000, 0.9510565162951535312, 1.000000000000000000, 0.9510565162951535312, 1.000000000000000000, 0.9510565162951535312, 1.000000000000000000, 0.9510565162951535312, 1.000000000000000000, 0.9510565162951535312, 1.000000000000000000, 0.9510565162951535312, 1.000000000000000000, 0.9510565162951535312, 1.000000000000000000, 0.9510565162951535312, 1.000000000000000000, 0.9510565162951535312, 1.000000000000000000, 0.9510565162951535312, 1.000000000000000000, 0.9510565162951535312, 1.000000000000000000, 0.9510565162951535312, 1.000000000000000000, 0.9510565162951535312, 1.000000000000000000, 0.9510565162951535312, 1.000000000000000000, 0.9510565162951535312, 1.000000000000000000, 0.9510565162951535312, 1.000000000000000000, 0.9510565162951535312, 1.000000000000000000, 0.9510565162951535312, 1.000000000000000000, 0.9510565162951535312, 1.000000000000000000, 0.9510565162951535312, 1.000000000000000000, 0.9510565162951535312, 1.000000000000000000, 0.9510565162951535312, 1.000000000000000000, 0.9510565162951535312, 1.000000000000000000, 0.9510565162951535312, 1.000000000000000000, 0.9510565162951535312, 1.000000000000000000, 0.9510565162951535312, 1.000000000000000000, 0.9510565162951535312, 1.000000000000000000, 0.9510565162951535312, 1.000000000000000000, 0.9510565162951535312, 1.000000000000000000, 0.9510565162951535312, 1.000000000000000000, 0.9510565162951535312, 1.000000000000000000, 0.9510565162951535312, 1.000000000000000000, 0.9510565162951535312, 1.000000000000000000, 0.9510565162951535312, 1.000000000000000000, 0.9510565162951535312, 1.000000000000000000, 0.9510565162951535312, 1.000000000000000000, 0.9510565162951535312, 1.000000000000000000, 0.9510565162951535312, 1.000000000000000000, 0.9510565162951535312, 1.000000000000000000, 0.9510565162951535312, 1.000000000000000000, 0.9510565162951535312, 1.000000000000000000, 0.9510565162951535312, 1.000000000000000000, 0.9510565162951535312, 1.000000000000000000, 0.9510565162951535312, 1.000000000000000000, 0.9510565162951535312, 1.000000000000000000, 0.9510565162951535312, 1.000000000000000000, 0.9510565162951535312, 1.000000000000000000, 0.9510565162951535312, 1.000000000000000000, 0.9510565162951535312, 1.000000000000000000, 0.9510565162951535312, 1.000000000000000000, 0.9510565162951535312, 1.000000000000000000, 0.9510565162951535312, 1.000000000000000000, 0.9510565162951535312, 1.000000000000000000, 0.9510565162951535312, 1.000000000000000000, 0.9510565162951535312, 1.000000000000000000, 0.9510565162951535312, 1.000000000000000000, 0.9510565162951535312, 1.000000000000000000, 0.9510565162951535312, 1.000000000000000000, 0.9510565162951535312, 1.000000000000000000, 0.9510565162951535312, 1.000000000000000000, 0.9510565162951535312, 1.000000000000000000, 0.9510565162951535312, 1.000000000000000000, 0.9510565162951535312, 1.000000000000000000, 0.9510565162951535312, 1.000000000000000000, 0.9510565162951535312, 1.000000000000000000, 0.9510565162951535312, 1.000000000000000000, 0.9510565162951535312, 1.000000000000000000, 0.9510565162951535312, 1.000000000000000000, 0.9510565162951535312, 1.000000000000000000, 0.9510565162951535312, 1.000000000000000000, 0.9510565162951535312, 1.000000000000000000, 0.9510565162951535312, 1.000000000000000000, 0.9510565162951535312, 1.000000000000000000) ) ) 
 REPRESENTATION_ITEM ( '' )  SURFACE ( )  );
#5845=CARTESIAN_POINT ( 'NONE',  ( 30.90169943749474157, 31.30000000000000071, -42.53254041760200721 ) ) ;
#5847=EDGE_CURVE ( 'NONE', #11087, #9397, #9038, .T. ) ;
#5849=ORIENTED_EDGE ( 'NONE', *, *, #3392, .T. ) ;
#5853=CARTESIAN_POINT ( 'NONE',  ( -15.40903463028481646, 37.45937500034139589, -47.42413220539093999 ) ) ;
#5856=CARTESIAN_POINT ( 'NONE',  ( 15.45084971874736723, 45.18125000068280173, -47.55282581475768211 ) ) ;
#5860=CARTESIAN_POINT ( 'NONE',  ( 15.40903463028481113, 31.32187500034139305, -47.42413220539094709 ) ) ;
#5863=CARTESIAN_POINT ( 'NONE',  ( -40.34137639590981195, 38.12187500034139731, 29.30972558990012189 ) ) ;
#5869=CARTESIAN_POINT ( 'NONE',  ( 30.81806926056964002, 42.55937500034139020, 42.41743335407646498 ) ) ;
#5870=VERTEX_POINT ( 'NONE', #5137 ) ;
#5871=CARTESIAN_POINT ( 'NONE',  ( 40.45084971874737789, 30.58125000068279675, 29.38926261462365375 ) ) ;
#5874=CARTESIAN_POINT ( 'NONE',  ( 9.631387414534489405E-15, 42.42187500034140157, 52.43083105670540789 ) ) ;
#5877=CARTESIAN_POINT ( 'NONE',  ( 49.86468353125001585, 22.82187500034138949, 16.20201782572375038 ) ) ;
#5884=CARTESIAN_POINT ( 'NONE',  ( 49.86468353125000164, 44.92187500034140157, -6.106662507704105588E-15 ) ) ;
#5885=CARTESIAN_POINT ( 'NONE',  ( 7.513064459987437071E-14, 42.28125000068280315, 50.00000000000000000 ) ) ;
#5900=EDGE_CURVE ( 'NONE', #14296, #12805, #15927, .T. ) ;
#5901=EDGE_CURVE ( 'NONE', #3842, #5010, #6297, .T. ) ;
#5902=CARTESIAN_POINT ( 'NONE',  ( 15.45084971874737789, 42.38125000068279746, 47.55282581475767500 ) ) ;
#5903=CARTESIAN_POINT ( 'NONE',  ( 15.45084971874737789, 36.60000000000000142, 47.55282581475767500 ) ) ;
#5905=CARTESIAN_POINT ( 'NONE',  ( -40.34137639590981905, 33.65937500034139873, -29.30972558990011478 ) ) ;
#5910=CARTESIAN_POINT ( 'NONE',  ( -40.45084971874737789, 45.58125000068280031, -29.38926261462365730 ) ) ;
#5915=DIRECTION ( 'NONE',  ( 0.000000000000000000, 0.000000000000000000, -1.000000000000000000 ) ) ;
#5919=DIRECTION ( 'NONE',  ( 0.000000000000000000, 0.000000000000000000, -1.000000000000000000 ) ) ;
#5922=CARTESIAN_POINT ( 'NONE',  ( 1.293669679204937499E-13, 39.50000000000000711, -50.00000000000000000 ) ) ;
#5924=CARTESIAN_POINT ( 'NONE',  ( -50.00000000000000000, 42.00000000000000000, 0.000000000000000000 ) ) ;
#5926=FACE_OUTER_BOUND ( 'NONE', #16365, .T. ) ;
#5928=CARTESIAN_POINT ( 'NONE',  ( 30.90169943749474157, 25.30000000000000071, -42.53254041760200721 ) ) ;
#5932=VECTOR ( 'NONE', #16339, 1000.000000000000000 ) ;
#5933=CARTESIAN_POINT ( 'NONE',  ( -3.210462471511496205E-15, 25.35937500034139802, -52.43083105670540789 ) ) ;
#5936=CARTESIAN_POINT ( 'NONE',  ( -15.40903463028480580, 38.25937500034140015, 47.42413220539094709 ) ) ;
#5937=CARTESIAN_POINT ( 'NONE',  ( -1.240322475938754499E-13, 40.28125000068280315, 50.00000000000000000 ) ) ;
#5944=CARTESIAN_POINT ( 'NONE',  ( -3.210462471511496205E-15, 33.42187500034140157, -52.43083105670540789 ) ) ;
#5946=CARTESIAN_POINT ( 'NONE',  ( 40.45084971874737079, 33.20000000000000284, -29.38926261462366440 ) ) ;
#5949=CARTESIAN_POINT ( 'NONE',  ( 15.40903463028481113, 39.32187500034140015, -47.42413220539094709 ) ) ;
#5952=CARTESIAN_POINT ( 'NONE',  ( 15.40903463028482356, 44.45937500034139589, 47.42413220539093999 ) ) ;
#5954=CARTESIAN_POINT ( 'NONE',  ( -49.99999999999999289, 21.88125000068280102, 16.24598481164533226 ) ) ;
#5955=TOROIDAL_SURFACE ( 'NONE', #3020, 63.16733765196516970, 2.000000000000000000 ) ;
#5956=ORIENTED_EDGE ( 'NONE', *, *, #3807, .F. ) ;
#5958=CARTESIAN_POINT ( 'NONE',  ( 30.81806926056962936, 39.22187500034139873, -42.41743335407646498 ) ) ;
#5961=CARTESIAN_POINT ( 'NONE',  ( -49.86468353125000164, 21.92187500034139802, 0.000000000000000000 ) ) ;
#5967=EDGE_LOOP ( 'NONE', ( #3123, #4918 ) ) ;
#5968=CARTESIAN_POINT ( 'NONE',  ( 9.631387414534489405E-15, 34.42187500034138736, 52.43083105670540789 ) ) ;
#5973=FACE_OUTER_BOUND ( 'NONE', #10821, .T. ) ;
#5974=CARTESIAN_POINT ( 'NONE',  ( -40.45084971874737789, 49.80000000000000426, -29.38926261462365730 ) ) ;
#5979=FACE_OUTER_BOUND ( 'NONE', #11781, .T. ) ;
#5983=CARTESIAN_POINT ( 'NONE',  ( 40.45084971874737079, 42.98125000068279888, -29.38926261462366440 ) ) ;
#5988=CARTESIAN_POINT ( 'NONE',  ( 15.40903463028481113, 31.25937500034140015, -47.42413220539094709 ) ) ;
#5990=CARTESIAN_POINT ( 'NONE',  ( -30.90169943749473447, 48.08125000068279320, 42.53254041760200721 ) ) ;
#5993=CARTESIAN_POINT ( 'NONE',  ( 15.45084971874736723, 41.18125000068280173, -47.55282581475768211 ) ) ;
#5995=ORIENTED_EDGE ( 'NONE', *, *, #14415, .F. ) ;
#5997=DIRECTION ( 'NONE',  ( -0.000000000000000000, -1.000000000000000000, -0.000000000000000000 ) ) ;
#5999=DIRECTION ( 'NONE',  ( 0.000000000000000000, 0.000000000000000000, -1.000000000000000000 ) ) ;
#6001=DIRECTION ( 'NONE',  ( 0.000000000000000000, 0.000000000000000000, -1.000000000000000000 ) ) ;
#6009=CARTESIAN_POINT ( 'NONE',  ( 9.657523855033129090E-15, 30.50000000000000000, 52.57311121191334990 ) ) ;
#6011=CARTESIAN_POINT ( 'NONE',  ( -30.90169943749473447, 44.30000000000000426, 42.53254041760200721 ) ) ;
#6020=CARTESIAN_POINT ( 'NONE',  ( -30.81806926056962226, 34.15937500034139163, 42.41743335407647919 ) ) ;
#6029=CARTESIAN_POINT ( 'NONE',  ( 49.86468353125000164, 32.92187500034139447, -6.106662507704105588E-15 ) ) ;
#6033=CARTESIAN_POINT ( 'NONE',  ( 49.86468353125000164, 40.92187500034139447, -6.106662507704105588E-15 ) ) ;
#6037=CARTESIAN_POINT ( 'NONE',  ( -40.34137639590981195, 44.05937500034139731, 29.30972558990012189 ) ) ;
#6041=CARTESIAN_POINT ( 'NONE',  ( -40.45084971874737079, 21.98125000068279888, 29.38926261462367151 ) ) ;
#6044=CARTESIAN_POINT ( 'NONE',  ( -3.210462471511496205E-15, 35.42187500034140157, -52.43083105670540789 ) ) ;
#6046=CARTESIAN_POINT ( 'NONE',  ( 7.919222016226875382, 41.44874571845315359, -49.99999999999997158 ) ) ;
#6047=CARTESIAN_POINT ( 'NONE',  ( 40.34137639590981195, 23.12187500034139731, -29.30972558990011834 ) ) ;
#6054=ORIENTED_EDGE ( 'NONE', *, *, #7538, .F. ) ;
#6055=CARTESIAN_POINT ( 'NONE',  ( 30.81806926056962936, 37.22187500034139873, -42.41743335407647209 ) ) ;
#6056=CARTESIAN_POINT ( 'NONE',  ( -30.90169943749474513, 31.48125000068279533, -42.53254041760200721 ) ) ;
#6068=CARTESIAN_POINT ( 'NONE',  ( -40.45084971874737079, 30.20000000000000284, 29.38926261462367151 ) ) ;
#6078=CARTESIAN_POINT ( 'NONE',  ( 49.86468353124999453, 26.95937500034139944, -16.20201782572376459 ) ) ;
#6082=CARTESIAN_POINT ( 'NONE',  ( 15.45084971874736723, 43.18125000068280173, -47.55282581475768211 ) ) ;
#6086=CARTESIAN_POINT ( 'NONE',  ( 30.90169943749473802, 39.08125000068280031, -42.53254041760200721 ) ) ;
#6098=CARTESIAN_POINT ( 'NONE',  ( -3.219174618344376363E-15, 27.50000000000000355, -52.57311121191334990 ) ) ;
#6100=CARTESIAN_POINT ( 'NONE',  ( -40.34137639590981905, 43.65937500034139163, -29.30972558990011478 ) ) ;
#6105=CARTESIAN_POINT ( 'NONE',  ( 9.631387414534489405E-15, 32.35937500034139447, 52.43083105670540789 ) ) ;
#6109=CARTESIAN_POINT ( 'NONE',  ( 40.45084971874737789, 44.58125000068280031, 29.38926261462365375 ) ) ;
#6116=CARTESIAN_POINT ( 'NONE',  ( -49.86468353125000164, 35.92187500034140157, 0.000000000000000000 ) ) ;
#6120=CARTESIAN_POINT ( 'NONE',  ( 40.34137639590981195, 41.05937500034139731, -29.30972558990011834 ) ) ;
#6122=CARTESIAN_POINT ( 'NONE',  ( -30.90169943749474868, 21.48125000068279533, -42.53254041760200721 ) ) ;
#6130=CARTESIAN_POINT ( 'NONE',  ( 9.631387414534489405E-15, 22.42187500034139802, 52.43083105670540789 ) ) ;
#6134=CARTESIAN_POINT ( 'NONE',  ( 15.40903463028482356, 36.52187500034139589, 47.42413220539093999 ) ) ;
#6135=CARTESIAN_POINT ( 'NONE',  ( 6.123233995736766085E-15, 51.99999999999999289, 50.00000000000000000 ) ) ;
#6146=DIRECTION ( 'NONE',  ( -0.000000000000000000, -1.000000000000000000, -0.000000000000000000 ) ) ;
#6148=CARTESIAN_POINT ( 'NONE',  ( -7.919222016226688865, 33.55125428154685352, -50.00000000000003553 ) ) ;
#6151=CARTESIAN_POINT ( 'NONE',  ( 30.81806926056962936, 25.15937500034139518, -42.41743335407647209 ) ) ;
#6153=ORIENTED_EDGE ( 'NONE', *, *, #13021, .T. ) ;
#6154=ORIENTED_EDGE ( 'NONE', *, *, #7135, .T. ) ;
#6155=CARTESIAN_POINT ( 'NONE',  ( 9.657523855033129090E-15, 38.28125000068279604, 52.57311121191334990 ) ) ;
#6162=CARTESIAN_POINT ( 'NONE',  ( 40.45084971874737789, 26.58125000068279675, 29.38926261462365375 ) ) ;
#6170=CARTESIAN_POINT ( 'NONE',  ( -40.45084971874737079, 30.20000000000000284, 29.38926261462367151 ) ) ;
#6173=CARTESIAN_POINT ( 'NONE',  ( 40.34137639590981195, 43.05937500034139731, -29.30972558990011834 ) ) ;
#6179=CARTESIAN_POINT ( 'NONE',  ( -40.34137639590981905, 37.65937500034139873, -29.30972558990011478 ) ) ;
#6182=CARTESIAN_POINT ( 'NONE',  ( 47.34572995173812160, 25.00000000000000000, -15.64827527265554785 ) ) ;
#6183=FACE_OUTER_BOUND ( 'NONE', #1060, .T. ) ;
#6191=CARTESIAN_POINT ( 'NONE',  ( 15.40903463028482356, 40.52187500034139589, 47.42413220539093999 ) ) ;
#6196=CARTESIAN_POINT ( 'NONE',  ( 15.40903463028481113, 43.25937500034139305, -47.42413220539094709 ) ) ;
#6197=EDGE_LOOP ( 'NONE', ( #3102, #6231, #1681, #7927 ) ) ;
#6199=CARTESIAN_POINT ( 'NONE',  ( 30.90169943749475578, 26.48125000068279888, 42.53254041760200010 ) ) ;
#6206=CARTESIAN_POINT ( 'NONE',  ( -49.86468353124999453, 23.82187500034139305, -16.20201782572375393 ) ) ;
#6212=CARTESIAN_POINT ( 'NONE',  ( -49.86468353124999453, 34.02187500034140299, 16.20201782572377525 ) ) ;
#6213=CARTESIAN_POINT ( 'NONE',  ( 1.293669679204937499E-13, 41.28125000068279604, -50.00000000000000000 ) ) ;
#6229=CARTESIAN_POINT ( 'NONE',  ( -15.40903463028480580, 24.25937500034139660, 47.42413220539094709 ) ) ;
#6230=CARTESIAN_POINT ( 'NONE',  ( -49.99999999999999289, 47.68125000068280173, -16.24598481164531449 ) ) ;
#6231=ORIENTED_EDGE ( 'NONE', *, *, #8648, .T. ) ;
#6232=ORIENTED_EDGE ( 'NONE', *, *, #3067, .T. ) ;
#6234=CARTESIAN_POINT ( 'NONE',  ( -40.45084971874737079, 35.98125000068279888, 29.38926261462367151 ) ) ;
#6236=DIRECTION ( 'NONE',  ( 0.000000000000000000, 1.000000000000000000, 0.000000000000000000 ) ) ;
#6237=ORIENTED_EDGE ( 'NONE', *, *, #15346, .F. ) ;
#6248=CARTESIAN_POINT ( 'NONE',  ( -2.547328955960238000E-13, 32.50000000000000000, 49.99999999999999289 ) ) ;
#6250=CARTESIAN_POINT ( 'NONE',  ( -49.99999999999999289, 21.90000000000000568, -16.24598481164531449 ) ) ;
#6254=CARTESIAN_POINT ( 'NONE',  ( -15.40903463028481646, 43.45937500034139589, -47.42413220539093999 ) ) ;
#6256=CARTESIAN_POINT ( 'NONE',  ( 0.000000000000000000, 193.4213562373095385, -50.00000000000000000 ) ) ;
#6261=CARTESIAN_POINT ( 'NONE',  ( 40.34137639590981195, 29.05937500034139376, -29.30972558990011834 ) ) ;
#6263=CARTESIAN_POINT ( 'NONE',  ( 30.90169943749473802, 41.08125000068280031, -42.53254041760200721 ) ) ;
#6265=CARTESIAN_POINT ( 'NONE',  ( 47.55097084096160387, 25.00000000000000000, -15.01398062572901893 ) ) ;
#6266=CARTESIAN_POINT ( 'NONE',  ( 50.00000000000000711, 30.68125000068279462, 16.24598481164530739 ) ) ;
#6271=CARTESIAN_POINT ( 'NONE',  ( -7.919222016226816763, 29.33250428222964601, -49.99999999999999289 ) ) ;
#6275=CARTESIAN_POINT ( 'NONE',  ( 49.86468353125000164, 28.92187500034139802, -6.106662507704105588E-15 ) ) ;
#6279=( BOUNDED_CURVE ( )  B_SPLINE_CURVE ( 2, ( #2346, #12570, #11091, #6263, #9921, #8423, #4693, #12495, #13486, #3601, #2255, #16154, #5937 ),
 .UNSPECIFIED., .F., .F. ) 
 B_SPLINE_CURVE_WITH_KNOTS ( ( 3, 2, 2, 2, 2, 2, 3 ),
 ( 0.2833333333333333814, 0.2866666666666666807, 0.2933333333333333348, 0.2999999999999999889, 0.3066666666666666430, 0.3133333333333333526, 0.3166666666666667074 ),
 .UNSPECIFIED. ) 
 CURVE ( )  GEOMETRIC_REPRESENTATION_ITEM ( )  RATIONAL_B_SPLINE_CURVE ( ( 0.9755282581475768211, 0.9755282581475770431, 1.000000000000000000, 0.9510565162951535312, 1.000000000000000000, 0.9510565162951535312, 1.000000000000000000, 0.9510565162951535312, 1.000000000000000000, 0.9510565162951535312, 1.000000000000000000, 0.9755282581475765991, 0.9755282581475768211 ) ) 
 REPRESENTATION_ITEM ( '' )  );
#6281=CARTESIAN_POINT ( 'NONE',  ( 15.40903463028482356, 34.45937500034139589, 47.42413220539093999 ) ) ;
#6283=CARTESIAN_POINT ( 'NONE',  ( -40.34137639590981905, 45.65937500034139873, -29.30972558990011478 ) ) ;
#6286=VECTOR ( 'NONE', #11486, 1000.000000000000000 ) ;
#6287=CARTESIAN_POINT ( 'NONE',  ( -30.81806926056963292, 23.62187500034139731, -42.41743335407647209 ) ) ;
#6292=CARTESIAN_POINT ( 'NONE',  ( -50.00000000000000000, 46.00000000000000000, 0.000000000000000000 ) ) ;
#6297=CIRCLE ( 'NONE', #11608, 62.25100647794772613 ) ;
#6299=CARTESIAN_POINT ( 'NONE',  ( -15.40903463028480580, 38.32187500034140015, 47.42413220539094709 ) ) ;
#6310=SURFACE_SIDE_STYLE ('',( #15178 ) ) ;
#6314=CARTESIAN_POINT ( 'NONE',  ( -40.45084971874737789, 39.80000000000000426, -29.38926261462365730 ) ) ;
#6315=CARTESIAN_POINT ( 'NONE',  ( 8.446640517145639571E-15, 28.28125000068279959, 50.00000000000000000 ) ) ;
#6319=CARTESIAN_POINT ( 'NONE',  ( -49.86468353124999453, 27.75937500034139660, -16.20201782572375393 ) ) ;
#6326=ADVANCED_FACE ( 'NONE', ( #9596 ), #14524, .F. ) ;
#6328=CARTESIAN_POINT ( 'NONE',  ( 30.90169943749475223, 28.70000000000000284, 42.53254041760199300 ) ) ;
#6336=CARTESIAN_POINT ( 'NONE',  ( 0.000000000000000000, 54.00000000000000711, 0.000000000000000000 ) ) ;
#6338=CARTESIAN_POINT ( 'NONE',  ( 30.90169943749474157, 21.30000000000000426, -42.53254041760200721 ) ) ;
#6341=CARTESIAN_POINT ( 'NONE',  ( 15.40903463028481113, 41.25937500034139305, -47.42413220539094709 ) ) ;
#6346=CARTESIAN_POINT ( 'NONE',  ( 40.34137639590981905, 26.65937500034139518, 29.30972558990010768 ) ) ;
#6347=DIRECTION ( 'NONE',  ( -1.000000000000000000, 0.000000000000000000, 0.000000000000000000 ) ) ;
#6350=CARTESIAN_POINT ( 'NONE',  ( 47.60088917010805432, 25.00000000000000711, -14.85495851097663333 ) ) ;
#6351=CARTESIAN_POINT ( 'NONE',  ( -40.34137639590981195, 36.12187500034139731, 29.30972558990012189 ) ) ;
#6361=CARTESIAN_POINT ( 'NONE',  ( -15.40903463028480580, 28.32187500034139660, 47.42413220539094709 ) ) ;
#6365=CARTESIAN_POINT ( 'NONE',  ( -49.86468353124999453, 35.75937500034139305, -16.20201782572375393 ) ) ;
#6368=CARTESIAN_POINT ( 'NONE',  ( -40.34137639590981905, 47.65937500034139873, -29.30972558990011478 ) ) ;
#6370=CARTESIAN_POINT ( 'NONE',  ( -30.81806926056963292, 21.62187500034139376, -42.41743335407647209 ) ) ;
#6375=CARTESIAN_POINT ( 'NONE',  ( 30.81806926056964002, 20.62187500034139020, 42.41743335407647209 ) ) ;
#6376=ADVANCED_FACE ( 'NONE', ( #7187 ), #10249, .T. ) ;
#6383=DIRECTION ( 'NONE',  ( 0.000000000000000000, 1.000000000000000000, 0.000000000000000000 ) ) ;
#6385=VERTEX_POINT ( 'NONE', #3850 ) ;
#6388=DIRECTION ( 'NONE',  ( 0.000000000000000000, 1.000000000000000000, 0.000000000000000000 ) ) ;
#6390=SURFACE_STYLE_USAGE ( .BOTH. , #6310 ) ;
#6397=CARTESIAN_POINT ( 'NONE',  ( -40.34137639590981195, 22.05937500034139731, 29.30972558990012189 ) ) ;
#6402=CARTESIAN_POINT ( 'NONE',  ( -2.445080149700054274E-14, 46.50000000000000711, 50.00000000000000000 ) ) ;
#6404=CARTESIAN_POINT ( 'NONE',  ( -7.919222016226816763, 27.55125428154684641, -49.99999999999999289 ) ) ;
#6414=CARTESIAN_POINT ( 'NONE',  ( -40.45084971874737789, 21.80000000000000071, -29.38926261462365730 ) ) ;
#6419=CARTESIAN_POINT ( 'NONE',  ( 30.81806926056962936, 45.15937500034139873, -42.41743335407647209 ) ) ;
#6424=CARTESIAN_POINT ( 'NONE',  ( -49.86468353125000164, 25.85937500034139802, 0.000000000000000000 ) ) ;
#6428=CARTESIAN_POINT ( 'NONE',  ( 47.44954343046539691, 25.00000000000000000, -15.33151233206056041 ) ) ;
#6429=CARTESIAN_POINT ( 'NONE',  ( -49.86468353124999453, 35.82187500034139305, -16.20201782572375393 ) ) ;
#6431=CARTESIAN_POINT ( 'NONE',  ( 40.45084971874737079, 30.98125000068279888, -29.38926261462366440 ) ) ;
#6433=FACE_OUTER_BOUND ( 'NONE', #16228, .T. ) ;
#6438=CARTESIAN_POINT ( 'NONE',  ( 49.86468353125001585, 30.82187500034139660, 16.20201782572375038 ) ) ;
#6440=ORIENTED_EDGE ( 'NONE', *, *, #10727, .T. ) ;
#6444=CARTESIAN_POINT ( 'NONE',  ( 9.631387414534489405E-15, 36.35937500034140157, 52.43083105670540789 ) ) ;
#6448=CARTESIAN_POINT ( 'NONE',  ( -49.86468353125000164, 49.85937500034139447, 0.000000000000000000 ) ) ;
#6450=CARTESIAN_POINT ( 'NONE',  ( 49.86468353124999453, 27.02187500034139589, -16.20201782572376459 ) ) ;
#6456=CARTESIAN_POINT ( 'NONE',  ( 49.99999999999999289, 45.10000000000000853, -16.24598481164532160 ) ) ;
#6459=CARTESIAN_POINT ( 'NONE',  ( -3.210462471511496205E-15, 49.42187500034138736, -52.43083105670540789 ) ) ;
#6462=ORIENTED_EDGE ( 'NONE', *, *, #13945, .F. ) ;
#6468=CARTESIAN_POINT ( 'NONE',  ( -30.81806926056962226, 48.22187500034139163, 42.41743335407647209 ) ) ;
#6475=DIRECTION ( 'NONE',  ( -0.000000000000000000, -1.000000000000000000, -0.000000000000000000 ) ) ;
#6477=CARTESIAN_POINT ( 'NONE',  ( -30.81806926056963292, 47.62187500034139731, -42.41743335407647209 ) ) ;
#6490=CARTESIAN_POINT ( 'NONE',  ( 30.90169943749473802, 27.08125000068280031, -42.53254041760200721 ) ) ;
#6496=CARTESIAN_POINT ( 'NONE',  ( -15.45084971874736368, 22.39999999999999858, 47.55282581475768211 ) ) ;
#6497=EDGE_CURVE ( 'NONE', #1275, #305, #6820, .T. ) ;
#6501=CARTESIAN_POINT ( 'NONE',  ( 9.631387414534489405E-15, 40.35937500034139447, 52.43083105670540789 ) ) ;
#6505=CARTESIAN_POINT ( 'NONE',  ( -49.86468353125000164, 31.85937500034139447, 0.000000000000000000 ) ) ;
#6510=CARTESIAN_POINT ( 'NONE',  ( 46.96694430692144095, 25.00000000000000000, -16.75173377947149689 ) ) ;
#6511=CARTESIAN_POINT ( 'NONE',  ( -15.40903463028481646, 33.52187500034140299, -47.42413220539093999 ) ) ;
#6515=CARTESIAN_POINT ( 'NONE',  ( 0.000000000000000000, 193.4213562373095385, 0.000000000000000000 ) ) ;
#6520=CARTESIAN_POINT ( 'NONE',  ( -30.81806926056963292, 33.62187500034139731, -42.41743335407647209 ) ) ;
#6525=CARTESIAN_POINT ( 'NONE',  ( -15.40903463028480580, 34.25937500034139305, 47.42413220539094709 ) ) ;
#6529=CARTESIAN_POINT ( 'NONE',  ( -30.81806926056962226, 48.15937500034139873, 42.41743335407647919 ) ) ;
#6531=CARTESIAN_POINT ( 'NONE',  ( 49.86468353125001585, 24.82187500034139305, 16.20201782572375038 ) ) ;
#6537=CARTESIAN_POINT ( 'NONE',  ( 15.45084971874736723, 47.40000000000000568, -47.55282581475768211 ) ) ;
#6538=EDGE_CURVE ( 'NONE', #7158, #11087, #13, .T. ) ;
#6547=VERTEX_POINT ( 'NONE', #7674 ) ;
#6551=CARTESIAN_POINT ( 'NONE',  ( 30.90169943749475578, 36.48125000068279888, 42.53254041760200010 ) ) ;
#6553=ORIENTED_EDGE ( 'NONE', *, *, #14934, .T. ) ;
#6557=CARTESIAN_POINT ( 'NONE',  ( -15.40903463028481646, 45.52187500034139589, -47.42413220539093999 ) ) ;
#6559=ADVANCED_FACE ( 'NONE', ( #6433 ), #12745, .F. ) ;
#6560=DIRECTION ( 'NONE',  ( -0.000000000000000000, -1.000000000000000000, -0.000000000000000000 ) ) ;
#6566=VECTOR ( 'NONE', #8975, 1000.000000000000000 ) ;
#6569=ORIENTED_EDGE ( 'NONE', *, *, #9105, .F. ) ;
#6570=CARTESIAN_POINT ( 'NONE',  ( -49.86468353124999453, 46.02187500034140299, 16.20201782572377525 ) ) ;
#6576=DIRECTION ( 'NONE',  ( -0.000000000000000000, -1.000000000000000000, -0.000000000000000000 ) ) ;
#6579=( BOUNDED_CURVE ( )  B_SPLINE_CURVE ( 2, ( #7146, #3308, #8375, #12282, #6068, #10806, #14854, #8615, #13450, #9554, #8537, #12123, #7309 ),
 .UNSPECIFIED., .F., .T. ) 
 B_SPLINE_CURVE_WITH_KNOTS ( ( 3, 2, 2, 2, 2, 2, 3 ),
 ( 0.6500000000000000222, 0.6533333333333333215, 0.6600000000000000311, 0.6666666666666666297, 0.6733333333333333393, 0.6800000000000000488, 0.6833333333333333481 ),
 .UNSPECIFIED. ) 
 CURVE ( )  GEOMETRIC_REPRESENTATION_ITEM ( )  RATIONAL_B_SPLINE_CURVE ( ( 0.9755282581475768211, 0.9755282581475771542, 1.000000000000000000, 0.9510565162951535312, 1.000000000000000000, 0.9510565162951535312, 1.000000000000000000, 0.9510565162951535312, 1.000000000000000000, 0.9510565162951535312, 1.000000000000000000, 0.9755282581475768211, 0.9755282581475768211 ) ) 
 REPRESENTATION_ITEM ( '' )  );
#6580=CARTESIAN_POINT ( 'NONE',  ( -30.90169943749474513, 27.70000000000000284, -42.53254041760200721 ) ) ;
#6583=CARTESIAN_POINT ( 'NONE',  ( 50.00000000000000000, 48.78125000068279604, -6.123233995736766085E-15 ) ) ;
#6591=CARTESIAN_POINT ( 'NONE',  ( 15.45084971874736723, 23.40000000000000213, -47.55282581475768211 ) ) ;
#6595=CARTESIAN_POINT ( 'NONE',  ( 49.86468353125001585, 40.75937500034138594, 16.20201782572375038 ) ) ;
#6597=FACE_OUTER_BOUND ( 'NONE', #14278, .T. ) ;
#6599=CARTESIAN_POINT ( 'NONE',  ( -30.81806926056963292, 29.55937500034139376, -42.41743335407647209 ) ) ;
#6604=CARTESIAN_POINT ( 'NONE',  ( -30.81806926056963292, 33.62187500034139731, -42.41743335407646498 ) ) ;
#6612=CARTESIAN_POINT ( 'NONE',  ( -30.81806926056962226, 34.22187500034139873, 42.41743335407647919 ) ) ;
#6614=ORIENTED_EDGE ( 'NONE', *, *, #7560, .F. ) ;
#6616=CARTESIAN_POINT ( 'NONE',  ( 49.86468353125000164, 38.85937500034139447, -6.106662507704105588E-15 ) ) ;
#6619=CARTESIAN_POINT ( 'NONE',  ( -15.40903463028480580, 46.25937500034140015, 47.42413220539094709 ) ) ;
#6621=CARTESIAN_POINT ( 'NONE',  ( 40.34137639590981905, 26.72187500034139518, 29.30972558990010768 ) ) ;
#6626=CARTESIAN_POINT ( 'NONE',  ( -3.111920190527341144E-15, 25.28125000068279604, -50.00000000000000000 ) ) ;
#6627=( BOUNDED_CURVE ( )  B_SPLINE_CURVE ( 2, ( #4164, #9474, #6831, #1650, #10643, #15695, #15531, #11959, #7059, #636, #1814, #9233, #7976 ),
 .UNSPECIFIED., .F., .F. ) 
 B_SPLINE_CURVE_WITH_KNOTS ( ( 3, 2, 2, 2, 2, 2, 3 ),
 ( 0.1166666666666666685, 0.1199999999999999956, 0.1266666666666666774, 0.1333333333333333315, 0.1400000000000000133, 0.1466666666666666674, 0.1499999999999999944 ),
 .UNSPECIFIED. ) 
 CURVE ( )  GEOMETRIC_REPRESENTATION_ITEM ( )  RATIONAL_B_SPLINE_CURVE ( ( 0.9755282581475768211, 0.9755282581475768211, 1.000000000000000000, 0.9510565162951535312, 1.000000000000000000, 0.9510565162951535312, 1.000000000000000000, 0.9510565162951535312, 1.000000000000000000, 0.9510565162951535312, 1.000000000000000000, 0.9755282581475768211, 0.9755282581475768211 ) ) 
 REPRESENTATION_ITEM ( '' )  );
#6629=CARTESIAN_POINT ( 'NONE',  ( 30.90169943749475578, 38.70000000000000284, 42.53254041760200010 ) ) ;
#6638=CARTESIAN_POINT ( 'NONE',  ( 50.00000000000000711, 34.68125000068279462, 16.24598481164530739 ) ) ;
#6644=CARTESIAN_POINT ( 'NONE',  ( -15.40903463028480580, 46.32187500034140015, 47.42413220539094709 ) ) ;
#6646=DIRECTION ( 'NONE',  ( -0.000000000000000000, -1.000000000000000000, -0.000000000000000000 ) ) ;
#6650=CARTESIAN_POINT ( 'NONE',  ( 7.919222016226693306, 34.33250428222964246, 50.00000000000003553 ) ) ;
#6654=CARTESIAN_POINT ( 'NONE',  ( 49.86468353125001585, 46.82187500034139305, 16.20201782572375038 ) ) ;
#6661=CARTESIAN_POINT ( 'NONE',  ( 40.45084971874737789, 28.80000000000000426, 29.38926261462365375 ) ) ;
#6669=CARTESIAN_POINT ( 'NONE',  ( -3.111920190527341144E-15, 27.28125000068279604, -50.00000000000000000 ) ) ;
#6673=CARTESIAN_POINT ( 'NONE',  ( 0.000000000000000000, 193.4213562373095385, -50.00000000000000000 ) ) ;
#6674=VERTEX_POINT ( 'NONE', #1993 ) ;
#6675=CARTESIAN_POINT ( 'NONE',  ( 15.40903463028481113, 39.25937500034140015, -47.42413220539094709 ) ) ;
#6677=CARTESIAN_POINT ( 'NONE',  ( -50.00000000000000000, 49.78125000068280315, 0.000000000000000000 ) ) ;
#6679=CARTESIAN_POINT ( 'NONE',  ( 30.81806926056964002, 20.55937500034139376, 42.41743335407647209 ) ) ;
#6686=CARTESIAN_POINT ( 'NONE',  ( -49.86468353124999453, 28.02187500034139589, 16.20201782572377169 ) ) ;
#6692=CARTESIAN_POINT ( 'NONE',  ( -40.45084971874737789, 37.79999999999999716, -29.38926261462365730 ) ) ;
#6694=CARTESIAN_POINT ( 'NONE',  ( 40.34137639590981195, 27.12187500034139731, -29.30972558990011834 ) ) ;
#6697=CARTESIAN_POINT ( 'NONE',  ( 15.40903463028482356, 32.45937500034138878, 47.42413220539093999 ) ) ;
#6700=CARTESIAN_POINT ( 'NONE',  ( -15.40903463028481646, 41.45937500034140299, -47.42413220539093999 ) ) ;
#6707=CARTESIAN_POINT ( 'NONE',  ( -49.99999999999999289, 38.10000000000000142, 16.24598481164533226 ) ) ;
#6709=CARTESIAN_POINT ( 'NONE',  ( -40.34137639590981905, 45.72187500034139873, -29.30972558990011478 ) ) ;
#6710=EDGE_CURVE ( 'NONE', #305, #11087, #3509, .T. ) ;
#6713=CARTESIAN_POINT ( 'NONE',  ( -40.34137639590981905, 47.65937500034139873, -29.30972558990011478 ) ) ;
#6715=CARTESIAN_POINT ( 'NONE',  ( -15.45084971874736368, 34.18125000068279462, 47.55282581475768211 ) ) ;
#6720=CARTESIAN_POINT ( 'NONE',  ( -2.547328955960238000E-13, 32.28125000068278894, 49.99999999999999289 ) ) ;
#6721=CARTESIAN_POINT ( 'NONE',  ( -40.34137639590981905, 47.72187500034139873, -29.30972558990011478 ) ) ;
#6728=CARTESIAN_POINT ( 'NONE',  ( 0.000000000000000000, 193.4213562373095385, 0.000000000000000000 ) ) ;
#6733=CARTESIAN_POINT ( 'NONE',  ( -30.81806926056963292, 45.62187500034139020, -42.41743335407647209 ) ) ;
#6736=CARTESIAN_POINT ( 'NONE',  ( -30.90169943749473447, 26.29999999999999716, 42.53254041760200721 ) ) ;
#6742=CARTESIAN_POINT ( 'NONE',  ( 6.123233995736766085E-15, 193.4213562373095385, 50.00000000000000000 ) ) ;
#6746=DIRECTION ( 'NONE',  ( 0.000000000000000000, -0.000000000000000000, 1.000000000000000000 ) ) ;
#6754=EDGE_CURVE ( 'NONE', #15993, #5627, #15968, .T. ) ;
#6758=CARTESIAN_POINT ( 'NONE',  ( -49.86468353124999453, 35.75937500034140015, -16.20201782572375393 ) ) ;
#6759=ORIENTED_EDGE ( 'NONE', *, *, #14415, .T. ) ;
#6762=CARTESIAN_POINT ( 'NONE',  ( 49.99999999999999289, 46.88125000068279036, -16.24598481164532160 ) ) ;
#6764=CARTESIAN_POINT ( 'NONE',  ( 9.631387414534489405E-15, 22.35937500034139802, 52.43083105670540789 ) ) ;
#6769=CARTESIAN_POINT ( 'NONE',  ( 15.40903463028481113, 29.32187500034139660, -47.42413220539094709 ) ) ;
#6775=DIRECTION ( 'NONE',  ( 0.000000000000000000, 0.000000000000000000, -1.000000000000000000 ) ) ;
#6777=CARTESIAN_POINT ( 'NONE',  ( -40.45084971874737079, 36.20000000000000284, 29.38926261462367151 ) ) ;
#6781=CARTESIAN_POINT ( 'NONE',  ( -49.86468353124999453, 29.95937500034139589, 16.20201782572377169 ) ) ;
#6784=CARTESIAN_POINT ( 'NONE',  ( -15.40903463028480580, 42.25937500034139305, 47.42413220539094709 ) ) ;
#6787=CARTESIAN_POINT ( 'NONE',  ( 15.40903463028482356, 20.52187500034139589, 47.42413220539093999 ) ) ;
#6792=CARTESIAN_POINT ( 'NONE',  ( 15.45084971874736723, 43.39999999999999858, -47.55282581475768211 ) ) ;
#6794=CARTESIAN_POINT ( 'NONE',  ( 40.34137639590981905, 46.72187500034139873, 29.30972558990010768 ) ) ;
#6799=CARTESIAN_POINT ( 'NONE',  ( -49.99999999999999289, 31.68125000068279462, -16.24598481164531449 ) ) ;
#6805=CARTESIAN_POINT ( 'NONE',  ( 40.34137639590981195, 47.12187500034140442, -29.30972558990011834 ) ) ;
#6807=DIRECTION ( 'NONE',  ( 0.000000000000000000, 1.000000000000000000, 0.000000000000000000 ) ) ;
#6816=AXIS2_PLACEMENT_3D ( 'NONE', #4136, #6646, #12400 ) ;
#6817=CARTESIAN_POINT ( 'NONE',  ( -40.34137639590981195, 20.05937500034139731, 29.30972558990012189 ) ) ;
#6820=( BOUNDED_CURVE ( )  B_SPLINE_CURVE ( 2, ( #7505, #15312, #13893, #12576, #2509, #4953, #2428, #7588, #3933, #7832, #10013, #8915, #9004 ),
 .UNSPECIFIED., .F., .F. ) 
 B_SPLINE_CURVE_WITH_KNOTS ( ( 3, 2, 2, 2, 2, 2, 3 ),
 ( 0.2166666666666666741, 0.2200000000000000011, 0.2266666666666666552, 0.2333333333333333370, 0.2399999999999999911, 0.2466666666666666730, 0.2500000000000000000 ),
 .UNSPECIFIED. ) 
 CURVE ( )  GEOMETRIC_REPRESENTATION_ITEM ( )  RATIONAL_B_SPLINE_CURVE ( ( 0.9755282581475768211, 0.9755282581475768211, 1.000000000000000000, 0.9510565162951535312, 1.000000000000000000, 0.9510565162951535312, 1.000000000000000000, 0.9510565162951535312, 1.000000000000000000, 0.9510565162951535312, 1.000000000000000000, 0.9755282581475768211, 0.9755282581475765991 ) ) 
 REPRESENTATION_ITEM ( '' )  );
#6822=LINE ( 'NONE', #10560, #2532 ) ;
#6829=CARTESIAN_POINT ( 'NONE',  ( 49.99999999999999289, 48.88125000068280457, -16.24598481164532160 ) ) ;
#6831=CARTESIAN_POINT ( 'NONE',  ( -15.45084971874736368, 46.40000000000000568, 47.55282581475768211 ) ) ;
#6832=CARTESIAN_POINT ( 'NONE',  ( 49.99999999999999289, 49.10000000000000142, -16.24598481164532160 ) ) ;
#6834=CARTESIAN_POINT ( 'NONE',  ( -49.99999999999999289, 37.68125000068279462, -16.24598481164531449 ) ) ;
#6837=DIRECTION ( 'NONE',  ( 0.000000000000000000, 0.000000000000000000, -1.000000000000000000 ) ) ;
#6839=CARTESIAN_POINT ( 'NONE',  ( -15.40903463028480580, 40.25937500034139305, 47.42413220539094709 ) ) ;
#6843=ADVANCED_FACE ( 'NONE', ( #13957 ), #5955, .T. ) ;
#6847=CARTESIAN_POINT ( 'NONE',  ( 30.81806926056962936, 21.15937500034140228, -42.41743335407647209 ) ) ;
#6849=EDGE_CURVE ( 'NONE', #14942, #1352, #2409, .T. ) ;
#6853=CARTESIAN_POINT ( 'NONE',  ( -15.40903463028481646, 25.52187500034139589, -47.42413220539093999 ) ) ;
#6862=CARTESIAN_POINT ( 'NONE',  ( 40.45084971874737079, 33.20000000000000284, -29.38926261462366440 ) ) ;
#6866=CARTESIAN_POINT ( 'NONE',  ( 40.34137639590981195, 31.05937500034139731, -29.30972558990011834 ) ) ;
#6867=ORIENTED_EDGE ( 'NONE', *, *, #9014, .T. ) ;
#6869=CARTESIAN_POINT ( 'NONE',  ( 49.86468353124999453, 42.95937500034139589, -16.20201782572376459 ) ) ;
#6874=CARTESIAN_POINT ( 'NONE',  ( 15.45084971874736723, 41.40000000000000568, -47.55282581475768211 ) ) ;
#6876=CARTESIAN_POINT ( 'NONE',  ( -40.34137639590981195, 44.12187500034139731, 29.30972558990012189 ) ) ;
#6878=CARTESIAN_POINT ( 'NONE',  ( -15.40903463028481646, 47.45937500034139589, -47.42413220539093999 ) ) ;
#6880=CARTESIAN_POINT ( 'NONE',  ( 40.45084971874737789, 32.58125000068280031, 29.38926261462365375 ) ) ;
#6884=CARTESIAN_POINT ( 'NONE',  ( 0.000000000000000000, 25.00000000000000000, 0.000000000000000000 ) ) ;
#6885=CARTESIAN_POINT ( 'NONE',  ( 40.34137639590981905, 42.72187500034139873, 29.30972558990010768 ) ) ;
#6888=CARTESIAN_POINT ( 'NONE',  ( 2.978552182361884590E-14, 47.50000000000000711, -50.00000000000000000 ) ) ;
#6895=CARTESIAN_POINT ( 'NONE',  ( -30.81806926056963292, 43.62187500034139020, -42.41743335407647209 ) ) ;
#6902=VECTOR ( 'NONE', #1649, 1000.000000000000000 ) ;
#6906=CARTESIAN_POINT ( 'NONE',  ( -7.919222016226688865, 33.33250428222964956, -50.00000000000003553 ) ) ;
#6911=CARTESIAN_POINT ( 'NONE',  ( 1.293669679204937499E-13, 37.50000000000000711, -50.00000000000000000 ) ) ;
#6914=CARTESIAN_POINT ( 'NONE',  ( -40.34137639590981195, 32.05937500034139731, 29.30972558990012189 ) ) ;
#6915=VECTOR ( 'NONE', #14360, 1000.000000000000000 ) ;
#6920=CARTESIAN_POINT ( 'NONE',  ( -15.40903463028481646, 23.45937500034139944, -47.42413220539093999 ) ) ;
#6921=ORIENTED_EDGE ( 'NONE', *, *, #6849, .T. ) ;
#6922=CARTESIAN_POINT ( 'NONE',  ( -7.919222016226804328, 48.44874571845315359, 50.00000000000000000 ) ) ;
#6925=CARTESIAN_POINT ( 'NONE',  ( 30.81806926056962936, 29.22187500034139873, -42.41743335407646498 ) ) ;
#6933=CARTESIAN_POINT ( 'NONE',  ( -49.99999999999999289, 37.90000000000000568, -16.24598481164531449 ) ) ;
#6938=CARTESIAN_POINT ( 'NONE',  ( -40.34137639590981905, 27.65937500034139873, -29.30972558990011478 ) ) ;
#6941=CARTESIAN_POINT ( 'NONE',  ( -49.86468353125000164, 39.85937500034139447, 0.000000000000000000 ) ) ;
#6948=CARTESIAN_POINT ( 'NONE',  ( -40.34137639590981195, 28.12187500034139731, 29.30972558990012189 ) ) ;
#6949=CARTESIAN_POINT ( 'NONE',  ( -49.99999999999999289, 42.09999999999999432, 16.24598481164533226 ) ) ;
#6951=CARTESIAN_POINT ( 'NONE',  ( 49.86468353125000164, 46.92187500034139447, -6.106662507704105588E-15 ) ) ;
#6955=CARTESIAN_POINT ( 'NONE',  ( -49.86468353124999453, 45.95937500034138878, 16.20201782572377169 ) ) ;
#6956=ORIENTED_EDGE ( 'NONE', *, *, #11569, .T. ) ;
#6957=CARTESIAN_POINT ( 'NONE',  ( 40.45084971874737079, 32.98125000068279888, -29.38926261462366440 ) ) ;
#6959=ORIENTED_EDGE ( 'NONE', *, *, #4233, .T. ) ;
#6962=CARTESIAN_POINT ( 'NONE',  ( -40.34137639590981905, 39.72187500034139873, -29.30972558990011478 ) ) ;
#6970=ORIENTED_EDGE ( 'NONE', *, *, #14631, .F. ) ;
#6971=CARTESIAN_POINT ( 'NONE',  ( 49.86468353125000164, 40.92187500034139447, -6.106662507704105588E-15 ) ) ;
#6973=EDGE_LOOP ( 'NONE', ( #13097, #11501, #9708 ) ) ;
#6974=DIRECTION ( 'NONE',  ( 0.000000000000000000, 1.000000000000000000, 0.000000000000000000 ) ) ;
#6975=DIRECTION ( 'NONE',  ( 0.000000000000000000, 0.000000000000000000, -1.000000000000000000 ) ) ;
#6986=CARTESIAN_POINT ( 'NONE',  ( 30.81806926056964002, 28.55937500034139731, 42.41743335407647209 ) ) ;
#6991=CARTESIAN_POINT ( 'NONE',  ( 30.90169943749475578, 42.48125000068279888, 42.53254041760200010 ) ) ;
#6993=CARTESIAN_POINT ( 'NONE',  ( 30.81806926056964002, 24.55937500034139376, 42.41743335407647209 ) ) ;
#6994=AXIS2_PLACEMENT_3D ( 'NONE', #9160, #9330, #419 ) ;
#6995=ORIENTED_EDGE ( 'NONE', *, *, #6538, .T. ) ;
#6996=CARTESIAN_POINT ( 'NONE',  ( -7.919222016226816763, 27.33250428222964246, -49.99999999999999289 ) ) ;
#6997=CARTESIAN_POINT ( 'NONE',  ( -49.99999999999999289, 47.89999999999999858, -16.24598481164531449 ) ) ;
#7000=CARTESIAN_POINT ( 'NONE',  ( 30.81806926056964002, 30.62187500034139376, 42.41743335407646498 ) ) ;
#7005=( BOUNDED_CURVE ( )  B_SPLINE_CURVE ( 2, ( #9046, #5155, #10212, #15264, #8965, #14022, #1132, #11219, #4911, #2638, #7713, #3655, #12782 ),
 .UNSPECIFIED., .F., .F. ) 
 B_SPLINE_CURVE_WITH_KNOTS ( ( 3, 2, 2, 2, 2, 2, 3 ),
 ( 0.4500000000000000111, 0.4533333333333333104, 0.4600000000000000200, 0.4666666666666666741, 0.4733333333333333282, 0.4799999999999999822, 0.4833333333333333370 ),
 .UNSPECIFIED. ) 
 CURVE ( )  GEOMETRIC_REPRESENTATION_ITEM ( )  RATIONAL_B_SPLINE_CURVE ( ( 0.9755282581475768211, 0.9755282581475770431, 1.000000000000000000, 0.9510565162951535312, 1.000000000000000000, 0.9510565162951535312, 1.000000000000000000, 0.9510565162951535312, 1.000000000000000000, 0.9510565162951535312, 1.000000000000000000, 0.9755282581475768211, 0.9755282581475768211 ) ) 
 REPRESENTATION_ITEM ( '' )  );
#7007=CARTESIAN_POINT ( 'NONE',  ( 30.90169943749475578, 34.70000000000000995, 42.53254041760200010 ) ) ;
#7012=CARTESIAN_POINT ( 'NONE',  ( 40.34137639590981195, 29.05937500034139376, -29.30972558990011834 ) ) ;
#7014=EDGE_CURVE ( 'NONE', #15272, #4817, #4137, .T. ) ;
#7016=CARTESIAN_POINT ( 'NONE',  ( 15.40903463028481113, 43.25937500034139305, -47.42413220539094709 ) ) ;
#7019=CYLINDRICAL_SURFACE ( 'NONE', #12913, 50.00000000000000000 ) ;
#7023=CARTESIAN_POINT ( 'NONE',  ( -30.81806926056962226, 28.22187500034139873, 42.41743335407647919 ) ) ;
#7026=CARTESIAN_POINT ( 'NONE',  ( 30.81806926056964002, 46.62187500034140442, 42.41743335407647209 ) ) ;
#7032=CARTESIAN_POINT ( 'NONE',  ( 15.40903463028481113, 49.25937500034139305, -47.42413220539094709 ) ) ;
#7035=CARTESIAN_POINT ( 'NONE',  ( -49.99999999999999289, 27.68125000068279462, -16.24598481164531449 ) ) ;
#7039=CARTESIAN_POINT ( 'NONE',  ( -40.34137639590981195, 40.12187500034139731, 29.30972558990012189 ) ) ;
#7046=CARTESIAN_POINT ( 'NONE',  ( -30.81806926056963292, 39.62187500034138310, -42.41743335407647209 ) ) ;
#7059=CARTESIAN_POINT ( 'NONE',  ( -40.45084971874737789, 45.79999999999999716, -29.38926261462365730 ) ) ;
#7064=CARTESIAN_POINT ( 'NONE',  ( -40.45084971874737079, 34.20000000000000284, 29.38926261462367151 ) ) ;
#7068=CARTESIAN_POINT ( 'NONE',  ( 9.631387414534489405E-15, 28.35937500034139802, 52.43083105670540789 ) ) ;
#7072=CARTESIAN_POINT ( 'NONE',  ( 15.45084971874736723, 45.18125000068280173, -47.55282581475768211 ) ) ;
#7082=CARTESIAN_POINT ( 'NONE',  ( -30.90169943749473447, 48.30000000000000426, 42.53254041760200721 ) ) ;
#7087=CARTESIAN_POINT ( 'NONE',  ( 7.857766451448484831E-15, 52.00000000000000711, -63.16733765196516970 ) ) ;
#7093=AXIS2_PLACEMENT_3D ( 'NONE', #7590, #12669, #15315 ) ;
#7094=CARTESIAN_POINT ( 'NONE',  ( 30.90169943749474157, 27.29999999999999716, -42.53254041760200721 ) ) ;
#7101=CARTESIAN_POINT ( 'NONE',  ( -30.81806926056962226, 26.15937500034139163, 42.41743335407647209 ) ) ;
#7104=CARTESIAN_POINT ( 'NONE',  ( -15.40903463028480580, 36.25937500034140015, 47.42413220539094709 ) ) ;
#7108=( BOUNDED_SURFACE ( )  B_SPLINE_SURFACE ( 1, 2, ( 
 ( #5140, #4036, #5308, #1195, #11363, #6459, #7857, #12690, #5222, #16430, #10356, #5064, #12936, #8948, #14004, #1541, #10440, #15496, #10116, #15166, #3795, #8858, #13917, #2536, #7616, #7940, #527, #15913, #13255, #11843, #6951, #1617, #6794, #7026, #4369, #8190, #15827, #4212, #2950, #602, #8098, #4458, #6709, #12081, #4537, #14253, #5550, #13014, #1855, #9434, #2873, #11761, #13331, #1935, #3117, #12006, #5462, #14333, #6876, #9354, #5624, #360, #10528, #15669, #15587, #688, #10849, #9279, #8017, #13092, #1697, #5696, #4291, #14485, #449, #10764, #10612, #14405, #3027, #9523, #13176, #11927, #1783, #3194, #10685, #15740, #14570, #8267, #5782, #2103, #6033, #9851, #12506, #7364, #6191, #855, #12428, #11186, #7191, #7440, #12333, #934, #16241, #2022, #13495, #11010, #5949, #14647, #9600, #13657, #11106, #11266, #12173, #4875, #12252, #9932, #7277, #14985, #5863, #16165, #8511, #4709, #16073, #9771, #7116, #10927, #16323, #4795, #1021, #3276, #14903, #14818, #2180, #3449, #13576, #2357, #3530, #1098, #3614, #8583, #6116, #8345, #14729, #13406, #2266, #8678, #13744, #773, #15990, #4616, #3361, #9679, #8432, #11425, #5199, #13986, #13821, #6612, #2763, #2683, #5122, #2433, #14067, #6520, #15073, #7757, #15318, #7510, #10256, #3938, #8921, #9011, #1269, #3776, #7680, #185, #10340, #2514, #8835, #12750, #10175, #7594, #1347, #15402, #12827, #4021, #18, #12582, #1430, #13899, #11667, #6438, #11499, #96, #5289, #9090, #12672, #2604, #3702, #14147, #8759, #11580, #7839, #12914, #3855, #15225, #1523, #4959, #10019, #1179, #6275, #11347, #16413, #5046, #10099, #15150, #6361, #9171, #15478, #12997, #2854, #5368, #7921, #10424, #263, #4100, #14230, #1600, #6694, #8521, #16093, #14998, #14833, #12519, #16004, #13589, #2369, #2115, #16252, #3289, #866, #12348, #3461, #9613, #16180, #14661, #2194, #7203, #12265, #4810, #11119, #9861, #8359, #1110, #2038, #15928, #14914, #3543, #13428, #7128, #7291, #6206, #8597, #13508, #13672, #12186, #8446, #8690, #6047, #2284, #1032, #5877, #4630, #7376, #9787, #6130, #786, #13756, #4549, #10939, #5961, #9694, #12440, #11200, #14746, #3379, #3633, #7452, #4887, #9943, #11024, #4726, #949, #6375, #2621, #16336, #12933, #12688, #1538, #9104, #7855 ),
 ( #11277, #7614, #15087, #1448, #4975, #8944, #11361, #200, #5138, #10034, #10114, #3791, #2448, #8856, #7696, #11515, #14164, #9027, #3714, #2533, #14081, #12845, #13915, #2780, #14002, #12766, #6537, #8772, #15164, #1285, #11440, #13834, #7526, #15334, #1365, #12598, #1193, #11602, #3953, #10354, #6292, #15416, #33, #16427, #5062, #5305, #10193, #7773, #15246, #6456, #4034, #3872, #111, #5219, #2697, #10279, #5382, #447, #3115, #358, #9432, #8265, #8096, #14331, #15666, #2948, #6792, #15825, #3025, #4456, #8187, #8015, #14483, #10437, #11757, #9521, #4210, #13089, #1695, #6949, #13253, #10762, #5459, #5548, #15493, #11838, #6874, #4289, #4118, #13329, #14568, #4367, #10610, #9189, #15736, #1853, #278, #12003, #525, #14251, #11925, #5620, #9352, #10683, #14402, #10526, #13174, #599, #5694, #9276, #15585, #1780, #3192, #6629, #11680, #2870, #7938, #13012, #1614, #6707, #10592, #6933, #6692, #5762, #11985, #5676, #9258, #1677, #10669, #13152, #9416, #11740, #3254, #3009, #8324, #15895, #14629, #10505, #6777, #11820, #1598, #582, #8080, #1837, #5531, #10746, #343, #14388, #5442, #8248, #15564, #15720, #427, #7007, #11909, #4194, #15648, #4272, #14314, #9338, #14461, #15804, #4519, #4434, #2933, #1760, #9505, #3177, #6862, #9584, #4351, #3095, #13313, #8000, #509, #5604, #8171, #13074, #13239, #14550, #1912, #12063, #665, #10831, #997, #12486, #3678, #5845, #9657, #15049, #16145, #16221, #13389, #14881, #4682, #6009, #9751, #13556, #6170, #9832, #11243, #14964, #14796, #4853, #12153, #2084, #16299, #10987, #3430, #8491, #13719, #3591, #1078, #7173, #12311, #754, #2162, #13634, #11077, #10908, #1997, #4937, #11166, #7254, #15972, #6098, #8649, #7094, #9910, #7336, #4593, #2246, #12406, #912, #2336, #4773, #12234, #3511, #7417, #9991, #16052, #837, #8564, #14707, #3338, #8410, #13478, #5928, #14123, #5268, #1405, #1244, #14045, #13800, #12887, #2662, #12802, #16388, #8813, #1324, #3833, #72, #2412, #10400, #10151, #15457, #6591, #5347, #1156, #13877, #2493, #8734, #7736, #15203, #8986, #12646, #6496, #7490, #5098, #12560, #15375, #6250, #6414, #7570, #2737, #2582, #11321, #6338, #11402, #5022, #8128, #5177, #11553, #11647, #160, #10074, #8899, #10318, #3998, #13961, #241 ) ),
 .UNSPECIFIED., .F., .F., .F. ) 
 B_SPLINE_SURFACE_WITH_KNOTS ( ( 2, 2 ),
 ( 3, 2, 2, 2, 2, 2, 2, 2, 2, 2, 2, 2, 2, 2, 2, 2, 2, 2, 2, 2, 2, 2, 2, 2, 2, 2, 2, 2, 2, 2, 2, 2, 2, 2, 2, 2, 2, 2, 2, 2, 2, 2, 2, 2, 2, 2, 2, 2, 2, 2, 2, 2, 2, 2, 2, 2, 2, 2, 2, 2, 2, 2, 2, 2, 2, 2, 2, 2, 2, 2, 2, 2, 2, 2, 2, 2, 2, 2, 2, 2, 2, 2, 2, 2, 2, 2, 2, 2, 2, 2, 2, 2, 2, 2, 2, 2, 2, 2, 2, 2, 2, 2, 2, 2, 2, 2, 2, 2, 2, 2, 2, 2, 2, 2, 2, 2, 2, 2, 2, 2, 2, 2, 2, 2, 2, 2, 2, 2, 2, 2, 2, 2, 2, 2, 2, 2, 2, 2, 2, 2, 2, 2, 2, 2, 2, 2, 2, 2, 2, 2, 3 ),
 ( 0.000000000000000000, 1.000000000000000000 ),
 ( 0.000000000000000000, 0.006666666666666667095, 0.01333333333333333419, 0.02000000000000000042, 0.02666666666666666838, 0.03333333333333333287, 0.04000000000000000083, 0.04666666666666666879, 0.05333333333333333676, 0.05999999999999999778, 0.06666666666666666574, 0.07333333333333333370, 0.08000000000000000167, 0.08666666666666666963, 0.09333333333333333759, 0.1000000000000000056, 0.1066666666666666735, 0.1133333333333333276, 0.1199999999999999956, 0.1266666666666666774, 0.1333333333333333315, 0.1400000000000000133, 0.1466666666666666674, 0.1533333333333333215, 0.1600000000000000033, 0.1666666666666666574, 0.1733333333333333393, 0.1799999999999999933, 0.1866666666666666752, 0.1933333333333333293, 0.2000000000000000111, 0.2066666666666666652, 0.2133333333333333470, 0.2200000000000000011, 0.2266666666666666552, 0.2333333333333333370, 0.2399999999999999911, 0.2466666666666666730, 0.2533333333333333548, 0.2600000000000000089, 0.2666666666666666630, 0.2733333333333333171, 0.2800000000000000266, 0.2866666666666666807, 0.2933333333333333348, 0.2999999999999999889, 0.3066666666666666430, 0.3133333333333333526, 0.3200000000000000067, 0.3266666666666666607, 0.3333333333333333148, 0.3400000000000000244, 0.3466666666666666785, 0.3533333333333333326, 0.3599999999999999867, 0.3666666666666666408, 0.3733333333333333504, 0.3800000000000000044, 0.3866666666666666585, 0.3933333333333333126, 0.4000000000000000222, 0.4066666666666666763, 0.4133333333333333304, 0.4199999999999999845, 0.4266666666666666941, 0.4333333333333333481, 0.4400000000000000022, 0.4466666666666666563, 0.4533333333333333104, 0.4600000000000000200, 0.4666666666666666741, 0.4733333333333333282, 0.4799999999999999822, 0.4866666666666666918, 0.4933333333333333459, 0.5000000000000000000, 0.5066666666666667096, 0.5133333333333333082, 0.5200000000000000178, 0.5266666666666666163, 0.5333333333333333259, 0.5400000000000000355, 0.5466666666666666341, 0.5533333333333333437, 0.5600000000000000533, 0.5666666666666666519, 0.5733333333333333615, 0.5799999999999999600, 0.5866666666666666696, 0.5933333333333333792, 0.5999999999999999778, 0.6066666666666666874, 0.6133333333333332860, 0.6199999999999999956, 0.6266666666666667052, 0.6333333333333333037, 0.6400000000000000133, 0.6466666666666666119, 0.6533333333333333215, 0.6600000000000000311, 0.6666666666666666297, 0.6733333333333333393, 0.6800000000000000488, 0.6866666666666666474, 0.6933333333333333570, 0.6999999999999999556, 0.7066666666666666652, 0.7133333333333333748, 0.7199999999999999734, 0.7266666666666666829, 0.7333333333333332815, 0.7399999999999999911, 0.7466666666666667007, 0.7533333333333332993, 0.7600000000000000089, 0.7666666666666667185, 0.7733333333333333171, 0.7800000000000000266, 0.7866666666666666252, 0.7933333333333333348, 0.8000000000000000444, 0.8066666666666666430, 0.8133333333333333526, 0.8199999999999999512, 0.8266666666666666607, 0.8333333333333333703, 0.8399999999999999689, 0.8466666666666666785, 0.8533333333333333881, 0.8599999999999999867, 0.8666666666666666963, 0.8733333333333332948, 0.8800000000000000044, 0.8866666666666667140, 0.8933333333333333126, 0.9000000000000000222, 0.9066666666666666208, 0.9133333333333333304, 0.9200000000000000400, 0.9266666666666666385, 0.9333333333333333481, 0.9399999999999999467, 0.9466666666666666563, 0.9533333333333333659, 0.9599999999999999645, 0.9666666666666666741, 0.9733333333333333837, 0.9799999999999999822, 0.9866666666666666918, 0.9933333333333332904, 1.000000000000000000 ),
 .UNSPECIFIED. ) 
 GEOMETRIC_REPRESENTATION_ITEM ( )  RATIONAL_B_SPLINE_SURFACE ( (
 ( 1.000000000000000000, 0.9510565162951535312, 1.000000000000000000, 0.9510565162951535312, 1.000000000000000000, 0.9510565162951535312, 1.000000000000000000, 0.9510565162951535312, 1.000000000000000000, 0.9510565162951535312, 1.000000000000000000, 0.9510565162951535312, 1.000000000000000000, 0.9510565162951535312, 1.000000000000000000, 0.9510565162951535312, 1.000000000000000000, 0.9510565162951535312, 1.000000000000000000, 0.9510565162951535312, 1.000000000000000000, 0.9510565162951535312, 1.000000000000000000, 0.9510565162951535312, 1.000000000000000000, 0.9510565162951535312, 1.000000000000000000, 0.9510565162951535312, 1.000000000000000000, 0.9510565162951535312, 1.000000000000000000, 0.9510565162951535312, 1.000000000000000000, 0.9510565162951535312, 1.000000000000000000, 0.9510565162951535312, 1.000000000000000000, 0.9510565162951535312, 1.000000000000000000, 0.9510565162951535312, 1.000000000000000000, 0.9510565162951535312, 1.000000000000000000, 0.9510565162951535312, 1.000000000000000000, 0.9510565162951535312, 1.000000000000000000, 0.9510565162951535312, 1.000000000000000000, 0.9510565162951535312, 1.000000000000000000, 0.9510565162951535312, 1.000000000000000000, 0.9510565162951535312, 1.000000000000000000, 0.9510565162951535312, 1.000000000000000000, 0.9510565162951535312, 1.000000000000000000, 0.9510565162951535312, 1.000000000000000000, 0.9510565162951535312, 1.000000000000000000, 0.9510565162951535312, 1.000000000000000000, 0.9510565162951535312, 1.000000000000000000, 0.9510565162951535312, 1.000000000000000000, 0.9510565162951535312, 1.000000000000000000, 0.9510565162951535312, 1.000000000000000000, 0.9510565162951535312, 1.000000000000000000, 0.9510565162951535312, 1.000000000000000000, 0.9510565162951535312, 1.000000000000000000, 0.9510565162951535312, 1.000000000000000000, 0.9510565162951535312, 1.000000000000000000, 0.9510565162951535312, 1.000000000000000000, 0.9510565162951535312, 1.000000000000000000, 0.9510565162951535312, 1.000000000000000000, 0.9510565162951535312, 1.000000000000000000, 0.9510565162951535312, 1.000000000000000000, 0.9510565162951535312, 1.000000000000000000, 0.9510565162951535312, 1.000000000000000000, 0.9510565162951535312, 1.000000000000000000, 0.9510565162951535312, 1.000000000000000000, 0.9510565162951535312, 1.000000000000000000, 0.9510565162951535312, 1.000000000000000000, 0.9510565162951535312, 1.000000000000000000, 0.9510565162951535312, 1.000000000000000000, 0.9510565162951535312, 1.000000000000000000, 0.9510565162951535312, 1.000000000000000000, 0.9510565162951535312, 1.000000000000000000, 0.9510565162951535312, 1.000000000000000000, 0.9510565162951535312, 1.000000000000000000, 0.9510565162951535312, 1.000000000000000000, 0.9510565162951535312, 1.000000000000000000, 0.9510565162951535312, 1.000000000000000000, 0.9510565162951535312, 1.000000000000000000, 0.9510565162951535312, 1.000000000000000000, 0.9510565162951535312, 1.000000000000000000, 0.9510565162951535312, 1.000000000000000000, 0.9510565162951535312, 1.000000000000000000, 0.9510565162951535312, 1.000000000000000000, 0.9510565162951535312, 1.000000000000000000, 0.9510565162951535312, 1.000000000000000000, 0.9510565162951535312, 1.000000000000000000, 0.9510565162951535312, 1.000000000000000000, 0.9510565162951535312, 1.000000000000000000, 0.9510565162951535312, 1.000000000000000000, 0.9510565162951535312, 1.000000000000000000, 0.9510565162951535312, 1.000000000000000000, 0.9510565162951535312, 1.000000000000000000, 0.9510565162951535312, 1.000000000000000000, 0.9510565162951535312, 1.000000000000000000, 0.9510565162951535312, 1.000000000000000000, 0.9510565162951535312, 1.000000000000000000, 0.9510565162951535312, 1.000000000000000000, 0.9510565162951535312, 1.000000000000000000, 0.9510565162951535312, 1.000000000000000000, 0.9510565162951535312, 1.000000000000000000, 0.9510565162951535312, 1.000000000000000000, 0.9510565162951535312, 1.000000000000000000, 0.9510565162951535312, 1.000000000000000000, 0.9510565162951535312, 1.000000000000000000, 0.9510565162951535312, 1.000000000000000000, 0.9510565162951535312, 1.000000000000000000, 0.9510565162951535312, 1.000000000000000000, 0.9510565162951535312, 1.000000000000000000, 0.9510565162951535312, 1.000000000000000000, 0.9510565162951535312, 1.000000000000000000, 0.9510565162951535312, 1.000000000000000000, 0.9510565162951535312, 1.000000000000000000, 0.9510565162951535312, 1.000000000000000000, 0.9510565162951535312, 1.000000000000000000, 0.9510565162951535312, 1.000000000000000000, 0.9510565162951535312, 1.000000000000000000, 0.9510565162951535312, 1.000000000000000000, 0.9510565162951535312, 1.000000000000000000, 0.9510565162951535312, 1.000000000000000000, 0.9510565162951535312, 1.000000000000000000, 0.9510565162951535312, 1.000000000000000000, 0.9510565162951535312, 1.000000000000000000, 0.9510565162951535312, 1.000000000000000000, 0.9510565162951535312, 1.000000000000000000, 0.9510565162951535312, 1.000000000000000000, 0.9510565162951535312, 1.000000000000000000, 0.9510565162951535312, 1.000000000000000000, 0.9510565162951535312, 1.000000000000000000, 0.9510565162951535312, 1.000000000000000000, 0.9510565162951535312, 1.000000000000000000, 0.9510565162951535312, 1.000000000000000000, 0.9510565162951535312, 1.000000000000000000, 0.9510565162951535312, 1.000000000000000000, 0.9510565162951535312, 1.000000000000000000, 0.9510565162951535312, 1.000000000000000000, 0.9510565162951535312, 1.000000000000000000, 0.9510565162951535312, 1.000000000000000000, 0.9510565162951535312, 1.000000000000000000, 0.9510565162951535312, 1.000000000000000000, 0.9510565162951535312, 1.000000000000000000, 0.9510565162951535312, 1.000000000000000000, 0.9510565162951535312, 1.000000000000000000, 0.9510565162951535312, 1.000000000000000000, 0.9510565162951535312, 1.000000000000000000, 0.9510565162951535312, 1.000000000000000000, 0.9510565162951535312, 1.000000000000000000, 0.9510565162951535312, 1.000000000000000000, 0.9510565162951535312, 1.000000000000000000, 0.9510565162951535312, 1.000000000000000000, 0.9510565162951535312, 1.000000000000000000, 0.9510565162951535312, 1.000000000000000000, 0.9510565162951535312, 1.000000000000000000, 0.9510565162951535312, 1.000000000000000000, 0.9510565162951535312, 1.000000000000000000, 0.9510565162951535312, 1.000000000000000000, 0.9510565162951535312, 1.000000000000000000, 0.9510565162951535312, 1.000000000000000000, 0.9510565162951535312, 1.000000000000000000, 0.9510565162951535312, 1.000000000000000000, 0.9510565162951535312, 1.000000000000000000, 0.9510565162951535312, 1.000000000000000000, 0.9510565162951535312, 1.000000000000000000, 0.9510565162951535312, 1.000000000000000000, 0.9510565162951535312, 1.000000000000000000, 0.9510565162951535312, 1.000000000000000000),
 ( 1.000000000000000000, 0.9510565162951535312, 1.000000000000000000, 0.9510565162951535312, 1.000000000000000000, 0.9510565162951535312, 1.000000000000000000, 0.9510565162951535312, 1.000000000000000000, 0.9510565162951535312, 1.000000000000000000, 0.9510565162951535312, 1.000000000000000000, 0.9510565162951535312, 1.000000000000000000, 0.9510565162951535312, 1.000000000000000000, 0.9510565162951535312, 1.000000000000000000, 0.9510565162951535312, 1.000000000000000000, 0.9510565162951535312, 1.000000000000000000, 0.9510565162951535312, 1.000000000000000000, 0.9510565162951535312, 1.000000000000000000, 0.9510565162951535312, 1.000000000000000000, 0.9510565162951535312, 1.000000000000000000, 0.9510565162951535312, 1.000000000000000000, 0.9510565162951535312, 1.000000000000000000, 0.9510565162951535312, 1.000000000000000000, 0.9510565162951535312, 1.000000000000000000, 0.9510565162951535312, 1.000000000000000000, 0.9510565162951535312, 1.000000000000000000, 0.9510565162951535312, 1.000000000000000000, 0.9510565162951535312, 1.000000000000000000, 0.9510565162951535312, 1.000000000000000000, 0.9510565162951535312, 1.000000000000000000, 0.9510565162951535312, 1.000000000000000000, 0.9510565162951535312, 1.000000000000000000, 0.9510565162951535312, 1.000000000000000000, 0.9510565162951535312, 1.000000000000000000, 0.9510565162951535312, 1.000000000000000000, 0.9510565162951535312, 1.000000000000000000, 0.9510565162951535312, 1.000000000000000000, 0.9510565162951535312, 1.000000000000000000, 0.9510565162951535312, 1.000000000000000000, 0.9510565162951535312, 1.000000000000000000, 0.9510565162951535312, 1.000000000000000000, 0.9510565162951535312, 1.000000000000000000, 0.9510565162951535312, 1.000000000000000000, 0.9510565162951535312, 1.000000000000000000, 0.9510565162951535312, 1.000000000000000000, 0.9510565162951535312, 1.000000000000000000, 0.9510565162951535312, 1.000000000000000000, 0.9510565162951535312, 1.000000000000000000, 0.9510565162951535312, 1.000000000000000000, 0.9510565162951535312, 1.000000000000000000, 0.9510565162951535312, 1.000000000000000000, 0.9510565162951535312, 1.000000000000000000, 0.9510565162951535312, 1.000000000000000000, 0.9510565162951535312, 1.000000000000000000, 0.9510565162951535312, 1.000000000000000000, 0.9510565162951535312, 1.000000000000000000, 0.9510565162951535312, 1.000000000000000000, 0.9510565162951535312, 1.000000000000000000, 0.9510565162951535312, 1.000000000000000000, 0.9510565162951535312, 1.000000000000000000, 0.9510565162951535312, 1.000000000000000000, 0.9510565162951535312, 1.000000000000000000, 0.9510565162951535312, 1.000000000000000000, 0.9510565162951535312, 1.000000000000000000, 0.9510565162951535312, 1.000000000000000000, 0.9510565162951535312, 1.000000000000000000, 0.9510565162951535312, 1.000000000000000000, 0.9510565162951535312, 1.000000000000000000, 0.9510565162951535312, 1.000000000000000000, 0.9510565162951535312, 1.000000000000000000, 0.9510565162951535312, 1.000000000000000000, 0.9510565162951535312, 1.000000000000000000, 0.9510565162951535312, 1.000000000000000000, 0.9510565162951535312, 1.000000000000000000, 0.9510565162951535312, 1.000000000000000000, 0.9510565162951535312, 1.000000000000000000, 0.9510565162951535312, 1.000000000000000000, 0.9510565162951535312, 1.000000000000000000, 0.9510565162951535312, 1.000000000000000000, 0.9510565162951535312, 1.000000000000000000, 0.9510565162951535312, 1.000000000000000000, 0.9510565162951535312, 1.000000000000000000, 0.9510565162951535312, 1.000000000000000000, 0.9510565162951535312, 1.000000000000000000, 0.9510565162951535312, 1.000000000000000000, 0.9510565162951535312, 1.000000000000000000, 0.9510565162951535312, 1.000000000000000000, 0.9510565162951535312, 1.000000000000000000, 0.9510565162951535312, 1.000000000000000000, 0.9510565162951535312, 1.000000000000000000, 0.9510565162951535312, 1.000000000000000000, 0.9510565162951535312, 1.000000000000000000, 0.9510565162951535312, 1.000000000000000000, 0.9510565162951535312, 1.000000000000000000, 0.9510565162951535312, 1.000000000000000000, 0.9510565162951535312, 1.000000000000000000, 0.9510565162951535312, 1.000000000000000000, 0.9510565162951535312, 1.000000000000000000, 0.9510565162951535312, 1.000000000000000000, 0.9510565162951535312, 1.000000000000000000, 0.9510565162951535312, 1.000000000000000000, 0.9510565162951535312, 1.000000000000000000, 0.9510565162951535312, 1.000000000000000000, 0.9510565162951535312, 1.000000000000000000, 0.9510565162951535312, 1.000000000000000000, 0.9510565162951535312, 1.000000000000000000, 0.9510565162951535312, 1.000000000000000000, 0.9510565162951535312, 1.000000000000000000, 0.9510565162951535312, 1.000000000000000000, 0.9510565162951535312, 1.000000000000000000, 0.9510565162951535312, 1.000000000000000000, 0.9510565162951535312, 1.000000000000000000, 0.9510565162951535312, 1.000000000000000000, 0.9510565162951535312, 1.000000000000000000, 0.9510565162951535312, 1.000000000000000000, 0.9510565162951535312, 1.000000000000000000, 0.9510565162951535312, 1.000000000000000000, 0.9510565162951535312, 1.000000000000000000, 0.9510565162951535312, 1.000000000000000000, 0.9510565162951535312, 1.000000000000000000, 0.9510565162951535312, 1.000000000000000000, 0.9510565162951535312, 1.000000000000000000, 0.9510565162951535312, 1.000000000000000000, 0.9510565162951535312, 1.000000000000000000, 0.9510565162951535312, 1.000000000000000000, 0.9510565162951535312, 1.000000000000000000, 0.9510565162951535312, 1.000000000000000000, 0.9510565162951535312, 1.000000000000000000, 0.9510565162951535312, 1.000000000000000000, 0.9510565162951535312, 1.000000000000000000, 0.9510565162951535312, 1.000000000000000000, 0.9510565162951535312, 1.000000000000000000, 0.9510565162951535312, 1.000000000000000000, 0.9510565162951535312, 1.000000000000000000, 0.9510565162951535312, 1.000000000000000000, 0.9510565162951535312, 1.000000000000000000, 0.9510565162951535312, 1.000000000000000000, 0.9510565162951535312, 1.000000000000000000, 0.9510565162951535312, 1.000000000000000000, 0.9510565162951535312, 1.000000000000000000, 0.9510565162951535312, 1.000000000000000000, 0.9510565162951535312, 1.000000000000000000, 0.9510565162951535312, 1.000000000000000000, 0.9510565162951535312, 1.000000000000000000, 0.9510565162951535312, 1.000000000000000000, 0.9510565162951535312, 1.000000000000000000, 0.9510565162951535312, 1.000000000000000000, 0.9510565162951535312, 1.000000000000000000, 0.9510565162951535312, 1.000000000000000000, 0.9510565162951535312, 1.000000000000000000, 0.9510565162951535312, 1.000000000000000000, 0.9510565162951535312, 1.000000000000000000, 0.9510565162951535312, 1.000000000000000000, 0.9510565162951535312, 1.000000000000000000, 0.9510565162951535312, 1.000000000000000000) ) ) 
 REPRESENTATION_ITEM ( '' )  SURFACE ( )  );
#7109=FACE_OUTER_BOUND ( 'NONE', #15075, .T. ) ;
#7113=CARTESIAN_POINT ( 'NONE',  ( -40.34137639590981905, 29.72187500034139518, -29.30972558990011478 ) ) ;
#7114=CARTESIAN_POINT ( 'NONE',  ( 2.600676159226420495E-13, 33.49999999999999289, -49.99999999999999289 ) ) ;
#7116=CARTESIAN_POINT ( 'NONE',  ( -15.40903463028481646, 37.52187500034139589, -47.42413220539093999 ) ) ;
#7119=CARTESIAN_POINT ( 'NONE',  ( -3.210462471511496205E-15, 41.35937500034138736, -52.43083105670540789 ) ) ;
#7121=CARTESIAN_POINT ( 'NONE',  ( 30.90169943749475578, 32.48125000068280599, 42.53254041760200010 ) ) ;
#7123=ADVANCED_FACE ( 'NONE', ( #14288, #9313 ), #5582, .T. ) ;
#7125=CARTESIAN_POINT ( 'NONE',  ( -49.86468353124999453, 43.82187500034140015, -16.20201782572375393 ) ) ;
#7127=CARTESIAN_POINT ( 'NONE',  ( -3.111920190527341144E-15, 25.50000000000000355, -50.00000000000000000 ) ) ;
#7128=CARTESIAN_POINT ( 'NONE',  ( -49.86468353124999453, 24.02187500034139589, 16.20201782572377525 ) ) ;
#7134=CARTESIAN_POINT ( 'NONE',  ( -3.210462471511496205E-15, 43.42187500034140157, -52.43083105670540789 ) ) ;
#7135=EDGE_CURVE ( 'NONE', #6385, #4580, #10198, .T. ) ;
#7137=ORIENTED_EDGE ( 'NONE', *, *, #3465, .F. ) ;
#7138=VERTEX_POINT ( 'NONE', #6669 ) ;
#7146=CARTESIAN_POINT ( 'NONE',  ( -2.547328955960238000E-13, 30.49999999999999645, 49.99999999999999289 ) ) ;
#7152=CARTESIAN_POINT ( 'NONE',  ( 15.45084971874736723, 43.18125000068280173, -47.55282581475768211 ) ) ;
#7153=CARTESIAN_POINT ( 'NONE',  ( 30.90169943749475223, 36.70000000000000284, 42.53254041760199300 ) ) ;
#7155=CARTESIAN_POINT ( 'NONE',  ( 40.34137639590981905, 28.65937500034139873, 29.30972558990010768 ) ) ;
#7158=VERTEX_POINT ( 'NONE', #1652 ) ;
#7159=CARTESIAN_POINT ( 'NONE',  ( 30.90169943749474157, 43.08125000068280031, -42.53254041760200721 ) ) ;
#7164=CARTESIAN_POINT ( 'NONE',  ( -1.240322475938754499E-13, 38.28125000068280315, 50.00000000000000000 ) ) ;
#7167=CARTESIAN_POINT ( 'NONE',  ( 0.000000000000000000, 193.4213562373095385, 0.000000000000000000 ) ) ;
#7169=CARTESIAN_POINT ( 'NONE',  ( 50.00000000000000000, 39.00000000000000000, -6.123233995736766085E-15 ) ) ;
#7172=CARTESIAN_POINT ( 'NONE',  ( -1.240322475938754499E-13, 36.50000000000000711, 50.00000000000000000 ) ) ;
#7173=CARTESIAN_POINT ( 'NONE',  ( 30.90169943749475578, 28.70000000000000284, 42.53254041760200010 ) ) ;
#7177=CARTESIAN_POINT ( 'NONE',  ( -40.34137639590981905, 25.65937500034139518, -29.30972558990011478 ) ) ;
#7181=CARTESIAN_POINT ( 'NONE',  ( -40.34137639590981195, 34.05937500034139731, 29.30972558990012189 ) ) ;
#7187=FACE_OUTER_BOUND ( 'NONE', #10022, .T. ) ;
#7188=CARTESIAN_POINT ( 'NONE',  ( -15.40903463028481646, 27.52187500034139944, -47.42413220539093999 ) ) ;
#7191=CARTESIAN_POINT ( 'NONE',  ( -40.34137639590981195, 40.12187500034139731, 29.30972558990012189 ) ) ;
#7194=CARTESIAN_POINT ( 'NONE',  ( 30.81806926056964002, 40.55937500034139731, 42.41743335407646498 ) ) ;
#7196=CARTESIAN_POINT ( 'NONE',  ( -40.45084971874737789, 25.58125000068279675, -29.38926261462365730 ) ) ;
#7199=CARTESIAN_POINT ( 'NONE',  ( -49.86468353124999453, 39.82187500034140015, -16.20201782572375393 ) ) ;
#7203=CARTESIAN_POINT ( 'NONE',  ( 30.81806926056962936, 25.22187500034139873, -42.41743335407647209 ) ) ;
#7204=ADVANCED_FACE ( 'NONE', ( #10882 ), #16119, .F. ) ;
#7209=CARTESIAN_POINT ( 'NONE',  ( 15.40903463028482356, 42.52187500034139589, 47.42413220539093999 ) ) ;
#7210=CARTESIAN_POINT ( 'NONE',  ( -40.45084971874737789, 43.58125000068280031, -29.38926261462365730 ) ) ;
#7224=FILL_AREA_STYLE_COLOUR ( '', #12379 ) ;
#7226=CARTESIAN_POINT ( 'NONE',  ( 1.010305842943185372E-14, 272.0000000000000000, 82.49773270518484480 ) ) ;
#7229=ORIENTED_EDGE ( 'NONE', *, *, #13125, .T. ) ;
#7230=ADVANCED_FACE ( 'NONE', ( #10718 ), #8299, .F. ) ;
#7231=CARTESIAN_POINT ( 'NONE',  ( 40.34137639590981905, 32.65937500034139873, 29.30972558990010768 ) ) ;
#7232=CARTESIAN_POINT ( 'NONE',  ( -15.45084971874736368, 48.18125000068280173, 47.55282581475768211 ) ) ;
#7235=CARTESIAN_POINT ( 'NONE',  ( -30.90169943749473802, 42.08125000068279320, 42.53254041760200721 ) ) ;
#7239=CARTESIAN_POINT ( 'NONE',  ( 7.919222016226875382, 39.22999571913595673, -49.99999999999997158 ) ) ;
#7245=CYLINDRICAL_SURFACE ( 'NONE', #3163, 50.00000000000000000 ) ;
#7246=( BOUNDED_CURVE ( )  B_SPLINE_CURVE ( 2, ( #13733, #1589, #15214, #5187, #3843, #14135, #4088, #252, #10242, #2750, #12660, #8909, #10411 ),
 .UNSPECIFIED., .F., .F. ) 
 B_SPLINE_CURVE_WITH_KNOTS ( ( 3, 2, 2, 2, 2, 2, 3 ),
 ( 0.7500000000000000000, 0.7533333333333332993, 0.7600000000000000089, 0.7666666666666667185, 0.7733333333333333171, 0.7800000000000000266, 0.7833333333333333259 ),
 .UNSPECIFIED. ) 
 CURVE ( )  GEOMETRIC_REPRESENTATION_ITEM ( )  RATIONAL_B_SPLINE_CURVE ( ( 0.9755282581475768211, 0.9755282581475768211, 1.000000000000000000, 0.9510565162951535312, 1.000000000000000000, 0.9510565162951535312, 1.000000000000000000, 0.9510565162951535312, 1.000000000000000000, 0.9510565162951535312, 1.000000000000000000, 0.9755282581475768211, 0.9755282581475768211 ) ) 
 REPRESENTATION_ITEM ( '' )  );
#7248=LINE ( 'NONE', #9578, #7861 ) ;
#7254=CARTESIAN_POINT ( 'NONE',  ( -30.90169943749474868, 27.70000000000000284, -42.53254041760200721 ) ) ;
#7257=CARTESIAN_POINT ( 'NONE',  ( 49.86468353124999453, 48.95937500034140299, -16.20201782572376459 ) ) ;
#7258=ORIENTED_EDGE ( 'NONE', *, *, #12310, .F. ) ;
#7264=CARTESIAN_POINT ( 'NONE',  ( 40.34137639590981905, 34.65937500034139873, 29.30972558990010768 ) ) ;
#7273=CARTESIAN_POINT ( 'NONE',  ( 30.81806926056962936, 27.22187500034139518, -42.41743335407647209 ) ) ;
#7277=CARTESIAN_POINT ( 'NONE',  ( -15.40903463028480580, 38.32187500034140015, 47.42413220539094709 ) ) ;
#7279=ORIENTED_EDGE ( 'NONE', *, *, #13105, .T. ) ;
#7280=CARTESIAN_POINT ( 'NONE',  ( 40.34137639590981195, 43.05937500034139731, -29.30972558990011834 ) ) ;
#7283=CARTESIAN_POINT ( 'NONE',  ( -30.90169943749473802, 22.08125000068279320, 42.53254041760200721 ) ) ;
#7287=CARTESIAN_POINT ( 'NONE',  ( -50.00000000000000000, 36.00000000000000711, 0.000000000000000000 ) ) ;
#7288=CARTESIAN_POINT ( 'NONE',  ( 15.40903463028481113, 33.32187500034139305, -47.42413220539094709 ) ) ;
#7291=CARTESIAN_POINT ( 'NONE',  ( -49.86468353125000164, 23.92187500034139447, 0.000000000000000000 ) ) ;
#7297=CARTESIAN_POINT ( 'NONE',  ( -40.34137639590981195, 36.12187500034139731, 29.30972558990012189 ) ) ;
#7305=CARTESIAN_POINT ( 'NONE',  ( -1.240322475938754499E-13, 38.28125000068280315, 50.00000000000000000 ) ) ;
#7309=CARTESIAN_POINT ( 'NONE',  ( -3.111920190527341144E-15, 29.50000000000000000, -50.00000000000000000 ) ) ;
#7311=FILL_AREA_STYLE ('',( #7224 ) ) ;
#7314=ORIENTED_EDGE ( 'NONE', *, *, #9863, .T. ) ;
#7316=CARTESIAN_POINT ( 'NONE',  ( -15.40903463028481646, 23.45937500034139944, -47.42413220539093999 ) ) ;
#7320=CARTESIAN_POINT ( 'NONE',  ( -49.99999999999999289, 41.88125000068279746, 16.24598481164533226 ) ) ;
#7321=CARTESIAN_POINT ( 'NONE',  ( 50.00000000000000000, 47.00000000000000000, -6.123233995736766085E-15 ) ) ;
#7332=CARTESIAN_POINT ( 'NONE',  ( 50.00000000000000000, 36.78125000068280315, -6.123233995736766085E-15 ) ) ;
#7336=CARTESIAN_POINT ( 'NONE',  ( 49.99999999999999289, 27.10000000000000497, -16.24598481164532160 ) ) ;
#7338=CARTESIAN_POINT ( 'NONE',  ( -7.919222016226816763, 43.55125428154684641, -49.99999999999999289 ) ) ;
#7341=CARTESIAN_POINT ( 'NONE',  ( -40.34137639590981195, 48.05937500034139731, 29.30972558990012189 ) ) ;
#7343=CIRCLE ( 'NONE', #2542, 65.15972704814865324 ) ;
#7350=CARTESIAN_POINT ( 'NONE',  ( -40.34137639590981905, 33.65937500034139873, -29.30972558990011478 ) ) ;
#7351=( BOUNDED_CURVE ( )  B_SPLINE_CURVE ( 2, ( #15105, #8790, #9296, #4140, #299, #4227, #221, #11623, #1383, #14350, #2714, #6650, #7958 ),
 .UNSPECIFIED., .F., .F. ) 
 B_SPLINE_CURVE_WITH_KNOTS ( ( 3, 2, 2, 2, 2, 2, 3 ),
 ( 0.4833333333333333370, 0.4866666666666666918, 0.4933333333333333459, 0.5000000000000000000, 0.5066666666666667096, 0.5133333333333333082, 0.5166666666666667185 ),
 .UNSPECIFIED. ) 
 CURVE ( )  GEOMETRIC_REPRESENTATION_ITEM ( )  RATIONAL_B_SPLINE_CURVE ( ( 0.9755282581475768211, 0.9755282581475768211, 1.000000000000000000, 0.9510565162951535312, 1.000000000000000000, 0.9510565162951535312, 1.000000000000000000, 0.9510565162951535312, 1.000000000000000000, 0.9510565162951535312, 1.000000000000000000, 0.9755282581475763770, 0.9755282581475768211 ) ) 
 REPRESENTATION_ITEM ( '' )  );
#7359=DIRECTION ( 'NONE',  ( 0.000000000000000000, 1.000000000000000000, 0.000000000000000000 ) ) ;
#7364=CARTESIAN_POINT ( 'NONE',  ( 30.81806926056964002, 40.62187500034139731, 42.41743335407647209 ) ) ;
#7367=CARTESIAN_POINT ( 'NONE',  ( 9.631387414534489405E-15, 44.35937500034140157, 52.43083105670540789 ) ) ;
#7371=CARTESIAN_POINT ( 'NONE',  ( -40.45084971874737789, 27.58125000068280031, -29.38926261462365730 ) ) ;
#7376=CARTESIAN_POINT ( 'NONE',  ( 30.81806926056964002, 22.62187500034139731, 42.41743335407647209 ) ) ;
#7380=CARTESIAN_POINT ( 'NONE',  ( 40.34137639590981905, 38.72187500034139873, 29.30972558990010768 ) ) ;
#7381=CARTESIAN_POINT ( 'NONE',  ( -49.99999999999999289, 31.88125000068280102, 16.24598481164533226 ) ) ;
#7388=CARTESIAN_POINT ( 'NONE',  ( -2.547328955960238000E-13, 34.28125000068279604, 49.99999999999999289 ) ) ;
#7398=CARTESIAN_POINT ( 'NONE',  ( -30.81806926056963292, 25.55937500034139376, -42.41743335407647209 ) ) ;
#7402=CARTESIAN_POINT ( 'NONE',  ( 40.45084971874737789, 38.58125000068280031, 29.38926261462365375 ) ) ;
#7410=CARTESIAN_POINT ( 'NONE',  ( 50.00000000000000711, 26.68125000068279462, 16.24598481164530739 ) ) ;
#7413=CARTESIAN_POINT ( 'NONE',  ( 15.45084971874736723, 49.39999999999999858, -47.55282581475768211 ) ) ;
#7415=FACE_OUTER_BOUND ( 'NONE', #4440, .T. ) ;
#7417=CARTESIAN_POINT ( 'NONE',  ( -40.45084971874737079, 26.20000000000000284, 29.38926261462367151 ) ) ;
#7420=CARTESIAN_POINT ( 'NONE',  ( -49.86468353124999453, 43.95937500034138878, 16.20201782572377525 ) ) ;
#7422=CARTESIAN_POINT ( 'NONE',  ( -15.40903463028480580, 26.25937500034140015, 47.42413220539094709 ) ) ;
#7425=CARTESIAN_POINT ( 'NONE',  ( -3.210462471511496205E-15, 37.35937500034139447, -52.43083105670540789 ) ) ;
#7427=CARTESIAN_POINT ( 'NONE',  ( -40.45084971874737789, 49.58125000068280031, -29.38926261462365730 ) ) ;
#7428=EDGE_CURVE ( 'NONE', #9397, #1352, #87, .T. ) ;
#7429=CARTESIAN_POINT ( 'NONE',  ( 46.13167797950631410, 24.99999999999999289, -18.93026546213357619 ) ) ;
#7440=CARTESIAN_POINT ( 'NONE',  ( -49.86468353124999453, 40.02187500034140299, 16.20201782572377525 ) ) ;
#7445=CARTESIAN_POINT ( 'NONE',  ( -15.40903463028480580, 44.25937500034140015, 47.42413220539094709 ) ) ;
#7447=CARTESIAN_POINT ( 'NONE',  ( 15.45084971874736723, 25.18125000068279817, -47.55282581475768211 ) ) ;
#7451=CARTESIAN_POINT ( 'NONE',  ( 30.90169943749475223, 30.70000000000000284, 42.53254041760199300 ) ) ;
#7452=CARTESIAN_POINT ( 'NONE',  ( 30.81806926056962936, 21.22187500034139518, -42.41743335407647209 ) ) ;
#7457=CARTESIAN_POINT ( 'NONE',  ( -30.81806926056963292, 37.62187500034139020, -42.41743335407647209 ) ) ;
#7458=CARTESIAN_POINT ( 'NONE',  ( -49.99999999999999289, 41.88125000068279746, 16.24598481164533226 ) ) ;
#7460=ORIENTED_EDGE ( 'NONE', *, *, #12461, .F. ) ;
#7468=CARTESIAN_POINT ( 'NONE',  ( 0.000000000000000000, 272.0000000000000000, 0.000000000000000000 ) ) ;
#7473=CARTESIAN_POINT ( 'NONE',  ( 15.40903463028481113, 25.25937500034139660, -47.42413220539094709 ) ) ;
#7474=ORIENTED_EDGE ( 'NONE', *, *, #13332, .T. ) ;
#7476=CARTESIAN_POINT ( 'NONE',  ( 50.00000000000000711, 38.68125000068280173, 16.24598481164530739 ) ) ;
#7479=ORIENTED_EDGE ( 'NONE', *, *, #1871, .F. ) ;
#7490=CARTESIAN_POINT ( 'NONE',  ( -30.90169943749473802, 22.30000000000000071, 42.53254041760200721 ) ) ;
#7493=CARTESIAN_POINT ( 'NONE',  ( 49.86468353125000164, 42.85937500034140157, -6.106662507704105588E-15 ) ) ;
#7498=CARTESIAN_POINT ( 'NONE',  ( -3.210462471511496205E-15, 29.35937500034139802, -52.43083105670540789 ) ) ;
#7501=CARTESIAN_POINT ( 'NONE',  ( 45.60931600130358987, 25.00000000000000000, -20.15700215907558146 ) ) ;
#7502=CARTESIAN_POINT ( 'NONE',  ( 40.45084971874737789, 46.58125000068280031, 29.38926261462365375 ) ) ;
#7505=CARTESIAN_POINT ( 'NONE',  ( -3.111920190527341144E-15, 43.50000000000000711, -50.00000000000000000 ) ) ;
#7510=CARTESIAN_POINT ( 'NONE',  ( 30.81806926056962936, 33.22187500034139163, -42.41743335407647209 ) ) ;
#7515=CARTESIAN_POINT ( 'NONE',  ( 49.86468353125000164, 34.85937500034140157, -6.106662507704105588E-15 ) ) ;
#7517=ORIENTED_EDGE ( 'NONE', *, *, #1432, .T. ) ;
#7518=CARTESIAN_POINT ( 'NONE',  ( 30.90169943749474157, 27.08125000068280031, -42.53254041760200721 ) ) ;
#7519=CARTESIAN_POINT ( 'NONE',  ( -1.240322475938754499E-13, 40.28125000068280315, 50.00000000000000000 ) ) ;
#7520=CARTESIAN_POINT ( 'NONE',  ( 49.86468353125001585, 26.82187500034138949, 16.20201782572375038 ) ) ;
#7524=CARTESIAN_POINT ( 'NONE',  ( -15.45084971874737256, 25.38125000068279746, -47.55282581475767500 ) ) ;
#7526=CARTESIAN_POINT ( 'NONE',  ( 40.45084971874737789, 46.80000000000000426, 29.38926261462365375 ) ) ;
#7535=CARTESIAN_POINT ( 'NONE',  ( -30.81806926056962226, 38.22187500034139873, 42.41743335407647919 ) ) ;
#7538=EDGE_CURVE ( 'NONE', #6674, #14577, #14967, .T. ) ;
#7545=( NAMED_UNIT ( * ) PLANE_ANGLE_UNIT ( ) SI_UNIT ( $, .RADIAN. ) );
#7548=CARTESIAN_POINT ( 'NONE',  ( -40.45084971874737079, 40.20000000000000284, 29.38926261462367151 ) ) ;
#7549=CYLINDRICAL_SURFACE ( 'NONE', #5290, 50.00000000000000000 ) ;
#7552=CARTESIAN_POINT ( 'NONE',  ( 40.34137639590981195, 23.05937500034139731, -29.30972558990011834 ) ) ;
#7560=EDGE_CURVE ( 'NONE', #4580, #6385, #8348, .T. ) ;
#7562=CARTESIAN_POINT ( 'NONE',  ( -49.99999999999999289, 38.10000000000000142, 16.24598481164533226 ) ) ;
#7570=CARTESIAN_POINT ( 'NONE',  ( -30.90169943749474868, 21.69999999999999574, -42.53254041760200721 ) ) ;
#7573=CARTESIAN_POINT ( 'NONE',  ( -15.40903463028480580, 42.25937500034139305, 47.42413220539094709 ) ) ;
#7575=ORIENTED_EDGE ( 'NONE', *, *, #3392, .F. ) ;
#7577=CARTESIAN_POINT ( 'NONE',  ( 40.34137639590981195, 27.05937500034139731, -29.30972558990011834 ) ) ;
#7579=EDGE_CURVE ( 'NONE', #8369, #9685, #7351, .T. ) ;
#7584=CARTESIAN_POINT ( 'NONE',  ( 48.34710198928263480, 25.00000000000000000, -12.20844498793593580 ) ) ;
#7585=CARTESIAN_POINT ( 'NONE',  ( 49.86468353125000164, 32.92187500034139447, -6.106662507704105588E-15 ) ) ;
#7586=CARTESIAN_POINT ( 'NONE',  ( 15.45084971874736723, 31.18125000068279817, -47.55282581475768211 ) ) ;
#7588=CARTESIAN_POINT ( 'NONE',  ( 50.00000000000000711, 42.89999999999999147, 16.24598481164530739 ) ) ;
#7590=CARTESIAN_POINT ( 'NONE',  ( 0.000000000000000000, 52.00000000000000711, 0.000000000000000000 ) ) ;
#7594=CARTESIAN_POINT ( 'NONE',  ( -49.86468353124999453, 31.82187500034139305, -16.20201782572375393 ) ) ;
#7601=CARTESIAN_POINT ( 'NONE',  ( 40.34137639590981905, 36.65937500034139873, 29.30972558990010768 ) ) ;
#7605=CARTESIAN_POINT ( 'NONE',  ( 40.34137639590981905, 46.65937500034139873, 29.30972558990010768 ) ) ;
#7609=CARTESIAN_POINT ( 'NONE',  ( -49.86468353124999453, 24.02187500034139589, 16.20201782572377525 ) ) ;
#7610=AXIS2_PLACEMENT_3D ( 'NONE', #5611, #8087, #11918 ) ;
#7613=CARTESIAN_POINT ( 'NONE',  ( -15.45084971874736368, 26.18125000068280173, 47.55282581475768211 ) ) ;
#7614=CARTESIAN_POINT ( 'NONE',  ( -49.99999999999999289, 49.89999999999999147, -16.24598481164531449 ) ) ;
#7616=CARTESIAN_POINT ( 'NONE',  ( -15.40903463028481646, 47.52187500034139589, -47.42413220539093999 ) ) ;
#7618=AXIS2_PLACEMENT_3D ( 'NONE', #6515, #8830, #7752 ) ;
#7622=ORIENTED_EDGE ( 'NONE', *, *, #3465, .T. ) ;
#7628=AXIS2_PLACEMENT_3D ( 'NONE', #10986, #13633, #2243 ) ;
#7630=PRESENTATION_STYLE_ASSIGNMENT (( #6390 ) ) ;
#7632=( BOUNDED_CURVE ( )  B_SPLINE_CURVE ( 2, ( #11262, #8917, #7676, #16320, #4955, #5118, #10016, #12747, #16410, #5196, #15070, #6271, #3699 ),
 .UNSPECIFIED., .F., .T. ) 
 B_SPLINE_CURVE_WITH_KNOTS ( ( 3, 2, 2, 2, 2, 2, 3 ),
 ( 0.6500000000000000222, 0.6533333333333333215, 0.6600000000000000311, 0.6666666666666666297, 0.6733333333333333393, 0.6800000000000000488, 0.6833333333333333481 ),
 .UNSPECIFIED. ) 
 CURVE ( )  GEOMETRIC_REPRESENTATION_ITEM ( )  RATIONAL_B_SPLINE_CURVE ( ( 0.9755282581475768211, 0.9755282581475771542, 1.000000000000000000, 0.9510565162951535312, 1.000000000000000000, 0.9510565162951535312, 1.000000000000000000, 0.9510565162951535312, 1.000000000000000000, 0.9510565162951535312, 1.000000000000000000, 0.9755282581475768211, 0.9755282581475768211 ) ) 
 REPRESENTATION_ITEM ( '' )  );
#7638=ADVANCED_FACE ( 'NONE', ( #14183 ), #4053, .T. ) ;
#7641=CARTESIAN_POINT ( 'NONE',  ( 15.40903463028482356, 26.45937500034139589, 47.42413220539093999 ) ) ;
#7648=DIRECTION ( 'NONE',  ( -0.000000000000000000, -1.000000000000000000, -0.000000000000000000 ) ) ;
#7649=CARTESIAN_POINT ( 'NONE',  ( -3.111920190527341144E-15, 27.50000000000000000, -50.00000000000000000 ) ) ;
#7650=CARTESIAN_POINT ( 'NONE',  ( 9.735664389687646693E-15, 252.1309828287255357, -79.49773270518484480 ) ) ;
#7651=DIRECTION ( 'NONE',  ( 0.000000000000000000, 0.000000000000000000, -1.000000000000000000 ) ) ;
#7660=CARTESIAN_POINT ( 'NONE',  ( 49.86468353125000164, 46.85937500034139447, -6.106662507704105588E-15 ) ) ;
#7661=ORIENTED_EDGE ( 'NONE', *, *, #15404, .F. ) ;
#7665=LINE ( 'NONE', #15463, #15580 ) ;
#7666=CARTESIAN_POINT ( 'NONE',  ( 49.86468353125000164, 26.85937500034139802, -6.106662507704105588E-15 ) ) ;
#7670=CARTESIAN_POINT ( 'NONE',  ( 45.11452830843730766, 25.00000000000000355, -21.24066852005663719 ) ) ;
#7671=CARTESIAN_POINT ( 'NONE',  ( 9.631387414534489405E-15, 36.42187500034139447, 52.43083105670540789 ) ) ;
#7672=CARTESIAN_POINT ( 'NONE',  ( -2.445080149700054274E-14, 46.28125000068280315, 50.00000000000000000 ) ) ;
#7674=CARTESIAN_POINT ( 'NONE',  ( 0.000000000000000000, 25.00000000000000000, -50.00000000000000000 ) ) ;
#7676=CARTESIAN_POINT ( 'NONE',  ( -15.45084971874736368, 30.18125000068280173, 47.55282581475768211 ) ) ;
#7680=CARTESIAN_POINT ( 'NONE',  ( 15.40903463028482356, 32.52187500034139589, 47.42413220539093999 ) ) ;
#7685=CARTESIAN_POINT ( 'NONE',  ( -49.86468353125000164, 37.85937500034139447, 0.000000000000000000 ) ) ;
#7687=ORIENTED_EDGE ( 'NONE', *, *, #10887, .T. ) ;
#7689=CARTESIAN_POINT ( 'NONE',  ( 49.86468353124999453, 48.95937500034140299, -16.20201782572376459 ) ) ;
#7691=CARTESIAN_POINT ( 'NONE',  ( -15.40903463028481646, 21.52187500034139589, -47.42413220539093999 ) ) ;
#7696=CARTESIAN_POINT ( 'NONE',  ( 15.45084971874737789, 48.60000000000000142, 47.55282581475767500 ) ) ;
#7708=EDGE_CURVE ( 'NONE', #15481, #15953, #2473, .T. ) ;
#7713=CARTESIAN_POINT ( 'NONE',  ( -15.45084971874737256, 35.38125000068279746, -47.55282581475767500 ) ) ;
#7716=CARTESIAN_POINT ( 'NONE',  ( 15.40903463028482356, 20.45937500034139589, 47.42413220539093999 ) ) ;
#7717=PRODUCT ( 'Heavy Glass Blender Jar Body', 'Heavy Glass Blender Jar Body', '', ( #15605 ) ) ;
#7720=ADVANCED_FACE ( 'NONE', ( #1631 ), #12952, .T. ) ;
#7728=CYLINDRICAL_SURFACE ( 'NONE', #15568, 50.00000000000000000 ) ;
#7735=EDGE_CURVE ( 'NONE', #14050, #1840, #1960, .T. ) ;
#7736=CARTESIAN_POINT ( 'NONE',  ( 40.45084971874737789, 22.80000000000000071, 29.38926261462365375 ) ) ;
#7739=CARTESIAN_POINT ( 'NONE',  ( -15.40903463028481646, 39.45937500034139589, -47.42413220539093999 ) ) ;
#7740=VERTEX_POINT ( 'NONE', #14993 ) ;
#7743=CARTESIAN_POINT ( 'NONE',  ( 15.40903463028482356, 28.45937500034139589, 47.42413220539093999 ) ) ;
#7748=CARTESIAN_POINT ( 'NONE',  ( 47.07787634996847714, 25.00000000000000000, -16.43739640347052955 ) ) ;
#7749=CARTESIAN_POINT ( 'NONE',  ( -40.34137639590981905, 31.72187500034139873, -29.30972558990011478 ) ) ;
#7750=CARTESIAN_POINT ( 'NONE',  ( 0.000000000000000000, 193.4213562373095385, 0.000000000000000000 ) ) ;
#7752=DIRECTION ( 'NONE',  ( 0.000000000000000000, 0.000000000000000000, -1.000000000000000000 ) ) ;
#7757=CARTESIAN_POINT ( 'NONE',  ( -3.210462471511496205E-15, 33.42187500034140157, -52.43083105670540789 ) ) ;
#7759=VERTEX_POINT ( 'NONE', #7519 ) ;
#7761=CARTESIAN_POINT ( 'NONE',  ( -49.86468353124999453, 37.95937500034139589, 16.20201782572377169 ) ) ;
#7765=CARTESIAN_POINT ( 'NONE',  ( 49.86468353125000164, 46.85937500034139447, -6.106662507704105588E-15 ) ) ;
#7768=CARTESIAN_POINT ( 'NONE',  ( -49.86468353124999453, 26.02187500034139944, 16.20201782572377525 ) ) ;
#7773=CARTESIAN_POINT ( 'NONE',  ( 30.90169943749474157, 45.29999999999999005, -42.53254041760200721 ) ) ;
#7779=CARTESIAN_POINT ( 'NONE',  ( 0.000000000000000000, 272.0000000000000000, 0.000000000000000000 ) ) ;
#7782=CARTESIAN_POINT ( 'NONE',  ( 30.90169943749474157, 37.08125000068279320, -42.53254041760200721 ) ) ;
#7784=VERTEX_POINT ( 'NONE', #12683 ) ;
#7789=CARTESIAN_POINT ( 'NONE',  ( 15.40903463028482356, 48.52187500034140299, 47.42413220539093999 ) ) ;
#7795=CARTESIAN_POINT ( 'NONE',  ( 5.143516556418884111E-15, 54.99999999999999289, 42.00000000000000711 ) ) ;
#7796=CARTESIAN_POINT ( 'NONE',  ( 30.90169943749475223, 28.48125000068279888, 42.53254041760199300 ) ) ;
#7798=CARTESIAN_POINT ( 'NONE',  ( -15.40903463028480580, 20.25937500034139660, 47.42413220539094709 ) ) ;
#7799=ORIENTED_EDGE ( 'NONE', *, *, #1880, .T. ) ;
#7816=ORIENTED_EDGE ( 'NONE', *, *, #9009, .T. ) ;
#7818=CARTESIAN_POINT ( 'NONE',  ( 40.34137639590981195, 39.05937500034140442, -29.30972558990011834 ) ) ;
#7822=CARTESIAN_POINT ( 'NONE',  ( 15.40903463028481113, 31.25937500034140015, -47.42413220539094709 ) ) ;
#7825=CARTESIAN_POINT ( 'NONE',  ( 6.123233995736766085E-15, 193.4213562373095385, 50.00000000000000000 ) ) ;
#7829=CARTESIAN_POINT ( 'NONE',  ( 49.86468353125000164, 34.92187500034140157, -6.106662507704105588E-15 ) ) ;
#7832=CARTESIAN_POINT ( 'NONE',  ( 30.90169943749475223, 42.69999999999999574, 42.53254041760199300 ) ) ;
#7839=CARTESIAN_POINT ( 'NONE',  ( -40.34137639590981905, 29.72187500034139518, -29.30972558990011478 ) ) ;
#7843=CARTESIAN_POINT ( 'NONE',  ( -15.40903463028481646, 37.45937500034139589, -47.42413220539093999 ) ) ;
#7846=CARTESIAN_POINT ( 'NONE',  ( 49.86468353125001585, 46.75937500034140015, 16.20201782572375038 ) ) ;
#7848=CARTESIAN_POINT ( 'NONE',  ( -40.34137639590981195, 26.12187500034139731, 29.30972558990012189 ) ) ;
#7853=CARTESIAN_POINT ( 'NONE',  ( -40.45084971874737789, 25.58125000068279675, -29.38926261462365730 ) ) ;
#7855=CARTESIAN_POINT ( 'NONE',  ( -49.86468353125000164, 19.92187500034139447, 0.000000000000000000 ) ) ;
#7857=CARTESIAN_POINT ( 'NONE',  ( 15.40903463028481113, 49.32187500034139305, -47.42413220539094709 ) ) ;
#7861=VECTOR ( 'NONE', #576, 1000.000000000000000 ) ;
#7864=CARTESIAN_POINT ( 'NONE',  ( 49.99999999999999289, 34.88125000068279746, -16.24598481164532160 ) ) ;
#7868=DIRECTION ( 'NONE',  ( 0.000000000000000000, 0.000000000000000000, -1.000000000000000000 ) ) ;
#7869=CARTESIAN_POINT ( 'NONE',  ( 15.40903463028481113, 47.32187500034140015, -47.42413220539094709 ) ) ;
#7877=CARTESIAN_POINT ( 'NONE',  ( 40.45084971874737079, 28.98125000068279888, -29.38926261462366440 ) ) ;
#7879=CARTESIAN_POINT ( 'NONE',  ( -30.81806926056962226, 48.22187500034139163, 42.41743335407647919 ) ) ;
#7880=EDGE_CURVE ( 'NONE', #11917, #3234, #15240, .T. ) ;
#7884=VERTEX_POINT ( 'NONE', #272 ) ;
#7892=CARTESIAN_POINT ( 'NONE',  ( 15.45084971874736723, 49.18125000068279462, -47.55282581475768211 ) ) ;
#7898=CARTESIAN_POINT ( 'NONE',  ( -40.45084971874737079, 37.98125000068279888, 29.38926261462367151 ) ) ;
#7902=CARTESIAN_POINT ( 'NONE',  ( -49.86468353125000164, 35.85937500034140157, 0.000000000000000000 ) ) ;
#7904=CARTESIAN_POINT ( 'NONE',  ( 40.45084971874737789, 48.58125000068280031, 29.38926261462365375 ) ) ;
#7906=CARTESIAN_POINT ( 'NONE',  ( 15.40903463028481113, 23.25937500034139660, -47.42413220539094709 ) ) ;
#7911=CARTESIAN_POINT ( 'NONE',  ( -40.34137639590981195, 26.12187500034139731, 29.30972558990012189 ) ) ;
#7921=CARTESIAN_POINT ( 'NONE',  ( -40.34137639590981905, 27.72187500034139873, -29.30972558990011478 ) ) ;
#7926=CARTESIAN_POINT ( 'NONE',  ( 15.40903463028481113, 27.25937500034139660, -47.42413220539094709 ) ) ;
#7927=ORIENTED_EDGE ( 'NONE', *, *, #701, .T. ) ;
#7930=CARTESIAN_POINT ( 'NONE',  ( 30.81806926056964002, 48.55937500034138310, 42.41743335407647209 ) ) ;
#7938=CARTESIAN_POINT ( 'NONE',  ( -15.45084971874736368, 38.40000000000000568, 47.55282581475768211 ) ) ;
#7940=CARTESIAN_POINT ( 'NONE',  ( -3.210462471511496205E-15, 47.42187500034138736, -52.43083105670540789 ) ) ;
#7946=CARTESIAN_POINT ( 'NONE',  ( 15.45084971874737789, 34.38125000068280457, 47.55282581475767500 ) ) ;
#7952=CARTESIAN_POINT ( 'NONE',  ( 15.45084971874736723, 33.18125000068279462, -47.55282581475768211 ) ) ;
#7953=CARTESIAN_POINT ( 'NONE',  ( 30.81806926056962936, 45.22187500034139873, -42.41743335407646498 ) ) ;
#7955=CARTESIAN_POINT ( 'NONE',  ( -40.45084971874737079, 39.98125000068279888, 29.38926261462367151 ) ) ;
#7958=CARTESIAN_POINT ( 'NONE',  ( -2.547328955960238000E-13, 34.28125000068279604, 49.99999999999999289 ) ) ;
#7962=CARTESIAN_POINT ( 'NONE',  ( 15.40903463028482356, 46.52187500034139589, 47.42413220539093999 ) ) ;
#7963=EDGE_LOOP ( 'NONE', ( #15541, #12355, #11633, #10508 ) ) ;
#7966=ORIENTED_EDGE ( 'NONE', *, *, #6754, .F. ) ;
#7969=DIRECTION ( 'NONE',  ( -0.000000000000000000, -1.000000000000000000, -0.000000000000000000 ) ) ;
#7974=CARTESIAN_POINT ( 'NONE',  ( 30.90169943749475223, 48.48125000068279888, 42.53254041760199300 ) ) ;
#7976=CARTESIAN_POINT ( 'NONE',  ( -3.111920190527341144E-15, 45.50000000000000000, -50.00000000000000000 ) ) ;
#7977=DIRECTION ( 'NONE',  ( 0.000000000000000000, 1.000000000000000000, 0.000000000000000000 ) ) ;
#7983=CARTESIAN_POINT ( 'NONE',  ( 30.81806926056962936, 35.15937500034139873, -42.41743335407647209 ) ) ;
#7988=CARTESIAN_POINT ( 'NONE',  ( -30.81806926056962226, 22.15937500034139873, 42.41743335407647919 ) ) ;
#7990=PRODUCT_DEFINITION_SHAPE ( 'NONE', 'NONE',  #9149 ) ;
#7994=CARTESIAN_POINT ( 'NONE',  ( 15.40903463028482356, 26.52187500034139589, 47.42413220539093999 ) ) ;
#8000=CARTESIAN_POINT ( 'NONE',  ( 30.90169943749475578, 32.70000000000000284, 42.53254041760200010 ) ) ;
#8004=CARTESIAN_POINT ( 'NONE',  ( 49.86468353125001585, 28.75937500034139305, 16.20201782572375038 ) ) ;
#8008=CARTESIAN_POINT ( 'NONE',  ( 9.631387414534489405E-15, 42.35937500034140157, 52.43083105670540789 ) ) ;
#8015=CARTESIAN_POINT ( 'NONE',  ( 50.00000000000000711, 42.89999999999999858, 16.24598481164530739 ) ) ;
#8017=CARTESIAN_POINT ( 'NONE',  ( 40.34137639590981195, 43.12187500034139731, -29.30972558990011834 ) ) ;
#8020=CARTESIAN_POINT ( 'NONE',  ( 15.40903463028482356, 46.45937500034139589, 47.42413220539093999 ) ) ;
#8022=CARTESIAN_POINT ( 'NONE',  ( 49.99999999999999289, 30.88125000068279391, -16.24598481164532160 ) ) ;
#8025=CARTESIAN_POINT ( 'NONE',  ( -2.547328955960238000E-13, 30.28125000068279604, 49.99999999999999289 ) ) ;
#8028=CARTESIAN_POINT ( 'NONE',  ( -49.93234176562499727, 49.82031250051209526, 0.000000000000000000 ) ) ;
#8029=CARTESIAN_POINT ( 'NONE',  ( -40.34137639590981195, 48.12187500034139731, 29.30972558990012189 ) ) ;
#8037=CARTESIAN_POINT ( 'NONE',  ( -3.111920190527341144E-15, 45.28125000068279604, -50.00000000000000000 ) ) ;
#8041=CARTESIAN_POINT ( 'NONE',  ( 15.40903463028481113, 49.32187500034139305, -47.42413220539094709 ) ) ;
#8043=CARTESIAN_POINT ( 'NONE',  ( 0.000000000000000000, 55.00000000000000711, 0.000000000000000000 ) ) ;
#8053=CARTESIAN_POINT ( 'NONE',  ( 0.000000000000000000, 55.00000000000000711, 0.000000000000000000 ) ) ;
#8057=CARTESIAN_POINT ( 'NONE',  ( 0.000000000000000000, 193.4213562373095385, -50.00000000000000000 ) ) ;
#8060=( BOUNDED_CURVE ( )  B_SPLINE_CURVE ( 2, ( #8279, #14419, #8112, #11859, #7955, #9449, #11939, #10860, #5475, #1629, #4224, #5634, #12099 ),
 .UNSPECIFIED., .F., .T. ) 
 B_SPLINE_CURVE_WITH_KNOTS ( ( 3, 2, 2, 2, 2, 2, 3 ),
 ( 0.3166666666666667074, 0.3200000000000000067, 0.3266666666666666607, 0.3333333333333333148, 0.3400000000000000244, 0.3466666666666666785, 0.3500000000000000333 ),
 .UNSPECIFIED. ) 
 CURVE ( )  GEOMETRIC_REPRESENTATION_ITEM ( )  RATIONAL_B_SPLINE_CURVE ( ( 0.9755282581475768211, 0.9755282581475770431, 1.000000000000000000, 0.9510565162951535312, 1.000000000000000000, 0.9510565162951535312, 1.000000000000000000, 0.9510565162951535312, 1.000000000000000000, 0.9510565162951535312, 1.000000000000000000, 0.9755282581475765991, 0.9755282581475768211 ) ) 
 REPRESENTATION_ITEM ( '' )  );
#8061=CARTESIAN_POINT ( 'NONE',  ( -40.34137639590981905, 39.65937500034139873, -29.30972558990011478 ) ) ;
#8064=AXIS2_PLACEMENT_3D ( 'NONE', #1576, #7977, #13051 ) ;
#8065=CARTESIAN_POINT ( 'NONE',  ( -49.99999999999999289, 49.68125000068279462, -16.24598481164531449 ) ) ;
#8067=CARTESIAN_POINT ( 'NONE',  ( -15.40903463028481646, 21.45937500034139589, -47.42413220539093999 ) ) ;
#8072=CARTESIAN_POINT ( 'NONE',  ( 49.86468353125000164, 30.92187500034139802, -6.106662507704105588E-15 ) ) ;
#8080=CARTESIAN_POINT ( 'NONE',  ( -40.45084971874737789, 35.79999999999999716, -29.38926261462365730 ) ) ;
#8084=CARTESIAN_POINT ( 'NONE',  ( -49.86468353124999453, 27.95937500034139944, 16.20201782572377169 ) ) ;
#8087=DIRECTION ( 'NONE',  ( 0.000000000000000000, 1.000000000000000000, 0.000000000000000000 ) ) ;
#8088=CARTESIAN_POINT ( 'NONE',  ( -30.81806926056962226, 42.15937500034139163, 42.41743335407647919 ) ) ;
#8091=CARTESIAN_POINT ( 'NONE',  ( -30.81806926056962226, 20.22187500034139163, 42.41743335407647919 ) ) ;
#8096=CARTESIAN_POINT ( 'NONE',  ( -40.45084971874737789, 43.80000000000000426, -29.38926261462365730 ) ) ;
#8098=CARTESIAN_POINT ( 'NONE',  ( -49.86468353125000164, 45.92187500034139447, 0.000000000000000000 ) ) ;
#8101=CARTESIAN_POINT ( 'NONE',  ( -49.86468353124999453, 47.75937500034139305, -16.20201782572375393 ) ) ;
#8103=CARTESIAN_POINT ( 'NONE',  ( -3.219174618344376363E-15, 29.28125000068279604, -52.57311121191334990 ) ) ;
#8109=CARTESIAN_POINT ( 'NONE',  ( 15.40903463028481113, 45.32187500034140015, -47.42413220539094709 ) ) ;
#8112=CARTESIAN_POINT ( 'NONE',  ( -15.45084971874736368, 40.18125000068280173, 47.55282581475768211 ) ) ;
#8120=AXIS2_PLACEMENT_3D ( 'NONE', #1668, #10493, #10823 ) ;
#8121=VERTEX_POINT ( 'NONE', #439 ) ;
#8124=CARTESIAN_POINT ( 'NONE',  ( 9.631387414534489405E-15, 40.42187500034138736, 52.43083105670540789 ) ) ;
#8128=CARTESIAN_POINT ( 'NONE',  ( 50.00000000000000000, 21.00000000000000000, -6.123233995736766085E-15 ) ) ;
#8133=LINE ( 'NONE', #3056, #8490 ) ;
#8135=CIRCLE ( 'NONE', #15278, 63.16733765196516970 ) ;
#8139=CARTESIAN_POINT ( 'NONE',  ( 8.446640517145639571E-15, 48.28125000068279604, 50.00000000000000000 ) ) ;
#8142=DIRECTION ( 'NONE',  ( -0.000000000000000000, -1.000000000000000000, -0.000000000000000000 ) ) ;
#8151=CARTESIAN_POINT ( 'NONE',  ( -15.40903463028480580, 30.25937500034140015, 47.42413220539094709 ) ) ;
#8158=CARTESIAN_POINT ( 'NONE',  ( 15.40903463028482356, 24.45937500034139589, 47.42413220539093999 ) ) ;
#8163=CARTESIAN_POINT ( 'NONE',  ( -3.210462471511496205E-15, 29.42187500034139447, -52.43083105670540789 ) ) ;
#8169=( BOUNDED_CURVE ( )  B_SPLINE_CURVE ( 2, ( #651, #3241, #8314, #746, #1068, #7562, #1315, #13867, #15118, #12633, #8723, #14036, #1235 ),
 .UNSPECIFIED., .F., .T. ) 
 B_SPLINE_CURVE_WITH_KNOTS ( ( 3, 2, 2, 2, 2, 2, 3 ),
 ( 0.3833333333333333592, 0.3866666666666666585, 0.3933333333333333126, 0.4000000000000000222, 0.4066666666666666763, 0.4133333333333333304, 0.4166666666666666852 ),
 .UNSPECIFIED. ) 
 CURVE ( )  GEOMETRIC_REPRESENTATION_ITEM ( )  RATIONAL_B_SPLINE_CURVE ( ( 0.9755282581475768211, 0.9755282581475770431, 1.000000000000000000, 0.9510565162951535312, 1.000000000000000000, 0.9510565162951535312, 1.000000000000000000, 0.9510565162951535312, 1.000000000000000000, 0.9510565162951535312, 1.000000000000000000, 0.9755282581475765991, 0.9755282581475768211 ) ) 
 REPRESENTATION_ITEM ( '' )  );
#8171=CARTESIAN_POINT ( 'NONE',  ( -15.45084971874736368, 32.39999999999999858, 47.55282581475768211 ) ) ;
#8176=CARTESIAN_POINT ( 'NONE',  ( -49.86468353124999453, 31.75937500034140015, -16.20201782572375393 ) ) ;
#8179=CARTESIAN_POINT ( 'NONE',  ( -30.81806926056963292, 41.55937500034139731, -42.41743335407647209 ) ) ;
#8180=EDGE_CURVE ( 'NONE', #5251, #326, #4110, .T. ) ;
#8186=CARTESIAN_POINT ( 'NONE',  ( -3.210462471511496205E-15, 31.42187500034139447, -52.43083105670540789 ) ) ;
#8187=CARTESIAN_POINT ( 'NONE',  ( 50.00000000000000000, 43.00000000000000000, -6.123233995736766085E-15 ) ) ;
#8190=CARTESIAN_POINT ( 'NONE',  ( 9.631387414534489405E-15, 46.42187500034139447, 52.43083105670540789 ) ) ;
#8193=CARTESIAN_POINT ( 'NONE',  ( -15.40903463028480580, 46.25937500034140015, 47.42413220539094709 ) ) ;
#8196=CARTESIAN_POINT ( 'NONE',  ( -15.45084971874737256, 31.38125000068280102, -47.55282581475767500 ) ) ;
#8197=ORIENTED_EDGE ( 'NONE', *, *, #5536, .F. ) ;
#8199=CARTESIAN_POINT ( 'NONE',  ( 7.919222016226940219, 33.22999571913595673, -49.99999999999996447 ) ) ;
#8200=CARTESIAN_POINT ( 'NONE',  ( -30.81806926056962226, 38.22187500034139873, 42.41743335407647209 ) ) ;
#8207=ORIENTED_EDGE ( 'NONE', *, *, #4087, .T. ) ;
#8208=CARTESIAN_POINT ( 'NONE',  ( 40.34137639590981905, 44.72187500034139163, 29.30972558990010768 ) ) ;
#8214=CARTESIAN_POINT ( 'NONE',  ( 0.000000000000000000, 193.4213562373095385, 0.000000000000000000 ) ) ;
#8219=CARTESIAN_POINT ( 'NONE',  ( 0.000000000000000000, 193.4213562373095385, -50.00000000000000000 ) ) ;
#8220=CARTESIAN_POINT ( 'NONE',  ( -15.45084971874736368, 34.18125000068279462, 47.55282581475768211 ) ) ;
#8226=EDGE_CURVE ( 'NONE', #7784, #4024, #1261, .T. ) ;
#8228=CARTESIAN_POINT ( 'NONE',  ( 49.86468353125000164, 28.85937500034139802, -6.106662507704105588E-15 ) ) ;
#8233=CARTESIAN_POINT ( 'NONE',  ( 9.657523855033129090E-15, 46.28125000068279604, 52.57311121191334990 ) ) ;
#8235=CARTESIAN_POINT ( 'NONE',  ( 40.34137639590981905, 24.65937500034139873, 29.30972558990010768 ) ) ;
#8240=CARTESIAN_POINT ( 'NONE',  ( -49.86468353124999453, 27.82187500034139305, -16.20201782572375393 ) ) ;
#8247=EDGE_CURVE ( 'NONE', #10886, #13613, #3847, .T. ) ;
#8248=CARTESIAN_POINT ( 'NONE',  ( 49.99999999999999289, 35.10000000000000853, -16.24598481164532160 ) ) ;
#8250=DIRECTION ( 'NONE',  ( 0.000000000000000000, 0.000000000000000000, -1.000000000000000000 ) ) ;
#8253=UNCERTAINTY_MEASURE_WITH_UNIT (LENGTH_MEASURE( 1.000000000000000082E-05 ), #9805, 'distance_accuracy_value', 'NONE');
#8254=CARTESIAN_POINT ( 'NONE',  ( -40.34137639590981195, 30.05937500034139731, 29.30972558990012189 ) ) ;
#8257=CARTESIAN_POINT ( 'NONE',  ( 49.86468353125001585, 40.75937500034138594, 16.20201782572375038 ) ) ;
#8259=( BOUNDED_CURVE ( )  B_SPLINE_CURVE ( 2, ( #2217, #4830, #7152, #2310, #5983, #11052, #9885, #1970, #3312, #812, #5902, #4494, #15873 ),
 .UNSPECIFIED., .F., .T. ) 
 B_SPLINE_CURVE_WITH_KNOTS ( ( 3, 2, 2, 2, 2, 2, 3 ),
 ( 0.2166666666666666741, 0.2200000000000000011, 0.2266666666666666552, 0.2333333333333333370, 0.2399999999999999911, 0.2466666666666666730, 0.2500000000000000000 ),
 .UNSPECIFIED. ) 
 CURVE ( )  GEOMETRIC_REPRESENTATION_ITEM ( )  RATIONAL_B_SPLINE_CURVE ( ( 0.9755282581475768211, 0.9755282581475768211, 1.000000000000000000, 0.9510565162951535312, 1.000000000000000000, 0.9510565162951535312, 1.000000000000000000, 0.9510565162951535312, 1.000000000000000000, 0.9510565162951535312, 1.000000000000000000, 0.9755282581475768211, 0.9755282581475765991 ) ) 
 REPRESENTATION_ITEM ( '' )  );
#8260=DIRECTION ( 'NONE',  ( 0.000000000000000000, 0.000000000000000000, -1.000000000000000000 ) ) ;
#8264=CARTESIAN_POINT ( 'NONE',  ( -3.210462471511496205E-15, 29.42187500034139092, -52.43083105670540789 ) ) ;
#8265=CARTESIAN_POINT ( 'NONE',  ( -49.99999999999999289, 43.90000000000000568, -16.24598481164531449 ) ) ;
#8267=CARTESIAN_POINT ( 'NONE',  ( 30.81806926056962936, 41.22187500034139873, -42.41743335407647209 ) ) ;
#8271=CARTESIAN_POINT ( 'NONE',  ( 49.86468353125001585, 48.75937500034140015, 16.20201782572375038 ) ) ;
#8274=CARTESIAN_POINT ( 'NONE',  ( -40.45084971874737079, 27.98125000068279888, 29.38926261462367151 ) ) ;
#8277=CARTESIAN_POINT ( 'NONE',  ( -30.81806926056963292, 37.62187500034138310, -42.41743335407646498 ) ) ;
#8279=CARTESIAN_POINT ( 'NONE',  ( -1.240322475938754499E-13, 40.28125000068280315, 50.00000000000000000 ) ) ;
#8285=CARTESIAN_POINT ( 'NONE',  ( 49.86468353125001585, 44.82187500034138594, 16.20201782572375038 ) ) ;
#8292=CARTESIAN_POINT ( 'NONE',  ( 7.594208199954109127E-15, 52.26146722824297797, -62.01141590572476758 ) ) ;
#8297=CARTESIAN_POINT ( 'NONE',  ( -40.45084971874737789, 33.58125000068280031, -29.38926261462365730 ) ) ;
#8298=PRESENTATION_STYLE_ASSIGNMENT (( #12371 ) ) ;
#8299=PLANE ( 'NONE',  #16303 ) ;
#8300=( BOUNDED_CURVE ( )  B_SPLINE_CURVE ( 2, ( #5596, #6922, #5432, #7082, #13303, #14540, #15885, #6997, #13229, #497, #10658, #9249, #3168 ),
 .UNSPECIFIED., .F., .F. ) 
 B_SPLINE_CURVE_WITH_KNOTS ( ( 3, 2, 2, 2, 2, 2, 3 ),
 ( 0.05000000000000000278, 0.05333333333333333676, 0.05999999999999999778, 0.06666666666666666574, 0.07333333333333333370, 0.08000000000000000167, 0.08333333333333334259 ),
 .UNSPECIFIED. ) 
 CURVE ( )  GEOMETRIC_REPRESENTATION_ITEM ( )  RATIONAL_B_SPLINE_CURVE ( ( 0.9755282581475768211, 0.9755282581475768211, 1.000000000000000000, 0.9510565162951535312, 1.000000000000000000, 0.9510565162951535312, 1.000000000000000000, 0.9510565162951535312, 1.000000000000000000, 0.9510565162951535312, 1.000000000000000000, 0.9755282581475767101, 0.9755282581475768211 ) ) 
 REPRESENTATION_ITEM ( '' )  );
#8306=CARTESIAN_POINT ( 'NONE',  ( 15.40903463028481113, 33.25937500034140015, -47.42413220539094709 ) ) ;
#8310=CARTESIAN_POINT ( 'NONE',  ( 40.45084971874737789, 46.58125000068280031, 29.38926261462365375 ) ) ;
#8314=CARTESIAN_POINT ( 'NONE',  ( -15.45084971874736368, 38.40000000000000568, 47.55282581475768211 ) ) ;
#8320=CARTESIAN_POINT ( 'NONE',  ( 50.00000000000000711, 36.68125000068280173, 16.24598481164530739 ) ) ;
#8321=CARTESIAN_POINT ( 'NONE',  ( 0.000000000000000000, 193.4213562373095385, -50.00000000000000000 ) ) ;
#8324=CARTESIAN_POINT ( 'NONE',  ( 15.45084971874737789, 36.60000000000000142, 47.55282581475767500 ) ) ;
#8327=CARTESIAN_POINT ( 'NONE',  ( 15.40903463028481113, 49.25937500034139305, -47.42413220539094709 ) ) ;
#8329=ADVANCED_FACE ( 'NONE', ( #14087 ), #9032, .T. ) ;
#8333=CARTESIAN_POINT ( 'NONE',  ( -49.86468353124999453, 41.75937500034139305, -16.20201782572375393 ) ) ;
#8335=CARTESIAN_POINT ( 'NONE',  ( 0.000000000000000000, 193.4213562373095385, -50.00000000000000000 ) ) ;
#8342=CARTESIAN_POINT ( 'NONE',  ( 15.40903463028482356, 32.52187500034139589, 47.42413220539093999 ) ) ;
#8345=CARTESIAN_POINT ( 'NONE',  ( -49.86468353124999453, 35.82187500034139305, -16.20201782572375393 ) ) ;
#8348=CIRCLE ( 'NONE', #3303, 79.49773270518484480 ) ;
#8350=CARTESIAN_POINT ( 'NONE',  ( -40.34137639590981195, 40.05937500034140442, 29.30972558990012189 ) ) ;
#8352=CARTESIAN_POINT ( 'NONE',  ( 30.90169943749474157, 33.08125000068279320, -42.53254041760200721 ) ) ;
#8353=ORIENTED_EDGE ( 'NONE', *, *, #11096, .T. ) ;
#8354=CARTESIAN_POINT ( 'NONE',  ( -30.90169943749473447, 36.29999999999999716, 42.53254041760200721 ) ) ;
#8355=CARTESIAN_POINT ( 'NONE',  ( 15.40903463028481113, 39.32187500034140015, -47.42413220539094709 ) ) ;
#8359=CARTESIAN_POINT ( 'NONE',  ( 40.34137639590981905, 24.72187500034139873, 29.30972558990010768 ) ) ;
#8365=CARTESIAN_POINT ( 'NONE',  ( 30.81806926056962936, 39.22187500034139873, -42.41743335407647209 ) ) ;
#8369=VERTEX_POINT ( 'NONE', #10286 ) ;
#8375=CARTESIAN_POINT ( 'NONE',  ( -15.45084971874736368, 30.40000000000000213, 47.55282581475768211 ) ) ;
#8387=CARTESIAN_POINT ( 'NONE',  ( -49.86468353124999453, 33.75937500034140015, -16.20201782572375393 ) ) ;
#8388=ORIENTED_EDGE ( 'NONE', *, *, #10990, .F. ) ;
#8391=CARTESIAN_POINT ( 'NONE',  ( -50.00000000000000000, 45.78125000068279604, 0.000000000000000000 ) ) ;
#8394=CARTESIAN_POINT ( 'NONE',  ( 49.99999999999999289, 47.10000000000000142, -16.24598481164532160 ) ) ;
#8398=CARTESIAN_POINT ( 'NONE',  ( 0.000000000000000000, 193.4213562373095385, 0.000000000000000000 ) ) ;
#8410=CARTESIAN_POINT ( 'NONE',  ( -3.219174618344376363E-15, 25.50000000000000355, -52.57311121191334990 ) ) ;
#8413=CARTESIAN_POINT ( 'NONE',  ( 40.34137639590981905, 48.65937500034139873, 29.30972558990010768 ) ) ;
#8416=CARTESIAN_POINT ( 'NONE',  ( 30.81806926056964002, 26.55937500034139376, 42.41743335407646498 ) ) ;
#8419=CARTESIAN_POINT ( 'NONE',  ( 30.81806926056962936, 33.15937500034139873, -42.41743335407647209 ) ) ;
#8422=ADVANCED_FACE ( 'NONE', ( #1939 ), #14573, .T. ) ;
#8423=CARTESIAN_POINT ( 'NONE',  ( 49.99999999999999289, 40.88125000068279746, -16.24598481164532160 ) ) ;
#8425=CIRCLE ( 'NONE', #12137, 82.49773270518484480 ) ;
#8426=CARTESIAN_POINT ( 'NONE',  ( 0.000000000000000000, 193.4213562373095385, 0.000000000000000000 ) ) ;
#8429=CARTESIAN_POINT ( 'NONE',  ( -49.86468353125000164, 31.92187500034139447, 0.000000000000000000 ) ) ;
#8430=CARTESIAN_POINT ( 'NONE',  ( -3.111920190527341144E-15, 29.50000000000000000, -50.00000000000000000 ) ) ;
#8432=CARTESIAN_POINT ( 'NONE',  ( 40.34137639590981905, 34.72187500034139873, 29.30972558990010768 ) ) ;
#8435=VERTEX_POINT ( 'NONE', #9358 ) ;
#8436=CARTESIAN_POINT ( 'NONE',  ( -30.81806926056963292, 39.55937500034140442, -42.41743335407646498 ) ) ;
#8438=CARTESIAN_POINT ( 'NONE',  ( 15.45084971874737789, 22.38125000068280102, 47.55282581475767500 ) ) ;
#8441=CARTESIAN_POINT ( 'NONE',  ( 49.86468353124999453, 41.02187500034139589, -16.20201782572376104 ) ) ;
#8445=EDGE_CURVE ( 'NONE', #7884, #1138, #12439, .T. ) ;
#8446=CARTESIAN_POINT ( 'NONE',  ( 15.40903463028481113, 23.32187500034139660, -47.42413220539094709 ) ) ;
#8452=CARTESIAN_POINT ( 'NONE',  ( 40.34137639590981905, 42.72187500034139873, 29.30972558990010768 ) ) ;
#8453=EDGE_CURVE ( 'NONE', #9685, #1121, #9588, .T. ) ;
#8454=CARTESIAN_POINT ( 'NONE',  ( -7.919222016226838967, 44.22999571913595673, 49.99999999999999289 ) ) ;
#8472=CARTESIAN_POINT ( 'NONE',  ( 40.34137639590981905, 30.65937500034139518, 29.30972558990010768 ) ) ;
#8477=CARTESIAN_POINT ( 'NONE',  ( -30.90169943749474868, 41.48125000068278467, -42.53254041760200721 ) ) ;
#8478=LINE ( 'NONE', #2230, #9162 ) ;
#8486=CARTESIAN_POINT ( 'NONE',  ( 49.99999999999999289, 39.10000000000000142, -16.24598481164532160 ) ) ;
#8487=CARTESIAN_POINT ( 'NONE',  ( 7.513064459987437071E-14, 42.50000000000000000, 50.00000000000000000 ) ) ;
#8489=CARTESIAN_POINT ( 'NONE',  ( 5.755839955992560641E-15, 51.99999999999999289, 47.00000000000000000 ) ) ;
#8490=VECTOR ( 'NONE', #3141, 1000.000000000000000 ) ;
#8491=CARTESIAN_POINT ( 'NONE',  ( 49.99999999999999289, 29.10000000000000142, -16.24598481164532160 ) ) ;
#8493=CARTESIAN_POINT ( 'NONE',  ( -50.00000000000000000, 44.00000000000000711, 0.000000000000000000 ) ) ;
#8500=CARTESIAN_POINT ( 'NONE',  ( 49.86468353124999453, 32.95937500034138168, -16.20201782572376459 ) ) ;
#8508=CARTESIAN_POINT ( 'NONE',  ( 49.86468353125000164, 28.92187500034139802, -6.106662507704105588E-15 ) ) ;
#8511=CARTESIAN_POINT ( 'NONE',  ( -49.86468353125000164, 37.92187500034140157, 0.000000000000000000 ) ) ;
#8514=CARTESIAN_POINT ( 'NONE',  ( -30.81806926056963292, 43.55937500034139731, -42.41743335407646498 ) ) ;
#8516=CARTESIAN_POINT ( 'NONE',  ( -30.90169943749474868, 25.48125000068279888, -42.53254041760200721 ) ) ;
#8519=CARTESIAN_POINT ( 'NONE',  ( 9.631387414534489405E-15, 38.42187500034139447, 52.43083105670540789 ) ) ;
#8521=CARTESIAN_POINT ( 'NONE',  ( 49.86468353124999453, 27.02187500034139589, -16.20201782572376459 ) ) ;
#8526=CARTESIAN_POINT ( 'NONE',  ( -40.34137639590981905, 37.72187500034139873, -29.30972558990011478 ) ) ;
#8528=ORIENTED_EDGE ( 'NONE', *, *, #1725, .F. ) ;
#8530=ORIENTED_EDGE ( 'NONE', *, *, #6497, .F. ) ;
#8537=CARTESIAN_POINT ( 'NONE',  ( -15.45084971874737256, 29.60000000000000142, -47.55282581475767500 ) ) ;
#8540=DIRECTION ( 'NONE',  ( 0.000000000000000000, 0.000000000000000000, -1.000000000000000000 ) ) ;
#8541=DIRECTION ( 'NONE',  ( 1.000000000000000000, 0.000000000000000000, -0.000000000000000000 ) ) ;
#8545=CARTESIAN_POINT ( 'NONE',  ( 15.40903463028481113, 27.25937500034139660, -47.42413220539094709 ) ) ;
#8549=CARTESIAN_POINT ( 'NONE',  ( -40.45084971874737079, 45.98125000068279888, 29.38926261462367151 ) ) ;
#8558=VECTOR ( 'NONE', #2218, 1000.000000000000000 ) ;
#8559=CARTESIAN_POINT ( 'NONE',  ( 40.45084971874737079, 39.19999999999999574, -29.38926261462366440 ) ) ;
#8560=DIRECTION ( 'NONE',  ( 1.000000000000000000, 0.000000000000000000, 0.000000000000000000 ) ) ;
#8564=CARTESIAN_POINT ( 'NONE',  ( -40.45084971874737789, 25.80000000000000071, -29.38926261462365730 ) ) ;
#8567=FACE_OUTER_BOUND ( 'NONE', #13059, .T. ) ;
#8569=CARTESIAN_POINT ( 'NONE',  ( 30.81806926056962936, 25.15937500034139518, -42.41743335407646498 ) ) ;
#8572=CARTESIAN_POINT ( 'NONE',  ( 15.40903463028482356, 32.45937500034138878, 47.42413220539093999 ) ) ;
#8573=CYLINDRICAL_SURFACE ( 'NONE', #16084, 50.00000000000000000 ) ;
#8583=CARTESIAN_POINT ( 'NONE',  ( -49.86468353124999453, 36.02187500034139589, 16.20201782572377525 ) ) ;
#8586=( BOUNDED_CURVE ( )  B_SPLINE_CURVE ( 2, ( #13230, #15639, #1669, #417, #1751, #4262, #15553, #5520, #13381, #9250, #1828, #1987, #14303 ),
 .UNSPECIFIED., .F., .F. ) 
 B_SPLINE_CURVE_WITH_KNOTS ( ( 3, 2, 2, 2, 2, 2, 3 ),
 ( 0.4833333333333333370, 0.4866666666666666918, 0.4933333333333333459, 0.5000000000000000000, 0.5066666666666667096, 0.5133333333333333082, 0.5166666666666667185 ),
 .UNSPECIFIED. ) 
 CURVE ( )  GEOMETRIC_REPRESENTATION_ITEM ( )  RATIONAL_B_SPLINE_CURVE ( ( 0.9755282581475768211, 0.9755282581475768211, 1.000000000000000000, 0.9510565162951535312, 1.000000000000000000, 0.9510565162951535312, 1.000000000000000000, 0.9510565162951535312, 1.000000000000000000, 0.9510565162951535312, 1.000000000000000000, 0.9755282581475763770, 0.9755282581475768211 ) ) 
 REPRESENTATION_ITEM ( '' )  );
#8588=CARTESIAN_POINT ( 'NONE',  ( 30.81806926056962936, 43.15937500034139873, -42.41743335407646498 ) ) ;
#8589=EDGE_LOOP ( 'NONE', ( #12383, #819, #10103, #2165 ) ) ;
#8591=CARTESIAN_POINT ( 'NONE',  ( 40.45084971874737079, 22.98125000068279888, -29.38926261462366440 ) ) ;
#8594=CARTESIAN_POINT ( 'NONE',  ( -15.45084971874736368, 36.39999999999999858, 47.55282581475768211 ) ) ;
#8597=CARTESIAN_POINT ( 'NONE',  ( -40.34137639590981905, 23.72187500034139873, -29.30972558990011478 ) ) ;
#8602=CARTESIAN_POINT ( 'NONE',  ( 30.81806926056964002, 38.62187500034139731, 42.41743335407647209 ) ) ;
#8606=ORIENTED_EDGE ( 'NONE', *, *, #16001, .T. ) ;
#8607=CYLINDRICAL_SURFACE ( 'NONE', #16129, 50.00000000000000000 ) ;
#8608=CYLINDRICAL_SURFACE ( 'NONE', #3870, 50.00000000000000000 ) ;
#8615=CARTESIAN_POINT ( 'NONE',  ( -49.99999999999999289, 29.89999999999999858, -16.24598481164531449 ) ) ;
#8619=EDGE_CURVE ( 'NONE', #10949, #10705, #10913, .T. ) ;
#8620=CARTESIAN_POINT ( 'NONE',  ( 6.123233995736766085E-15, 25.00000000000000000, 50.00000000000000000 ) ) ;
#8621=LINE ( 'NONE', #13777, #8558 ) ;
#8624=VECTOR ( 'NONE', #7648, 1000.000000000000000 ) ;
#8625=CARTESIAN_POINT ( 'NONE',  ( -3.210462471511496205E-15, 27.35937500034139802, -52.43083105670540789 ) ) ;
#8626=CARTESIAN_POINT ( 'NONE',  ( -7.919222016226804328, 48.22999571913595673, 50.00000000000000000 ) ) ;
#8629=ORIENTED_EDGE ( 'NONE', *, *, #5714, .T. ) ;
#8631=CARTESIAN_POINT ( 'NONE',  ( 49.99999999999999289, 36.88125000068279036, -16.24598481164532160 ) ) ;
#8645=CARTESIAN_POINT ( 'NONE',  ( -6.668400408272873429E-15, 49.50000000000000000, -50.00000000000000000 ) ) ;
#8648=EDGE_CURVE ( 'NONE', #1840, #14050, #14717, .T. ) ;
#8649=CARTESIAN_POINT ( 'NONE',  ( 15.45084971874736723, 27.40000000000000213, -47.55282581475768211 ) ) ;
#8653=CARTESIAN_POINT ( 'NONE',  ( -49.86468353124999453, 45.95937500034138878, 16.20201782572377525 ) ) ;
#8662=CARTESIAN_POINT ( 'NONE',  ( 9.631387414534489405E-15, 34.35937500034139447, 52.43083105670540789 ) ) ;
#8667=DIRECTION ( 'NONE',  ( -0.000000000000000000, -1.000000000000000000, -0.000000000000000000 ) ) ;
#8671=VECTOR ( 'NONE', #15204, 1000.000000000000000 ) ;
#8678=CARTESIAN_POINT ( 'NONE',  ( -3.210462471511496205E-15, 35.42187500034140157, -52.43083105670540789 ) ) ;
#8680=ORIENTED_EDGE ( 'NONE', *, *, #5004, .F. ) ;
#8681=CARTESIAN_POINT ( 'NONE',  ( -40.34137639590981905, 45.65937500034139873, -29.30972558990011478 ) ) ;
#8685=CARTESIAN_POINT ( 'NONE',  ( 9.657523855033129090E-15, 26.28125000068279604, 52.57311121191334990 ) ) ;
#8690=CARTESIAN_POINT ( 'NONE',  ( 30.81806926056962936, 23.22187500034139163, -42.41743335407647209 ) ) ;
#8695=CARTESIAN_POINT ( 'NONE',  ( 49.86468353125001585, 34.82187500034140015, 16.20201782572375038 ) ) ;
#8696=CARTESIAN_POINT ( 'NONE',  ( -7.919222016226752814, 41.33250428222964246, -50.00000000000000711 ) ) ;
#8700=ORIENTED_EDGE ( 'NONE', *, *, #1871, .T. ) ;
#8701=CARTESIAN_POINT ( 'NONE',  ( -49.99999999999999289, 32.10000000000000142, 16.24598481164533226 ) ) ;
#8702=CARTESIAN_POINT ( 'NONE',  ( 30.90169943749475223, 44.69999999999999574, 42.53254041760199300 ) ) ;
#8712=DIRECTION ( 'NONE',  ( 0.000000000000000000, 0.000000000000000000, -1.000000000000000000 ) ) ;
#8714=CARTESIAN_POINT ( 'NONE',  ( -30.81806926056963292, 27.55937500034139376, -42.41743335407647209 ) ) ;
#8718=CARTESIAN_POINT ( 'NONE',  ( 49.99999999999999289, 38.88125000068279036, -16.24598481164532160 ) ) ;
#8722=CARTESIAN_POINT ( 'NONE',  ( 40.45084971874737079, 38.98125000068279888, -29.38926261462366440 ) ) ;
#8723=CARTESIAN_POINT ( 'NONE',  ( -15.45084971874737256, 37.60000000000000142, -47.55282581475767500 ) ) ;
#8734=CARTESIAN_POINT ( 'NONE',  ( 50.00000000000000711, 22.90000000000000213, 16.24598481164530739 ) ) ;
#8735=CARTESIAN_POINT ( 'NONE',  ( 0.000000000000000000, 54.99999999999999289, -42.00000000000000711 ) ) ;
#8737=CARTESIAN_POINT ( 'NONE',  ( 30.81806926056962936, 43.15937500034140584, -42.41743335407647209 ) ) ;
#8740=CARTESIAN_POINT ( 'NONE',  ( 0.000000000000000000, 54.99999999999999289, 0.000000000000000000 ) ) ;
#8743=CARTESIAN_POINT ( 'NONE',  ( -40.34137639590981195, 28.05937500034139731, 29.30972558990012189 ) ) ;
#8747=CARTESIAN_POINT ( 'NONE',  ( 45.80914010100575240, 25.00000000000000000, -19.69865795820044951 ) ) ;
#8759=CARTESIAN_POINT ( 'NONE',  ( -49.86468353125000164, 29.92187500034139802, 0.000000000000000000 ) ) ;
#8760=ADVANCED_FACE ( 'NONE', ( #9324, #5592 ), #13223, .F. ) ;
#8762=EDGE_LOOP ( 'NONE', ( #188, #10934, #15058, #11504 ) ) ;
#8763=CARTESIAN_POINT ( 'NONE',  ( 30.81806926056962936, 37.15937500034139163, -42.41743335407646498 ) ) ;
#8766=CARTESIAN_POINT ( 'NONE',  ( -49.99999999999999289, 23.88125000068279746, 16.24598481164533226 ) ) ;
#8768=CARTESIAN_POINT ( 'NONE',  ( 30.81806926056964002, 24.62187500034139731, 42.41743335407647209 ) ) ;
#8772=CARTESIAN_POINT ( 'NONE',  ( 30.90169943749474157, 47.29999999999999716, -42.53254041760200721 ) ) ;
#8779=CARTESIAN_POINT ( 'NONE',  ( -15.40903463028480580, 34.32187500034139305, 47.42413220539094709 ) ) ;
#8782=ORIENTED_EDGE ( 'NONE', *, *, #5722, .T. ) ;
#8788=( BOUNDED_CURVE ( )  B_SPLINE_CURVE ( 2, ( #4668, #9741, #2233, #16211, #4843, #15960, #4763, #9820, #3579, #14617, #1902, #6996, #3417 ),
 .UNSPECIFIED., .F., .T. ) 
 B_SPLINE_CURVE_WITH_KNOTS ( ( 3, 2, 2, 2, 2, 2, 3 ),
 ( 0.7166666666666666741, 0.7199999999999999734, 0.7266666666666666829, 0.7333333333333332815, 0.7399999999999999911, 0.7466666666666667007, 0.7500000000000000000 ),
 .UNSPECIFIED. ) 
 CURVE ( )  GEOMETRIC_REPRESENTATION_ITEM ( )  RATIONAL_B_SPLINE_CURVE ( ( 0.9755282581475768211, 0.9755282581475768211, 1.000000000000000000, 0.9510565162951535312, 1.000000000000000000, 0.9510565162951535312, 1.000000000000000000, 0.9510565162951535312, 1.000000000000000000, 0.9510565162951535312, 1.000000000000000000, 0.9755282581475768211, 0.9755282581475768211 ) ) 
 REPRESENTATION_ITEM ( '' )  );
#8790=CARTESIAN_POINT ( 'NONE',  ( 7.919222016226809657, 35.22999571913594963, -50.00000000000000000 ) ) ;
#8794=ADVANCED_FACE ( 'NONE', ( #6597 ), #5842, .T. ) ;
#8795=CARTESIAN_POINT ( 'NONE',  ( -30.81806926056963292, 23.55937500034139376, -42.41743335407647209 ) ) ;
#8803=CARTESIAN_POINT ( 'NONE',  ( 15.45084971874737789, 38.38125000068279746, 47.55282581475767500 ) ) ;
#8813=CARTESIAN_POINT ( 'NONE',  ( -40.45084971874737079, 24.20000000000000284, 29.38926261462367151 ) ) ;
#8815=CARTESIAN_POINT ( 'NONE',  ( -7.919222016226838967, 44.44874571845315359, 49.99999999999999289 ) ) ;
#8816=CARTESIAN_POINT ( 'NONE',  ( -40.34137639590981905, 41.65937500034139873, -29.30972558990011478 ) ) ;
#8821=CARTESIAN_POINT ( 'NONE',  ( -3.210462471511496205E-15, 27.35937500034139802, -52.43083105670540789 ) ) ;
#8822=VECTOR ( 'NONE', #13131, 1000.000000000000000 ) ;
#8825=CARTESIAN_POINT ( 'NONE',  ( 48.11476475577527623, 25.00000000000000000, -13.09518440664933436 ) ) ;
#8826=CARTESIAN_POINT ( 'NONE',  ( 15.40903463028482356, 32.52187500034139589, 47.42413220539093999 ) ) ;
#8830=DIRECTION ( 'NONE',  ( -0.000000000000000000, -1.000000000000000000, -0.000000000000000000 ) ) ;
#8835=CARTESIAN_POINT ( 'NONE',  ( -40.34137639590981195, 32.12187500034140442, 29.30972558990012189 ) ) ;
#8836=( BOUNDED_CURVE ( )  B_SPLINE_CURVE ( 2, ( #5263, #10393, #7892, #1489, #14284, #6829, #6583, #10641, #3059, #7974, #9063, #15693, #8139 ),
 .UNSPECIFIED., .F., .T. ) 
 B_SPLINE_CURVE_WITH_KNOTS ( ( 3, 2, 2, 2, 2, 2, 3 ),
 ( 0.01666666666666666644, 0.02000000000000000042, 0.02666666666666666838, 0.03333333333333333287, 0.04000000000000000083, 0.04666666666666666879, 0.05000000000000000278 ),
 .UNSPECIFIED. ) 
 CURVE ( )  GEOMETRIC_REPRESENTATION_ITEM ( )  RATIONAL_B_SPLINE_CURVE ( ( 0.9755282581475768211, 0.9755282581475768211, 1.000000000000000000, 0.9510565162951535312, 1.000000000000000000, 0.9510565162951535312, 1.000000000000000000, 0.9510565162951535312, 1.000000000000000000, 0.9510565162951535312, 1.000000000000000000, 0.9755282581475768211, 0.9755282581475768211 ) ) 
 REPRESENTATION_ITEM ( '' )  );
#8837=EDGE_CURVE ( 'NONE', #4024, #1001, #8478, .T. ) ;
#8842=CARTESIAN_POINT ( 'NONE',  ( -49.86468353124999453, 37.75937500034140015, -16.20201782572375393 ) ) ;
#8846=CARTESIAN_POINT ( 'NONE',  ( -40.34137639590981905, 49.65937500034139873, -29.30972558990011478 ) ) ;
#8850=CARTESIAN_POINT ( 'NONE',  ( 15.40903463028481113, 25.32187500034139660, -47.42413220539094709 ) ) ;
#8855=CARTESIAN_POINT ( 'NONE',  ( -49.99999999999999289, 25.88125000068279746, 16.24598481164533226 ) ) ;
#8856=CARTESIAN_POINT ( 'NONE',  ( 30.90169943749475578, 48.69999999999999574, 42.53254041760200010 ) ) ;
#8858=CARTESIAN_POINT ( 'NONE',  ( -49.86468353124999453, 47.82187500034140015, -16.20201782572375393 ) ) ;
#8859=ADVANCED_FACE ( 'NONE', ( #11152 ), #15521, .F. ) ;
#8866=EDGE_LOOP ( 'NONE', ( #9951, #3324, #9619, #2142 ) ) ;
#8867=CARTESIAN_POINT ( 'NONE',  ( -5.823736356558307894E-14, 44.50000000000000000, 50.00000000000000000 ) ) ;
#8875=CARTESIAN_POINT ( 'NONE',  ( -7.919222016226870942, 40.44874571845315359, 49.99999999999997158 ) ) ;
#8880=CARTESIAN_POINT ( 'NONE',  ( 49.86468353125001585, 22.75937500034139660, 16.20201782572375038 ) ) ;
#8887=LINE ( 'NONE', #2569, #8624 ) ;
#8890=CARTESIAN_POINT ( 'NONE',  ( 8.446640517145639571E-15, 26.50000000000000000, 50.00000000000000000 ) ) ;
#8898=AXIS2_PLACEMENT_3D ( 'NONE', #8740, #10323, #16465 ) ;
#8899=CARTESIAN_POINT ( 'NONE',  ( -15.45084971874736368, 20.40000000000000213, 47.55282581475768211 ) ) ;
#8902=CARTESIAN_POINT ( 'NONE',  ( 49.86468353125000164, 40.85937500034139447, -6.106662507704105588E-15 ) ) ;
#8906=CARTESIAN_POINT ( 'NONE',  ( -15.40903463028480580, 26.25937500034140015, 47.42413220539094709 ) ) ;
#8909=CARTESIAN_POINT ( 'NONE',  ( 7.919222016226822092, 26.55125428154684641, 49.99999999999999289 ) ) ;
#8911=CARTESIAN_POINT ( 'NONE',  ( 46.00435827497725683, 24.99999999999998579, -19.23833313609256734 ) ) ;
#8912=CARTESIAN_POINT ( 'NONE',  ( -49.86468353124999453, 32.02187500034139589, 16.20201782572377169 ) ) ;
#8913=CARTESIAN_POINT ( 'NONE',  ( 40.45084971874737789, 30.58125000068279675, 29.38926261462365375 ) ) ;
#8915=CARTESIAN_POINT ( 'NONE',  ( 7.919222016226854954, 42.55125428154684641, 49.99999999999998579 ) ) ;
#8917=CARTESIAN_POINT ( 'NONE',  ( -7.919222016226934890, 30.22999571913595318, 49.99999999999996447 ) ) ;
#8920=AXIS2_PLACEMENT_3D ( 'NONE', #6884, #5631, #291 ) ;
#8921=CARTESIAN_POINT ( 'NONE',  ( 49.86468353125000164, 32.92187500034139447, -6.106662507704105588E-15 ) ) ;
#8929=CARTESIAN_POINT ( 'NONE',  ( -40.34137639590981195, 36.05937500034139731, 29.30972558990012189 ) ) ;
#8934=CARTESIAN_POINT ( 'NONE',  ( -15.40903463028481646, 47.45937500034139589, -47.42413220539093999 ) ) ;
#8939=CARTESIAN_POINT ( 'NONE',  ( 40.34137639590981195, 21.12187500034139376, -29.30972558990011834 ) ) ;
#8944=CARTESIAN_POINT ( 'NONE',  ( -3.219174618344376363E-15, 49.50000000000000711, -52.57311121191334990 ) ) ;
#8948=CARTESIAN_POINT ( 'NONE',  ( 30.81806926056964002, 48.62187500034139731, 42.41743335407647209 ) ) ;
#8950=CIRCLE ( 'NONE', #7093, 42.00000000000000711 ) ;
#8965=CARTESIAN_POINT ( 'NONE',  ( -40.45084971874737079, 35.98125000068279888, 29.38926261462367151 ) ) ;
#8969=CARTESIAN_POINT ( 'NONE',  ( 15.40903463028482356, 48.52187500034140299, 47.42413220539093999 ) ) ;
#8973=ORIENTED_EDGE ( 'NONE', *, *, #3067, .F. ) ;
#8975=DIRECTION ( 'NONE',  ( -0.000000000000000000, -1.000000000000000000, -0.000000000000000000 ) ) ;
#8986=CARTESIAN_POINT ( 'NONE',  ( 15.45084971874737789, 22.60000000000000142, 47.55282581475767500 ) ) ;
#8991=CARTESIAN_POINT ( 'NONE',  ( -15.40903463028480580, 44.25937500034140015, 47.42413220539094709 ) ) ;
#8992=ORIENTED_EDGE ( 'NONE', *, *, #8453, .T. ) ;
#8996=CARTESIAN_POINT ( 'NONE',  ( 49.86468353124999453, 28.95937500034139944, -16.20201782572376459 ) ) ;
#9000=CARTESIAN_POINT ( 'NONE',  ( 48.20095974065459643, 25.00000000000000000, -12.77318064350110838 ) ) ;
#9001=CARTESIAN_POINT ( 'NONE',  ( -15.40903463028480580, 32.32187500034139305, 47.42413220539094709 ) ) ;
#9004=CARTESIAN_POINT ( 'NONE',  ( 7.513064459987437071E-14, 42.50000000000000000, 50.00000000000000000 ) ) ;
#9009=EDGE_CURVE ( 'NONE', #9775, #11764, #11229, .T. ) ;
#9011=CARTESIAN_POINT ( 'NONE',  ( 49.86468353125001585, 32.82187500034139305, 16.20201782572375038 ) ) ;
#9014=EDGE_CURVE ( 'NONE', #4580, #3492, #16456, .T. ) ;
#9015=CARTESIAN_POINT ( 'NONE',  ( 15.40903463028482356, 38.45937500034139589, 47.42413220539093999 ) ) ;
#9019=CARTESIAN_POINT ( 'NONE',  ( 15.40903463028482356, 46.45937500034139589, 47.42413220539093999 ) ) ;
#9022=CARTESIAN_POINT ( 'NONE',  ( 40.34137639590981195, 27.12187500034139731, -29.30972558990011834 ) ) ;
#9027=CARTESIAN_POINT ( 'NONE',  ( -30.90169943749473802, 48.30000000000000426, 42.53254041760200721 ) ) ;
#9030=CIRCLE ( 'NONE', #1846, 47.00000000000000000 ) ;
#9032=CYLINDRICAL_SURFACE ( 'NONE', #896, 82.49773270518484480 ) ;
#9034=CARTESIAN_POINT ( 'NONE',  ( -40.45084971874737789, 39.58125000068280031, -29.38926261462365730 ) ) ;
#9036=CARTESIAN_POINT ( 'NONE',  ( 2.600676159226420495E-13, 31.49999999999999289, -49.99999999999999289 ) ) ;
#9038=( BOUNDED_CURVE ( )  B_SPLINE_CURVE ( 2, ( #2368, #6046, #865, #11022, #16092, #9786, #4725, #14831, #3460, #11118, #14996, #10277, #13913 ),
 .UNSPECIFIED., .F., .F. ) 
 B_SPLINE_CURVE_WITH_KNOTS ( ( 3, 2, 2, 2, 2, 2, 3 ),
 ( 0.2833333333333333814, 0.2866666666666666807, 0.2933333333333333348, 0.2999999999999999889, 0.3066666666666666430, 0.3133333333333333526, 0.3166666666666667074 ),
 .UNSPECIFIED. ) 
 CURVE ( )  GEOMETRIC_REPRESENTATION_ITEM ( )  RATIONAL_B_SPLINE_CURVE ( ( 0.9755282581475768211, 0.9755282581475770431, 1.000000000000000000, 0.9510565162951535312, 1.000000000000000000, 0.9510565162951535312, 1.000000000000000000, 0.9510565162951535312, 1.000000000000000000, 0.9510565162951535312, 1.000000000000000000, 0.9755282581475765991, 0.9755282581475768211 ) ) 
 REPRESENTATION_ITEM ( '' )  );
#9040=CARTESIAN_POINT ( 'NONE',  ( 30.81806926056962936, 49.22187500034139873, -42.41743335407646498 ) ) ;
#9046=CARTESIAN_POINT ( 'NONE',  ( -1.240322475938754499E-13, 36.28125000068280315, 50.00000000000000000 ) ) ;
#9049=EDGE_CURVE ( 'NONE', #3473, #8435, #5009, .T. ) ;
#9050=CARTESIAN_POINT ( 'NONE',  ( 30.81806926056964002, 46.62187500034140442, 42.41743335407647209 ) ) ;
#9058=EDGE_CURVE ( 'NONE', #7884, #11917, #10309, .T. ) ;
#9059=CARTESIAN_POINT ( 'NONE',  ( 15.45084971874737789, 28.60000000000000142, 47.55282581475767500 ) ) ;
#9062=DIRECTION ( 'NONE',  ( 0.000000000000000000, 0.000000000000000000, 1.000000000000000000 ) ) ;
#9063=CARTESIAN_POINT ( 'NONE',  ( 15.45084971874737789, 48.38125000068280457, 47.55282581475767500 ) ) ;
#9073=CARTESIAN_POINT ( 'NONE',  ( -40.34137639590981195, 40.05937500034140442, 29.30972558990012189 ) ) ;
#9077=CARTESIAN_POINT ( 'NONE',  ( -49.86468353124999453, 29.95937500034139944, 16.20201782572377525 ) ) ;
#9081=CARTESIAN_POINT ( 'NONE',  ( 47.98103867763196462, 25.00000000000000000, -13.57697939761754036 ) ) ;
#9082=CARTESIAN_POINT ( 'NONE',  ( 9.631387414534489405E-15, 34.42187500034139447, 52.43083105670540789 ) ) ;
#9087=DIRECTION ( 'NONE',  ( -0.000000000000000000, -1.000000000000000000, -0.000000000000000000 ) ) ;
#9090=CARTESIAN_POINT ( 'NONE',  ( 9.631387414534489405E-15, 30.42187500034139447, 52.43083105670540789 ) ) ;
#9092=UNCERTAINTY_MEASURE_WITH_UNIT (LENGTH_MEASURE( 1.000000000000000082E-05 ), #11140, 'distance_accuracy_value', 'NONE');
#9093=CARTESIAN_POINT ( 'NONE',  ( 30.81806926056962936, 39.15937500034139873, -42.41743335407646498 ) ) ;
#9097=CARTESIAN_POINT ( 'NONE',  ( 30.81806926056962936, 45.15937500034139873, -42.41743335407647209 ) ) ;
#9099=CARTESIAN_POINT ( 'NONE',  ( 30.81806926056962936, 25.22187500034139873, -42.41743335407647209 ) ) ;
#9104=CARTESIAN_POINT ( 'NONE',  ( -49.86468353124999453, 20.02187500034139589, 16.20201782572377525 ) ) ;
#9105=EDGE_CURVE ( 'NONE', #5127, #8121, #8887, .T. ) ;
#9111=CARTESIAN_POINT ( 'NONE',  ( 40.45084971874737079, 34.98125000068279888, -29.38926261462366440 ) ) ;
#9114=CARTESIAN_POINT ( 'NONE',  ( -3.111920190527341144E-15, 25.28125000068279604, -50.00000000000000000 ) ) ;
#9117=CARTESIAN_POINT ( 'NONE',  ( -49.86468353125000164, 47.92187500034139447, 0.000000000000000000 ) ) ;
#9125=CARTESIAN_POINT ( 'NONE',  ( 40.45084971874737789, 28.58125000068280031, 29.38926261462365375 ) ) ;
#9126=ORIENTED_EDGE ( 'NONE', *, *, #10357, .T. ) ;
#9127=CARTESIAN_POINT ( 'NONE',  ( 40.34137639590981195, 47.12187500034140442, -29.30972558990011834 ) ) ;
#9128=ORIENTED_EDGE ( 'NONE', *, *, #6497, .T. ) ;
#9132=( BOUNDED_CURVE ( )  B_SPLINE_CURVE ( 2, ( #5146, #10202, #13926, #120, #2545, #8701, #13767, #5234, #16265, #3962, #2379, #11286, #9036 ),
 .UNSPECIFIED., .F., .F. ) 
 B_SPLINE_CURVE_WITH_KNOTS ( ( 3, 2, 2, 2, 2, 2, 3 ),
 ( 0.5833333333333333703, 0.5866666666666666696, 0.5933333333333333792, 0.5999999999999999778, 0.6066666666666666874, 0.6133333333333332860, 0.6166666666666666963 ),
 .UNSPECIFIED. ) 
 CURVE ( )  GEOMETRIC_REPRESENTATION_ITEM ( )  RATIONAL_B_SPLINE_CURVE ( ( 0.9755282581475768211, 0.9755282581475771542, 1.000000000000000000, 0.9510565162951535312, 1.000000000000000000, 0.9510565162951535312, 1.000000000000000000, 0.9510565162951535312, 1.000000000000000000, 0.9510565162951535312, 1.000000000000000000, 0.9755282581475763770, 0.9755282581475768211 ) ) 
 REPRESENTATION_ITEM ( '' )  );
#9145=CARTESIAN_POINT ( 'NONE',  ( -30.90169943749474513, 37.48125000068279888, -42.53254041760200721 ) ) ;
#9149=PRODUCT_DEFINITION ( 'UNKNOWN', '', #947, #2767 ) ;
#9152=CARTESIAN_POINT ( 'NONE',  ( -40.34137639590981195, 36.05937500034139731, 29.30972558990012189 ) ) ;
#9154=DIRECTION ( 'NONE',  ( 0.000000000000000000, -0.000000000000000000, 1.000000000000000000 ) ) ;
#9156=CARTESIAN_POINT ( 'NONE',  ( -30.81806926056962226, 24.15937500034139873, 42.41743335407647919 ) ) ;
#9160=CARTESIAN_POINT ( 'NONE',  ( 7.735767786613922123E-15, 54.00000000000000711, -63.16733765196516970 ) ) ;
#9161=CARTESIAN_POINT ( 'NONE',  ( 30.81806926056964002, 28.62187500034139731, 42.41743335407646498 ) ) ;
#9162=VECTOR ( 'NONE', #9571, 1000.000000000000000 ) ;
#9171=CARTESIAN_POINT ( 'NONE',  ( -30.81806926056962226, 28.22187500034139873, 42.41743335407647919 ) ) ;
#9176=CARTESIAN_POINT ( 'NONE',  ( 15.40903463028482356, 30.45937500034139589, 47.42413220539093999 ) ) ;
#9180=CARTESIAN_POINT ( 'NONE',  ( 15.40903463028481113, 49.25937500034139305, -47.42413220539094709 ) ) ;
#9186=AXIS2_PLACEMENT_3D ( 'NONE', #11358, #1189, #5135 ) ;
#9189=CARTESIAN_POINT ( 'NONE',  ( 30.90169943749475578, 40.69999999999999574, 42.53254041760200010 ) ) ;
#9196=EDGE_CURVE ( 'NONE', #13613, #15272, #6822, .T. ) ;
#9202=CARTESIAN_POINT ( 'NONE',  ( -49.99999999999999289, 35.68125000068278752, -16.24598481164531449 ) ) ;
#9207=CARTESIAN_POINT ( 'NONE',  ( 49.86468353125001585, 46.82187500034139305, 16.20201782572375038 ) ) ;
#9210=CYLINDRICAL_SURFACE ( 'NONE', #12640, 50.00000000000000000 ) ;
#9215=DIRECTION ( 'NONE',  ( -0.000000000000000000, -1.000000000000000000, -0.000000000000000000 ) ) ;
#9219=CARTESIAN_POINT ( 'NONE',  ( -40.34137639590981905, 45.72187500034139873, -29.30972558990011478 ) ) ;
#9233=CARTESIAN_POINT ( 'NONE',  ( -7.919222016226816763, 45.55125428154684641, -49.99999999999999289 ) ) ;
#9237=CARTESIAN_POINT ( 'NONE',  ( 1.293669679204937499E-13, 39.50000000000000711, -50.00000000000000000 ) ) ;
#9240=ORIENTED_EDGE ( 'NONE', *, *, #2139, .F. ) ;
#9242=CARTESIAN_POINT ( 'NONE',  ( -30.81806926056962226, 38.15937500034138452, 42.41743335407647919 ) ) ;
#9249=CARTESIAN_POINT ( 'NONE',  ( -7.919222016226802552, 47.55125428154684641, -50.00000000000000000 ) ) ;
#9250=CARTESIAN_POINT ( 'NONE',  ( 30.90169943749475223, 34.70000000000000284, 42.53254041760199300 ) ) ;
#9252=CARTESIAN_POINT ( 'NONE',  ( 49.86468353125001585, 28.82187500034139305, 16.20201782572375038 ) ) ;
#9258=CARTESIAN_POINT ( 'NONE',  ( 15.45084971874736723, 37.40000000000000568, -47.55282581475768211 ) ) ;
#9263=CARTESIAN_POINT ( 'NONE',  ( 30.81806926056964002, 30.55937500034139731, 42.41743335407646498 ) ) ;
#9266=CARTESIAN_POINT ( 'NONE',  ( -3.210462471511496205E-15, 43.35937500034138736, -52.43083105670540789 ) ) ;
#9268=CARTESIAN_POINT ( 'NONE',  ( 0.000000000000000000, 25.00000000000000000, 0.000000000000000000 ) ) ;
#9269=EDGE_CURVE ( 'NONE', #1639, #3492, #3600, .T. ) ;
#9276=CARTESIAN_POINT ( 'NONE',  ( 49.99999999999999289, 39.10000000000000853, -16.24598481164532160 ) ) ;
#9279=CARTESIAN_POINT ( 'NONE',  ( 30.81806926056962936, 43.22187500034140584, -42.41743335407647209 ) ) ;
#9282=CARTESIAN_POINT ( 'NONE',  ( 40.34137639590981195, 47.05937500034140442, -29.30972558990011834 ) ) ;
#9283=ORIENTED_EDGE ( 'NONE', *, *, #7135, .F. ) ;
#9284=CARTESIAN_POINT ( 'NONE',  ( 49.99999999999999289, 28.88125000068279391, -16.24598481164532160 ) ) ;
#9285=ORIENTED_EDGE ( 'NONE', *, *, #7538, .T. ) ;
#9289=CARTESIAN_POINT ( 'NONE',  ( 40.34137639590981195, 45.12187500034139731, -29.30972558990011834 ) ) ;
#9296=CARTESIAN_POINT ( 'NONE',  ( 15.45084971874736723, 35.18125000068280173, -47.55282581475768211 ) ) ;
#9299=CARTESIAN_POINT ( 'NONE',  ( 7.919222016226822092, 28.33250428222963890, 49.99999999999999289 ) ) ;
#9301=CARTESIAN_POINT ( 'NONE',  ( 49.86468353124999453, 49.02187500034140299, -16.20201782572376459 ) ) ;
#9304=ORIENTED_EDGE ( 'NONE', *, *, #9058, .F. ) ;
#9313=FACE_OUTER_BOUND ( 'NONE', #5967, .T. ) ;
#9319=CYLINDRICAL_SURFACE ( 'NONE', #1655, 79.49773270518484480 ) ;
#9321=CARTESIAN_POINT ( 'NONE',  ( -49.86468353125000164, 37.85937500034139447, 0.000000000000000000 ) ) ;
#9324=FACE_OUTER_BOUND ( 'NONE', #3982, .T. ) ;
#9326=CARTESIAN_POINT ( 'NONE',  ( -49.86468353125000164, 23.85937500034139447, 0.000000000000000000 ) ) ;
#9330=DIRECTION ( 'NONE',  ( 1.000000000000000000, -0.000000000000000000, 1.224646799147353207E-16 ) ) ;
#9331=CARTESIAN_POINT ( 'NONE',  ( 49.86468353124999453, 27.02187500034139944, -16.20201782572376104 ) ) ;
#9336=( BOUNDED_CURVE ( )  B_SPLINE_CURVE ( 2, ( #397, #5506, #15536, #4250, #7898, #10398, #14290, #6834, #5584, #9145, #15455, #2911, #319 ),
 .UNSPECIFIED., .F., .F. ) 
 B_SPLINE_CURVE_WITH_KNOTS ( ( 3, 2, 2, 2, 2, 2, 3 ),
 ( 0.3833333333333333592, 0.3866666666666666585, 0.3933333333333333126, 0.4000000000000000222, 0.4066666666666666763, 0.4133333333333333304, 0.4166666666666666852 ),
 .UNSPECIFIED. ) 
 CURVE ( )  GEOMETRIC_REPRESENTATION_ITEM ( )  RATIONAL_B_SPLINE_CURVE ( ( 0.9755282581475768211, 0.9755282581475770431, 1.000000000000000000, 0.9510565162951535312, 1.000000000000000000, 0.9510565162951535312, 1.000000000000000000, 0.9510565162951535312, 1.000000000000000000, 0.9510565162951535312, 1.000000000000000000, 0.9755282581475765991, 0.9755282581475768211 ) ) 
 REPRESENTATION_ITEM ( '' )  );
#9338=CARTESIAN_POINT ( 'NONE',  ( -49.99999999999999289, 34.10000000000000853, 16.24598481164533226 ) ) ;
#9342=CARTESIAN_POINT ( 'NONE',  ( 49.86468353125001585, 30.75937500034139305, 16.20201782572375038 ) ) ;
#9343=ORIENTED_EDGE ( 'NONE', *, *, #9912, .F. ) ;
#9345=CARTESIAN_POINT ( 'NONE',  ( 40.34137639590981905, 42.65937500034139873, 29.30972558990010768 ) ) ;
#9352=CARTESIAN_POINT ( 'NONE',  ( -40.45084971874737789, 39.80000000000000426, -29.38926261462365730 ) ) ;
#9354=CARTESIAN_POINT ( 'NONE',  ( -49.86468353124999453, 44.02187500034139589, 16.20201782572377525 ) ) ;
#9358=CARTESIAN_POINT ( 'NONE',  ( -2.547328955960238000E-13, 30.49999999999999645, 49.99999999999999289 ) ) ;
#9360=CARTESIAN_POINT ( 'NONE',  ( -49.99999999999999289, 29.68125000068279817, -16.24598481164531449 ) ) ;
#9367=CARTESIAN_POINT ( 'NONE',  ( -30.81806926056963292, 47.62187500034139731, -42.41743335407646498 ) ) ;
#9377=CARTESIAN_POINT ( 'NONE',  ( 30.81806926056964002, 40.62187500034139731, 42.41743335407647209 ) ) ;
#9397=VERTEX_POINT ( 'NONE', #10875 ) ;
#9398=CARTESIAN_POINT ( 'NONE',  ( 40.34137639590981905, 40.65937500034139873, 29.30972558990010768 ) ) ;
#9402=DIRECTION ( 'NONE',  ( 0.000000000000000000, 1.000000000000000000, 0.000000000000000000 ) ) ;
#9404=CARTESIAN_POINT ( 'NONE',  ( 49.86468353125001585, 24.75937500034140015, 16.20201782572375038 ) ) ;
#9405=ORIENTED_EDGE ( 'NONE', *, *, #16062, .T. ) ;
#9409=CARTESIAN_POINT ( 'NONE',  ( 15.40903463028481113, 25.32187500034139660, -47.42413220539094709 ) ) ;
#9410=CARTESIAN_POINT ( 'NONE',  ( -3.111920190527341144E-15, 29.28125000068279604, -50.00000000000000000 ) ) ;
#9416=CARTESIAN_POINT ( 'NONE',  ( 50.00000000000000000, 37.00000000000000711, -6.123233995736766085E-15 ) ) ;
#9420=CARTESIAN_POINT ( 'NONE',  ( -15.40903463028480580, 32.25937500034140015, 47.42413220539094709 ) ) ;
#9421=ORIENTED_EDGE ( 'NONE', *, *, #8226, .T. ) ;
#9423=CARTESIAN_POINT ( 'NONE',  ( 15.40903463028482356, 40.45937500034139589, 47.42413220539093999 ) ) ;
#9431=CARTESIAN_POINT ( 'NONE',  ( 30.81806926056964002, 32.62187500034140442, 42.41743335407647209 ) ) ;
#9432=CARTESIAN_POINT ( 'NONE',  ( -50.00000000000000000, 44.00000000000000711, 0.000000000000000000 ) ) ;
#9434=CARTESIAN_POINT ( 'NONE',  ( 49.86468353124999453, 45.02187500034138878, -16.20201782572376459 ) ) ;
#9439=CARTESIAN_POINT ( 'NONE',  ( 40.34137639590981195, 49.05937500034139731, -29.30972558990011834 ) ) ;
#9441=CARTESIAN_POINT ( 'NONE',  ( 15.45084971874737789, 30.38125000068280102, 47.55282581475767500 ) ) ;
#9445=CARTESIAN_POINT ( 'NONE',  ( 49.86468353125001585, 38.82187500034140015, 16.20201782572375038 ) ) ;
#9449=CARTESIAN_POINT ( 'NONE',  ( -49.99999999999999289, 39.88125000068280457, 16.24598481164533226 ) ) ;
#9453=CARTESIAN_POINT ( 'NONE',  ( -50.00000000000000000, 45.78125000068279604, 0.000000000000000000 ) ) ;
#9458=CARTESIAN_POINT ( 'NONE',  ( 40.34137639590981905, 40.72187500034139873, 29.30972558990010768 ) ) ;
#9460=EDGE_LOOP ( 'NONE', ( #10872, #11270, #1162, #12342 ) ) ;
#9465=DIRECTION ( 'NONE',  ( 0.000000000000000000, 0.000000000000000000, 1.000000000000000000 ) ) ;
#9474=CARTESIAN_POINT ( 'NONE',  ( -7.919222016226822092, 46.44874571845315359, 50.00000000000000000 ) ) ;
#9483=CARTESIAN_POINT ( 'NONE',  ( -49.86468353124999453, 29.95937500034139944, 16.20201782572377525 ) ) ;
#9490=CARTESIAN_POINT ( 'NONE',  ( -40.45084971874737079, 47.98125000068279888, 29.38926261462367151 ) ) ;
#9497=CARTESIAN_POINT ( 'NONE',  ( -40.34137639590981905, 27.72187500034139873, -29.30972558990011478 ) ) ;
#9498=CARTESIAN_POINT ( 'NONE',  ( 40.45084971874737789, 38.80000000000000426, 29.38926261462365375 ) ) ;
#9505=CARTESIAN_POINT ( 'NONE',  ( 15.45084971874736723, 33.39999999999999858, -47.55282581475768211 ) ) ;
#9507=CARTESIAN_POINT ( 'NONE',  ( -49.86468353124999453, 49.75937500034138594, -16.20201782572375393 ) ) ;
#9508=VERTEX_POINT ( 'NONE', #2128 ) ;
#9509=CARTESIAN_POINT ( 'NONE',  ( -30.81806926056962226, 32.15937500034139873, 42.41743335407647209 ) ) ;
#9512=CARTESIAN_POINT ( 'NONE',  ( 49.86468353124999453, 38.95937500034139589, -16.20201782572376459 ) ) ;
#9520=CARTESIAN_POINT ( 'NONE',  ( -30.81806926056962226, 32.22187500034139163, 42.41743335407647919 ) ) ;
#9521=CARTESIAN_POINT ( 'NONE',  ( 9.657523855033129090E-15, 42.50000000000000711, 52.57311121191334990 ) ) ;
#9523=CARTESIAN_POINT ( 'NONE',  ( -49.86468353124999453, 42.02187500034139589, 16.20201782572377525 ) ) ;
#9524=ADVANCED_FACE ( 'NONE', ( #5973 ), #8608, .T. ) ;
#9527=CARTESIAN_POINT ( 'NONE',  ( -15.40903463028481646, 49.45937500034140299, -47.42413220539093999 ) ) ;
#9530=CARTESIAN_POINT ( 'NONE',  ( 30.90169943749474157, 31.08125000068280031, -42.53254041760200721 ) ) ;
#9532=ORIENTED_EDGE ( 'NONE', *, *, #534, .F. ) ;
#9534=CARTESIAN_POINT ( 'NONE',  ( 30.90169943749473802, 33.08125000068279320, -42.53254041760200721 ) ) ;
#9535=CARTESIAN_POINT ( 'NONE',  ( 15.40903463028482356, 42.52187500034139589, 47.42413220539093999 ) ) ;
#9543=CARTESIAN_POINT ( 'NONE',  ( -15.40903463028481646, 43.52187500034139589, -47.42413220539093999 ) ) ;
#9549=CARTESIAN_POINT ( 'NONE',  ( 0.000000000000000000, 52.00000000000000711, 0.000000000000000000 ) ) ;
#9554=CARTESIAN_POINT ( 'NONE',  ( -30.90169943749474513, 29.69999999999999929, -42.53254041760200721 ) ) ;
#9555=CARTESIAN_POINT ( 'NONE',  ( -15.45084971874737256, 33.38125000068280457, -47.55282581475767500 ) ) ;
#9560=CARTESIAN_POINT ( 'NONE',  ( -15.45084971874736368, 34.39999999999999858, 47.55282581475768211 ) ) ;
#9563=CARTESIAN_POINT ( 'NONE',  ( 9.631387414534489405E-15, 30.35937500034139447, 52.43083105670540789 ) ) ;
#9569=CARTESIAN_POINT ( 'NONE',  ( -3.219174618344376363E-15, 43.28125000068280315, -52.57311121191334990 ) ) ;
#9571=DIRECTION ( 'NONE',  ( -0.000000000000000000, -1.000000000000000000, -0.000000000000000000 ) ) ;
#9578=CARTESIAN_POINT ( 'NONE',  ( 6.123233995736766085E-15, 193.4213562373095385, 50.00000000000000000 ) ) ;
#9584=CARTESIAN_POINT ( 'NONE',  ( 49.99999999999999289, 33.10000000000000853, -16.24598481164532160 ) ) ;
#9588=LINE ( 'NONE', #15901, #14192 ) ;
#9591=CARTESIAN_POINT ( 'NONE',  ( -40.34137639590981195, 44.05937500034139731, 29.30972558990012189 ) ) ;
#9596=FACE_OUTER_BOUND ( 'NONE', #8762, .T. ) ;
#9597=CARTESIAN_POINT ( 'NONE',  ( -15.40903463028481646, 33.52187500034140299, -47.42413220539093999 ) ) ;
#9600=CARTESIAN_POINT ( 'NONE',  ( 40.34137639590981195, 39.12187500034139731, -29.30972558990011834 ) ) ;
#9603=CARTESIAN_POINT ( 'NONE',  ( 49.86468353125000164, 48.85937500034139447, -6.106662507704105588E-15 ) ) ;
#9606=CARTESIAN_POINT ( 'NONE',  ( -50.00000000000000000, 33.78125000068280315, 0.000000000000000000 ) ) ;
#9609=CARTESIAN_POINT ( 'NONE',  ( -49.86468353125000164, 39.92187500034139447, 0.000000000000000000 ) ) ;
#9612=DIRECTION ( 'NONE',  ( 0.000000000000000000, 0.000000000000000000, 1.000000000000000000 ) ) ;
#9613=CARTESIAN_POINT ( 'NONE',  ( -30.81806926056963292, 25.62187500034139731, -42.41743335407647209 ) ) ;
#9618=CARTESIAN_POINT ( 'NONE',  ( -40.34137639590981905, 39.72187500034139873, -29.30972558990011478 ) ) ;
#9619=ORIENTED_EDGE ( 'NONE', *, *, #15346, .T. ) ;
#9636=CARTESIAN_POINT ( 'NONE',  ( -3.210462471511496205E-15, 33.35937500034140157, -52.43083105670540789 ) ) ;
#9641=CARTESIAN_POINT ( 'NONE',  ( -15.45084971874736368, 42.18125000068279462, 47.55282581475768211 ) ) ;
#9649=CYLINDRICAL_SURFACE ( 'NONE', #4082, 47.00000000000000000 ) ;
#9651=CARTESIAN_POINT ( 'NONE',  ( 15.45084971874737789, 38.60000000000000142, 47.55282581475767500 ) ) ;
#9652=CARTESIAN_POINT ( 'NONE',  ( 30.90169943749473802, 37.08125000068280031, -42.53254041760200721 ) ) ;
#9654=DIRECTION ( 'NONE',  ( -0.000000000000000000, -1.000000000000000000, -0.000000000000000000 ) ) ;
#9657=CARTESIAN_POINT ( 'NONE',  ( 40.45084971874737079, 31.20000000000000284, -29.38926261462366440 ) ) ;
#9661=EDGE_LOOP ( 'NONE', ( #2294, #1472, #6995, #4501 ) ) ;
#9662=CARTESIAN_POINT ( 'NONE',  ( 9.631387414534489405E-15, 26.35937500034139802, 52.43083105670540789 ) ) ;
#9665=CARTESIAN_POINT ( 'NONE',  ( -30.81806926056962226, 38.15937500034138452, 42.41743335407647919 ) ) ;
#9667=EDGE_CURVE ( 'NONE', #11385, #5080, #16018, .T. ) ;
#9675=CARTESIAN_POINT ( 'NONE',  ( 15.40903463028482356, 28.52187500034139589, 47.42413220539093999 ) ) ;
#9679=CARTESIAN_POINT ( 'NONE',  ( 49.86468353125001585, 34.82187500034140015, 16.20201782572375038 ) ) ;
#9684=CARTESIAN_POINT ( 'NONE',  ( 9.631387414534489405E-15, 40.35937500034139447, 52.43083105670540789 ) ) ;
#9685=VERTEX_POINT ( 'NONE', #7388 ) ;
#9686=CARTESIAN_POINT ( 'NONE',  ( 15.45084971874736723, 27.18125000068279817, -47.55282581475768211 ) ) ;
#9688=CARTESIAN_POINT ( 'NONE',  ( -49.99999999999999289, 36.10000000000000142, 16.24598481164533226 ) ) ;
#9689=CARTESIAN_POINT ( 'NONE',  ( 30.81806926056964002, 42.62187500034139731, 42.41743335407646498 ) ) ;
#9694=CARTESIAN_POINT ( 'NONE',  ( -49.86468353124999453, 21.82187500034139305, -16.20201782572375393 ) ) ;
#9702=CARTESIAN_POINT ( 'NONE',  ( 30.81806926056964002, 44.62187500034140442, 42.41743335407647209 ) ) ;
#9708=ORIENTED_EDGE ( 'NONE', *, *, #12429, .T. ) ;
#9718=SHAPE_REPRESENTATION_RELATIONSHIP ( 'NONE' , 'NONE' ,  #13496, #1259 ) ;
#9719=CIRCLE ( 'NONE', #12636, 82.49773270518484480 ) ;
#9724=CARTESIAN_POINT ( 'NONE',  ( -30.90169943749474513, 33.70000000000000284, -42.53254041760200721 ) ) ;
#9728=CARTESIAN_POINT ( 'NONE',  ( 30.81806926056962936, 31.15937500034139518, -42.41743335407647209 ) ) ;
#9732=CARTESIAN_POINT ( 'NONE',  ( -3.219174618344376363E-15, 45.28125000068279604, -52.57311121191334990 ) ) ;
#9741=CARTESIAN_POINT ( 'NONE',  ( -7.919222016226804328, 28.22999571913594963, 50.00000000000000000 ) ) ;
#9747=CARTESIAN_POINT ( 'NONE',  ( 15.45084971874737789, 36.38125000068279746, 47.55282581475767500 ) ) ;
#9748=CARTESIAN_POINT ( 'NONE',  ( -15.45084971874737256, 41.60000000000000142, -47.55282581475767500 ) ) ;
#9751=CARTESIAN_POINT ( 'NONE',  ( -15.45084971874736368, 30.40000000000000213, 47.55282581475768211 ) ) ;
#9760=CARTESIAN_POINT ( 'NONE',  ( 15.40903463028481113, 35.25937500034139305, -47.42413220539094709 ) ) ;
#9762=LINE ( 'NONE', #3604, #10176 ) ;
#9768=CARTESIAN_POINT ( 'NONE',  ( 15.40903463028481113, 27.32187500034139660, -47.42413220539094709 ) ) ;
#9771=CARTESIAN_POINT ( 'NONE',  ( -30.81806926056963292, 37.62187500034139020, -42.41743335407647209 ) ) ;
#9774=( BOUNDED_CURVE ( )  B_SPLINE_CURVE ( 2, ( #11335, #3521, #7427, #12013, #13567, #4376, #13645 ),
 .UNSPECIFIED., .F., .F. ) 
 B_SPLINE_CURVE_WITH_KNOTS ( ( 3, 2, 2, 3 ),
 ( 0.000000000000000000, 0.006666666666666667095, 0.01333333333333333419, 0.01666666666666666644 ),
 .UNSPECIFIED. ) 
 CURVE ( )  GEOMETRIC_REPRESENTATION_ITEM ( )  RATIONAL_B_SPLINE_CURVE ( ( 1.000000000000000000, 0.9510565162951535312, 1.000000000000000000, 0.9510565162951535312, 1.000000000000000000, 0.9755282581475768211, 0.9755282581475768211 ) ) 
 REPRESENTATION_ITEM ( '' )  );
#9775=VERTEX_POINT ( 'NONE', #8025 ) ;
#9776=CARTESIAN_POINT ( 'NONE',  ( -15.40903463028481646, 43.45937500034139589, -47.42413220539093999 ) ) ;
#9778=CARTESIAN_POINT ( 'NONE',  ( 50.00000000000000000, 26.78125000068279959, -6.123233995736766085E-15 ) ) ;
#9783=CARTESIAN_POINT ( 'NONE',  ( -3.111920190527341144E-15, 35.50000000000000000, -50.00000000000000000 ) ) ;
#9784=CARTESIAN_POINT ( 'NONE',  ( 15.40903463028482356, 38.52187500034139589, 47.42413220539093999 ) ) ;
#9786=CARTESIAN_POINT ( 'NONE',  ( 49.99999999999999289, 41.10000000000000142, -16.24598481164532160 ) ) ;
#9787=CARTESIAN_POINT ( 'NONE',  ( 15.40903463028482356, 22.52187500034139589, 47.42413220539093999 ) ) ;
#9792=CARTESIAN_POINT ( 'NONE',  ( -49.86468353125000164, 35.92187500034140157, 0.000000000000000000 ) ) ;
#9793=CARTESIAN_POINT ( 'NONE',  ( -30.90169943749473447, 44.08125000068279320, 42.53254041760200721 ) ) ;
#9796=ORIENTED_EDGE ( 'NONE', *, *, #9269, .T. ) ;
#9805=( LENGTH_UNIT ( ) NAMED_UNIT ( * ) SI_UNIT ( .MILLI., .METRE. ) );
#9808=CARTESIAN_POINT ( 'NONE',  ( -49.99999999999999289, 34.10000000000000853, 16.24598481164533226 ) ) ;
#9810=CARTESIAN_POINT ( 'NONE',  ( 40.34137639590981195, 33.05937500034139731, -29.30972558990011834 ) ) ;
#9814=CARTESIAN_POINT ( 'NONE',  ( 50.00000000000000000, 40.78125000068279604, -6.123233995736766085E-15 ) ) ;
#9820=CARTESIAN_POINT ( 'NONE',  ( -49.99999999999999289, 27.68125000068279462, -16.24598481164531449 ) ) ;
#9832=CARTESIAN_POINT ( 'NONE',  ( -49.99999999999999289, 30.10000000000000497, 16.24598481164533226 ) ) ;
#9840=CARTESIAN_POINT ( 'NONE',  ( -30.81806926056962226, 36.15937500034139163, 42.41743335407647919 ) ) ;
#9841=DIRECTION ( 'NONE',  ( 0.000000000000000000, 1.000000000000000000, 0.000000000000000000 ) ) ;
#9851=CARTESIAN_POINT ( 'NONE',  ( 49.86468353125001585, 40.82187500034140726, 16.20201782572375038 ) ) ;
#9854=CARTESIAN_POINT ( 'NONE',  ( 15.40903463028481113, 41.25937500034139305, -47.42413220539094709 ) ) ;
#9856=CARTESIAN_POINT ( 'NONE',  ( -49.99999999999999289, 23.68125000068279462, -16.24598481164531449 ) ) ;
#9861=CARTESIAN_POINT ( 'NONE',  ( 49.86468353125001585, 24.82187500034139305, 16.20201782572375038 ) ) ;
#9863=EDGE_CURVE ( 'NONE', #7784, #13965, #10448, .T. ) ;
#9864=( BOUNDED_CURVE ( )  B_SPLINE_CURVE ( 2, ( #16108, #966, #5974, #2129, #12278, #14676, #12453 ),
 .UNSPECIFIED., .F., .F. ) 
 B_SPLINE_CURVE_WITH_KNOTS ( ( 3, 2, 2, 3 ),
 ( 0.000000000000000000, 0.006666666666666667095, 0.01333333333333333419, 0.01666666666666666644 ),
 .UNSPECIFIED. ) 
 CURVE ( )  GEOMETRIC_REPRESENTATION_ITEM ( )  RATIONAL_B_SPLINE_CURVE ( ( 1.000000000000000000, 0.9510565162951535312, 1.000000000000000000, 0.9510565162951535312, 1.000000000000000000, 0.9755282581475768211, 0.9755282581475768211 ) ) 
 REPRESENTATION_ITEM ( '' )  );
#9868=CARTESIAN_POINT ( 'NONE',  ( -3.210462471511496205E-15, 35.42187500034140157, -52.43083105670540789 ) ) ;
#9869=CARTESIAN_POINT ( 'NONE',  ( -3.111920190527341144E-15, 43.28125000068280315, -50.00000000000000000 ) ) ;
#9881=CARTESIAN_POINT ( 'NONE',  ( 49.99999999999999289, 25.10000000000000142, -16.24598481164532160 ) ) ;
#9883=( NAMED_UNIT ( * ) PLANE_ANGLE_UNIT ( ) SI_UNIT ( $, .RADIAN. ) );
#9885=CARTESIAN_POINT ( 'NONE',  ( 50.00000000000000000, 42.78125000068280315, -6.123233995736766085E-15 ) ) ;
#9889=CARTESIAN_POINT ( 'NONE',  ( -49.86468353125000164, 21.85937500034139802, 0.000000000000000000 ) ) ;
#9892=EDGE_LOOP ( 'NONE', ( #8606, #16035, #981, #8973, #2803 ) ) ;
#9893=CARTESIAN_POINT ( 'NONE',  ( 30.90169943749475578, 44.48125000068279888, 42.53254041760200010 ) ) ;
#9894=CARTESIAN_POINT ( 'NONE',  ( 40.45084971874737789, 46.80000000000000426, 29.38926261462365375 ) ) ;
#9896=ADVANCED_FACE ( 'NONE', ( #5630 ), #10692, .T. ) ;
#9897=ORIENTED_EDGE ( 'NONE', *, *, #14923, .F. ) ;
#9902=CARTESIAN_POINT ( 'NONE',  ( 48.35726954556789536, 24.99999999999999645, -12.16803787670825265 ) ) ;
#9903=CARTESIAN_POINT ( 'NONE',  ( 41.19975849074683794, 25.00000000000000711, -28.55207485309309945 ) ) ;
#9910=CARTESIAN_POINT ( 'NONE',  ( 40.45084971874737079, 27.20000000000000284, -29.38926261462366440 ) ) ;
#9912=EDGE_CURVE ( 'NONE', #5251, #2810, #12856, .T. ) ;
#9913=CARTESIAN_POINT ( 'NONE',  ( -30.90169943749474513, 43.70000000000000284, -42.53254041760200721 ) ) ;
#9914=CARTESIAN_POINT ( 'NONE',  ( 30.81806926056964002, 44.55937500034139020, 42.41743335407647209 ) ) ;
#9920=CARTESIAN_POINT ( 'NONE',  ( -49.86468353124999453, 37.75937500034140015, -16.20201782572375393 ) ) ;
#9921=CARTESIAN_POINT ( 'NONE',  ( 40.45084971874737079, 40.98125000068279888, -29.38926261462366440 ) ) ;
#9932=CARTESIAN_POINT ( 'NONE',  ( 9.631387414534489405E-15, 38.42187500034139447, 52.43083105670540789 ) ) ;
#9935=CARTESIAN_POINT ( 'NONE',  ( 40.34137639590981905, 42.65937500034139873, 29.30972558990010768 ) ) ;
#9938=CARTESIAN_POINT ( 'NONE',  ( -3.219174618344376363E-15, 21.28125000068279959, -52.57311121191334990 ) ) ;
#9940=CARTESIAN_POINT ( 'NONE',  ( -40.45084971874737079, 36.20000000000000284, 29.38926261462367151 ) ) ;
#9943=CARTESIAN_POINT ( 'NONE',  ( 49.86468353124999453, 21.02187500034139589, -16.20201782572376459 ) ) ;
#9948=CARTESIAN_POINT ( 'NONE',  ( 30.81806926056962936, 35.22187500034138452, -42.41743335407647209 ) ) ;
#9949=CARTESIAN_POINT ( 'NONE',  ( -30.90169943749473447, 42.08125000068279320, 42.53254041760200721 ) ) ;
#9951=ORIENTED_EDGE ( 'NONE', *, *, #8837, .F. ) ;
#9961=( BOUNDED_CURVE ( )  B_SPLINE_CURVE ( 2, ( #7114, #14816, #12170, #12426, #5946, #771, #11008, #4706, #3447, #12331, #932, #15146, #14064 ),
 .UNSPECIFIED., .F., .F. ) 
 B_SPLINE_CURVE_WITH_KNOTS ( ( 3, 2, 2, 2, 2, 2, 3 ),
 ( 0.5500000000000000444, 0.5533333333333333437, 0.5600000000000000533, 0.5666666666666666519, 0.5733333333333333615, 0.5799999999999999600, 0.5833333333333333703 ),
 .UNSPECIFIED. ) 
 CURVE ( )  GEOMETRIC_REPRESENTATION_ITEM ( )  RATIONAL_B_SPLINE_CURVE ( ( 0.9755282581475768211, 0.9755282581475771542, 1.000000000000000000, 0.9510565162951535312, 1.000000000000000000, 0.9510565162951535312, 1.000000000000000000, 0.9510565162951535312, 1.000000000000000000, 0.9510565162951535312, 1.000000000000000000, 0.9755282581475763770, 0.9755282581475768211 ) ) 
 REPRESENTATION_ITEM ( '' )  );
#9964=FACE_OUTER_BOUND ( 'NONE', #3048, .T. ) ;
#9965=CARTESIAN_POINT ( 'NONE',  ( 29.32979127811506004, 25.09142360399907901, -43.04328433925368813 ) ) ;
#9969=CARTESIAN_POINT ( 'NONE',  ( 49.86468353125000164, 26.85937500034139802, -6.106662507704105588E-15 ) ) ;
#9971=ORIENTED_EDGE ( 'NONE', *, *, #14934, .F. ) ;
#9975=CARTESIAN_POINT ( 'NONE',  ( 40.45084971874737079, 38.98125000068279888, -29.38926261462366440 ) ) ;
#9976=CARTESIAN_POINT ( 'NONE',  ( 6.123233995736766085E-15, 193.4213562373095385, 50.00000000000000000 ) ) ;
#9979=CARTESIAN_POINT ( 'NONE',  ( 15.45084971874736723, 39.18125000068280173, -47.55282581475768211 ) ) ;
#9987=FACE_OUTER_BOUND ( 'NONE', #6973, .T. ) ;
#9991=CARTESIAN_POINT ( 'NONE',  ( -49.99999999999999289, 26.10000000000000142, 16.24598481164533226 ) ) ;
#9994=CARTESIAN_POINT ( 'NONE',  ( 9.631387414534489405E-15, 44.35937500034140157, 52.43083105670540789 ) ) ;
#9999=AXIS2_PLACEMENT_3D ( 'NONE', #15369, #14038, #9062 ) ;
#10003=CARTESIAN_POINT ( 'NONE',  ( -49.86468353125000164, 33.85937500034139447, 0.000000000000000000 ) ) ;
#10004=CARTESIAN_POINT ( 'NONE',  ( 0.000000000000000000, 193.4213562373095385, 0.000000000000000000 ) ) ;
#10007=CARTESIAN_POINT ( 'NONE',  ( 45.87472660798608359, 24.99999999999998579, -19.54543171153504488 ) ) ;
#10013=CARTESIAN_POINT ( 'NONE',  ( 15.45084971874737789, 42.60000000000000142, 47.55282581475767500 ) ) ;
#10016=CARTESIAN_POINT ( 'NONE',  ( -50.00000000000000000, 29.78125000068279959, 0.000000000000000000 ) ) ;
#10019=CARTESIAN_POINT ( 'NONE',  ( 40.34137639590981195, 29.12187500034139376, -29.30972558990011834 ) ) ;
#10020=( BOUNDED_CURVE ( )  B_SPLINE_CURVE ( 2, ( #11161, #5758, #5838, #9652, #13385, #4675, #7332, #8320, #993, #3586, #9747, #12149, #2330 ),
 .UNSPECIFIED., .F., .F. ) 
 B_SPLINE_CURVE_WITH_KNOTS ( ( 3, 2, 2, 2, 2, 2, 3 ),
 ( 0.4166666666666666852, 0.4199999999999999845, 0.4266666666666666941, 0.4333333333333333481, 0.4400000000000000022, 0.4466666666666666563, 0.4500000000000000111 ),
 .UNSPECIFIED. ) 
 CURVE ( )  GEOMETRIC_REPRESENTATION_ITEM ( )  RATIONAL_B_SPLINE_CURVE ( ( 0.9755282581475768211, 0.9755282581475770431, 1.000000000000000000, 0.9510565162951535312, 1.000000000000000000, 0.9510565162951535312, 1.000000000000000000, 0.9510565162951535312, 1.000000000000000000, 0.9510565162951535312, 1.000000000000000000, 0.9755282581475765991, 0.9755282581475768211 ) ) 
 REPRESENTATION_ITEM ( '' )  );
#10022=EDGE_LOOP ( 'NONE', ( #9421, #2145, #5995, #1545 ) ) ;
#10023=CARTESIAN_POINT ( 'NONE',  ( -15.40903463028480580, 40.25937500034139305, 47.42413220539094709 ) ) ;
#10026=VERTEX_POINT ( 'NONE', #15063 ) ;
#10028=CARTESIAN_POINT ( 'NONE',  ( 40.45084971874737789, 26.58125000068279675, 29.38926261462365375 ) ) ;
#10030=CARTESIAN_POINT ( 'NONE',  ( 30.81806926056964002, 22.62187500034139731, 42.41743335407647209 ) ) ;
#10034=CARTESIAN_POINT ( 'NONE',  ( 49.99999999999999289, 49.10000000000000853, -16.24598481164532160 ) ) ;
#10039=CARTESIAN_POINT ( 'NONE',  ( 15.40903463028481113, 37.32187500034140015, -47.42413220539094709 ) ) ;
#10041=ORIENTED_EDGE ( 'NONE', *, *, #13093, .T. ) ;
#10055=CARTESIAN_POINT ( 'NONE',  ( 30.81806926056962936, 27.15937500034139163, -42.41743335407647209 ) ) ;
#10074=CARTESIAN_POINT ( 'NONE',  ( 9.657523855033129090E-15, 20.50000000000000355, 52.57311121191334990 ) ) ;
#10076=CARTESIAN_POINT ( 'NONE',  ( 1.010305842943185372E-14, 272.0000000000000000, 82.49773270518484480 ) ) ;
#10078=CARTESIAN_POINT ( 'NONE',  ( 9.631387414534489405E-15, 42.35937500034140157, 52.43083105670540789 ) ) ;
#10085=CARTESIAN_POINT ( 'NONE',  ( -40.34137639590981905, 27.65937500034139873, -29.30972558990011478 ) ) ;
#10088=CARTESIAN_POINT ( 'NONE',  ( 45.47188453826132104, 25.00000000000000000, -20.46517872429543061 ) ) ;
#10089=CARTESIAN_POINT ( 'NONE',  ( -40.34137639590981195, 34.12187500034139731, 29.30972558990012189 ) ) ;
#10091=CARTESIAN_POINT ( 'NONE',  ( 8.679606986189813260E-15, 55.00000000000000711, -62.25100647794772613 ) ) ;
#10099=CARTESIAN_POINT ( 'NONE',  ( 15.40903463028482356, 28.52187500034139589, 47.42413220539093999 ) ) ;
#10101=ORIENTED_EDGE ( 'NONE', *, *, #11569, .F. ) ;
#10102=CARTESIAN_POINT ( 'NONE',  ( -15.40903463028481646, 35.45937500034139589, -47.42413220539093999 ) ) ;
#10103=ORIENTED_EDGE ( 'NONE', *, *, #5847, .F. ) ;
#10106=CARTESIAN_POINT ( 'NONE',  ( 15.45084971874737789, 20.38125000068279746, 47.55282581475767500 ) ) ;
#10108=CARTESIAN_POINT ( 'NONE',  ( 40.34137639590981195, 23.12187500034139731, -29.30972558990011834 ) ) ;
#10114=CARTESIAN_POINT ( 'NONE',  ( 50.00000000000000000, 49.00000000000000000, -6.123233995736766085E-15 ) ) ;
#10116=CARTESIAN_POINT ( 'NONE',  ( -40.34137639590981195, 48.12187500034139731, 29.30972558990012189 ) ) ;
#10124=CARTESIAN_POINT ( 'NONE',  ( 15.45084971874737789, 44.60000000000000142, 47.55282581475767500 ) ) ;
#10131=DIRECTION ( 'NONE',  ( 0.000000000000000000, 0.000000000000000000, 1.000000000000000000 ) ) ;
#10134=CARTESIAN_POINT ( 'NONE',  ( 15.40903463028482356, 24.45937500034139589, 47.42413220539093999 ) ) ;
#10135=ORIENTED_EDGE ( 'NONE', *, *, #10357, .F. ) ;
#10136=CARTESIAN_POINT ( 'NONE',  ( 0.000000000000000000, 52.00000000000000711, 0.000000000000000000 ) ) ;
#10141=CARTESIAN_POINT ( 'NONE',  ( -15.45084971874737256, 27.60000000000000142, -47.55282581475767500 ) ) ;
#10143=CARTESIAN_POINT ( 'NONE',  ( 0.000000000000000000, 51.99999999999999289, -50.00000000000000000 ) ) ;
#10151=CARTESIAN_POINT ( 'NONE',  ( -15.45084971874737256, 23.60000000000000142, -47.55282581475767500 ) ) ;
#10153=LINE ( 'NONE', #14965, #8671 ) ;
#10155=CARTESIAN_POINT ( 'NONE',  ( 40.34137639590981905, 46.65937500034139873, 29.30972558990010768 ) ) ;
#10160=CARTESIAN_POINT ( 'NONE',  ( 30.81806926056964002, 28.55937500034139731, 42.41743335407647209 ) ) ;
#10165=EDGE_CURVE ( 'NONE', #13411, #15993, #9774, .T. ) ;
#10166=CARTESIAN_POINT ( 'NONE',  ( 46.56218328577816123, 25.00000000000000000, -17.84593874833561955 ) ) ;
#10167=CARTESIAN_POINT ( 'NONE',  ( 40.34137639590981195, 37.12187500034139731, -29.30972558990011834 ) ) ;
#10168=DIRECTION ( 'NONE',  ( 0.000000000000000000, 0.000000000000000000, -1.000000000000000000 ) ) ;
#10170=DIRECTION ( 'NONE',  ( -0.000000000000000000, -1.000000000000000000, -0.000000000000000000 ) ) ;
#10175=CARTESIAN_POINT ( 'NONE',  ( -49.86468353125000164, 31.92187500034139447, 0.000000000000000000 ) ) ;
#10176=VECTOR ( 'NONE', #14810, 1000.000000000000000 ) ;
#10181=CARTESIAN_POINT ( 'NONE',  ( 49.86468353124999453, 38.95937500034139589, -16.20201782572376104 ) ) ;
#10185=CARTESIAN_POINT ( 'NONE',  ( 40.34137639590981195, 47.05937500034140442, -29.30972558990011834 ) ) ;
#10187=CARTESIAN_POINT ( 'NONE',  ( -15.40903463028481646, 25.52187500034139589, -47.42413220539093999 ) ) ;
#10193=CARTESIAN_POINT ( 'NONE',  ( 15.45084971874736723, 45.40000000000000568, -47.55282581475768211 ) ) ;
#10198=CIRCLE ( 'NONE', #8064, 79.49773270518484480 ) ;
#10202=CARTESIAN_POINT ( 'NONE',  ( -7.919222016226934890, 32.44874571845316069, 49.99999999999996447 ) ) ;
#10204=( BOUNDED_CURVE ( )  B_SPLINE_CURVE ( 2, ( #13543, #14614, #1064, #14696, #14782, #8394, #7321, #2319, #9894, #3413, #12391, #12139, #13464 ),
 .UNSPECIFIED., .F., .F. ) 
 B_SPLINE_CURVE_WITH_KNOTS ( ( 3, 2, 2, 2, 2, 2, 3 ),
 ( 0.08333333333333334259, 0.08666666666666666963, 0.09333333333333333759, 0.1000000000000000056, 0.1066666666666666735, 0.1133333333333333276, 0.1166666666666666685 ),
 .UNSPECIFIED. ) 
 CURVE ( )  GEOMETRIC_REPRESENTATION_ITEM ( )  RATIONAL_B_SPLINE_CURVE ( ( 0.9755282581475768211, 0.9755282581475768211, 1.000000000000000000, 0.9510565162951535312, 1.000000000000000000, 0.9510565162951535312, 1.000000000000000000, 0.9510565162951535312, 1.000000000000000000, 0.9510565162951535312, 1.000000000000000000, 0.9755282581475767101, 0.9755282581475768211 ) ) 
 REPRESENTATION_ITEM ( '' )  );
#10211=CARTESIAN_POINT ( 'NONE',  ( -7.919222016226752814, 39.55125428154683931, -50.00000000000000711 ) ) ;
#10212=CARTESIAN_POINT ( 'NONE',  ( -15.45084971874736368, 36.18125000068280173, 47.55282581475768211 ) ) ;
#10213=CARTESIAN_POINT ( 'NONE',  ( 15.45084971874737789, 28.38125000068279746, 47.55282581475767500 ) ) ;
#10215=CARTESIAN_POINT ( 'NONE',  ( 30.81806926056962936, 49.22187500034139873, -42.41743335407647209 ) ) ;
#10221=CARTESIAN_POINT ( 'NONE',  ( 0.000000000000000000, 193.4213562373095385, 0.000000000000000000 ) ) ;
#10234=ORIENTED_EDGE ( 'NONE', *, *, #2139, .T. ) ;
#10235=CARTESIAN_POINT ( 'NONE',  ( 49.86468353125001585, 44.75937500034138594, 16.20201782572375038 ) ) ;
#10239=CARTESIAN_POINT ( 'NONE',  ( 40.34137639590981195, 31.05937500034139731, -29.30972558990011834 ) ) ;
#10242=CARTESIAN_POINT ( 'NONE',  ( 40.45084971874737789, 26.80000000000000071, 29.38926261462365375 ) ) ;
#10245=CARTESIAN_POINT ( 'NONE',  ( 46.68017951973684632, 24.99999999999999289, -17.53418100958397829 ) ) ;
#10246=CARTESIAN_POINT ( 'NONE',  ( -15.40903463028481646, 35.52187500034139589, -47.42413220539093999 ) ) ;
#10249=CYLINDRICAL_SURFACE ( 'NONE', #7618, 50.00000000000000000 ) ;
#10256=CARTESIAN_POINT ( 'NONE',  ( 40.34137639590981195, 33.12187500034139731, -29.30972558990011834 ) ) ;
#10257=TOROIDAL_SURFACE ( 'NONE', #15821, 63.16733765196516970, 2.000000000000000000 ) ;
#10263=CARTESIAN_POINT ( 'NONE',  ( -40.34137639590981195, 34.05937500034139731, 29.30972558990012189 ) ) ;
#10267=CARTESIAN_POINT ( 'NONE',  ( 40.45084971874737079, 20.98125000068279888, -29.38926261462366440 ) ) ;
#10270=AXIS2_PLACEMENT_3D ( 'NONE', #10452, #12641, #13873 ) ;
#10272=CARTESIAN_POINT ( 'NONE',  ( 49.86468353125001585, 20.82187500034140015, 16.20201782572375038 ) ) ;
#10274=CARTESIAN_POINT ( 'NONE',  ( 8.446640517145639571E-15, 48.28125000068279604, 50.00000000000000000 ) ) ;
#10277=CARTESIAN_POINT ( 'NONE',  ( 7.919222016226758143, 40.55125428154685352, 50.00000000000000711 ) ) ;
#10279=CARTESIAN_POINT ( 'NONE',  ( 9.657523855033129090E-15, 44.50000000000000711, 52.57311121191334990 ) ) ;
#10286=CARTESIAN_POINT ( 'NONE',  ( -3.111920190527341144E-15, 35.28125000068280315, -50.00000000000000000 ) ) ;
#10288=CARTESIAN_POINT ( 'NONE',  ( 50.00000000000000000, 38.78125000068279604, -6.123233995736766085E-15 ) ) ;
#10292=CARTESIAN_POINT ( 'NONE',  ( 7.919222016226809657, 45.44874571845314648, -50.00000000000000000 ) ) ;
#10294=CARTESIAN_POINT ( 'NONE',  ( -49.86468353124999453, 46.02187500034139589, 16.20201782572377169 ) ) ;
#10300=CARTESIAN_POINT ( 'NONE',  ( 30.90169943749473802, 29.08125000068280031, -42.53254041760200721 ) ) ;
#10302=CARTESIAN_POINT ( 'NONE',  ( -30.81806926056963292, 49.62187500034139020, -42.41743335407647209 ) ) ;
#10304=CARTESIAN_POINT ( 'NONE',  ( -30.90169943749474513, 25.69999999999999574, -42.53254041760200721 ) ) ;
#10309=LINE ( 'NONE', #14111, #3331 ) ;
#10318=CARTESIAN_POINT ( 'NONE',  ( -30.90169943749473802, 20.30000000000000426, 42.53254041760200721 ) ) ;
#10321=CARTESIAN_POINT ( 'NONE',  ( 9.631387414534489405E-15, 36.35937500034140157, 52.43083105670540789 ) ) ;
#10323=DIRECTION ( 'NONE',  ( 0.000000000000000000, 1.000000000000000000, 0.000000000000000000 ) ) ;
#10324=AXIS2_PLACEMENT_3D ( 'NONE', #3805, #11375, #16269 ) ;
#10326=CARTESIAN_POINT ( 'NONE',  ( 49.86468353125001585, 30.75937500034139305, 16.20201782572375038 ) ) ;
#10331=CARTESIAN_POINT ( 'NONE',  ( 46.38089879718482678, 25.00000000000000000, -18.31192695794318226 ) ) ;
#10332=CARTESIAN_POINT ( 'NONE',  ( 15.40903463028481113, 31.32187500034139305, -47.42413220539094709 ) ) ;
#10340=CARTESIAN_POINT ( 'NONE',  ( -15.40903463028480580, 32.32187500034139305, 47.42413220539094709 ) ) ;
#10342=CARTESIAN_POINT ( 'NONE',  ( 30.81806926056964002, 38.55937500034139731, 42.41743335407646498 ) ) ;
#10346=CARTESIAN_POINT ( 'NONE',  ( -3.210462471511496205E-15, 49.35937500034138736, -52.43083105670540789 ) ) ;
#10349=CARTESIAN_POINT ( 'NONE',  ( -30.81806926056962226, 24.22187500034139163, 42.41743335407647919 ) ) ;
#10354=CARTESIAN_POINT ( 'NONE',  ( -49.99999999999999289, 46.09999999999999432, 16.24598481164533226 ) ) ;
#10356=CARTESIAN_POINT ( 'NONE',  ( 49.86468353125000164, 48.92187500034139447, -6.106662507704105588E-15 ) ) ;
#10357=EDGE_CURVE ( 'NONE', #11210, #7740, #8586, .T. ) ;
#10362=CARTESIAN_POINT ( 'NONE',  ( -15.45084971874736368, 38.18125000068280173, 47.55282581475768211 ) ) ;
#10368=CARTESIAN_POINT ( 'NONE',  ( 9.631387414534489405E-15, 46.42187500034139447, 52.43083105670540789 ) ) ;
#10380=CARTESIAN_POINT ( 'NONE',  ( -3.111920190527341144E-15, 29.28125000068279604, -50.00000000000000000 ) ) ;
#10382=CARTESIAN_POINT ( 'NONE',  ( -49.86468353124999453, 47.82187500034140015, -16.20201782572375393 ) ) ;
#10384=CARTESIAN_POINT ( 'NONE',  ( -3.111920190527341144E-15, 25.50000000000000355, -50.00000000000000000 ) ) ;
#10393=CARTESIAN_POINT ( 'NONE',  ( 7.919222016226807881, 49.22999571913593542, -50.00000000000000000 ) ) ;
#10396=CARTESIAN_POINT ( 'NONE',  ( 0.000000000000000000, 272.0000000000000000, 0.000000000000000000 ) ) ;
#10398=CARTESIAN_POINT ( 'NONE',  ( -49.99999999999999289, 37.88125000068279746, 16.24598481164533226 ) ) ;
#10400=CARTESIAN_POINT ( 'NONE',  ( -30.90169943749474868, 23.69999999999999929, -42.53254041760200721 ) ) ;
#10404=CARTESIAN_POINT ( 'NONE',  ( 9.631387414534489405E-15, 38.35937500034139447, 52.43083105670540789 ) ) ;
#10408=DIRECTION ( 'NONE',  ( -0.000000000000000000, -1.000000000000000000, -0.000000000000000000 ) ) ;
#10409=CARTESIAN_POINT ( 'NONE',  ( 49.86468353125000164, 30.85937500034139802, -6.106662507704105588E-15 ) ) ;
#10411=CARTESIAN_POINT ( 'NONE',  ( 8.446640517145639571E-15, 26.50000000000000000, 50.00000000000000000 ) ) ;
#10414=CARTESIAN_POINT ( 'NONE',  ( -49.86468353124999453, 33.82187500034138594, -16.20201782572375393 ) ) ;
#10424=CARTESIAN_POINT ( 'NONE',  ( -30.81806926056963292, 27.62187500034139731, -42.41743335407647209 ) ) ;
#10427=CARTESIAN_POINT ( 'NONE',  ( -49.86468353124999453, 27.75937500034139660, -16.20201782572375393 ) ) ;
#10430=CARTESIAN_POINT ( 'NONE',  ( -40.34137639590981195, 46.05937500034139731, 29.30972558990012189 ) ) ;
#10437=CARTESIAN_POINT ( 'NONE',  ( 30.90169943749475578, 42.69999999999999574, 42.53254041760200010 ) ) ;
#10440=CARTESIAN_POINT ( 'NONE',  ( -15.40903463028480580, 48.32187500034140015, 47.42413220539094709 ) ) ;
#10444=CARTESIAN_POINT ( 'NONE',  ( -15.45084971874737256, 37.38125000068279746, -47.55282581475767500 ) ) ;
#10448=LINE ( 'NONE', #1706, #10766 ) ;
#10449=CARTESIAN_POINT ( 'NONE',  ( 49.99999999999999289, 32.88125000068280457, -16.24598481164532160 ) ) ;
#10450=CARTESIAN_POINT ( 'NONE',  ( -49.86468353124999453, 45.82187500034140015, -16.20201782572375393 ) ) ;
#10452=CARTESIAN_POINT ( 'NONE',  ( 0.000000000000000000, 193.4213562373095385, 0.000000000000000000 ) ) ;
#10455=CARTESIAN_POINT ( 'NONE',  ( 49.40314992384931259, 25.00000000000000000, -8.200154929058095732 ) ) ;
#10460=CARTESIAN_POINT ( 'NONE',  ( 9.631387414534489405E-15, 46.42187500034139447, 52.43083105670540789 ) ) ;
#10468=CARTESIAN_POINT ( 'NONE',  ( 30.90169943749473802, 29.30000000000000071, -42.53254041760200721 ) ) ;
#10478=LINE ( 'NONE', #8057, #5538 ) ;
#10482=CARTESIAN_POINT ( 'NONE',  ( -15.40903463028481646, 37.45937500034139589, -47.42413220539093999 ) ) ;
#10487=CARTESIAN_POINT ( 'NONE',  ( -30.90169943749474868, 47.48125000068279178, -42.53254041760200721 ) ) ;
#10489=CARTESIAN_POINT ( 'NONE',  ( -30.81806926056962226, 20.15937500034139518, 42.41743335407647919 ) ) ;
#10493=DIRECTION ( 'NONE',  ( 0.000000000000000000, 1.000000000000000000, 0.000000000000000000 ) ) ;
#10497=CARTESIAN_POINT ( 'NONE',  ( -30.81806926056962226, 26.22187500034139518, 42.41743335407647209 ) ) ;
#10498=AXIS2_PLACEMENT_3D ( 'NONE', #15462, #9402, #9154 ) ;
#10505=CARTESIAN_POINT ( 'NONE',  ( -30.90169943749473802, 36.29999999999998295, 42.53254041760200721 ) ) ;
#10508=ORIENTED_EDGE ( 'NONE', *, *, #13723, .F. ) ;
#10510=CARTESIAN_POINT ( 'NONE',  ( -30.81806926056962226, 28.15937500034139518, 42.41743335407647209 ) ) ;
#10514=CARTESIAN_POINT ( 'NONE',  ( 0.000000000000000000, 193.4213562373095385, 0.000000000000000000 ) ) ;
#10515=CARTESIAN_POINT ( 'NONE',  ( -15.40903463028481646, 43.45937500034139589, -47.42413220539093999 ) ) ;
#10526=CARTESIAN_POINT ( 'NONE',  ( -3.219174618344376363E-15, 39.49999999999999289, -52.57311121191334990 ) ) ;
#10528=CARTESIAN_POINT ( 'NONE',  ( -40.34137639590981905, 43.72187500034139873, -29.30972558990011478 ) ) ;
#10531=CARTESIAN_POINT ( 'NONE',  ( 30.81806926056962936, 47.15937500034139163, -42.41743335407646498 ) ) ;
#10532=ORIENTED_EDGE ( 'NONE', *, *, #3632, .F. ) ;
#10535=CIRCLE ( 'NONE', #7610, 65.15972704814865324 ) ;
#10536=CARTESIAN_POINT ( 'NONE',  ( -30.90169943749473802, 38.08125000068280031, 42.53254041760200721 ) ) ;
#10541=LINE ( 'NONE', #8028, #13691 ) ;
#10542=CARTESIAN_POINT ( 'NONE',  ( -49.86468353125000164, 45.92187500034139447, 0.000000000000000000 ) ) ;
#10554=CARTESIAN_POINT ( 'NONE',  ( 40.34137639590981905, 20.65937500034139873, 29.30972558990010768 ) ) ;
#10560=CARTESIAN_POINT ( 'NONE',  ( 0.000000000000000000, 193.4213562373095385, -50.00000000000000000 ) ) ;
#10566=DIRECTION ( 'NONE',  ( 0.000000000000000000, 1.000000000000000000, 0.000000000000000000 ) ) ;
#10574=CARTESIAN_POINT ( 'NONE',  ( 49.86468353124999453, 34.95937500034138878, -16.20201782572376459 ) ) ;
#10579=CARTESIAN_POINT ( 'NONE',  ( -49.86468353124999453, 21.75937500034140015, -16.20201782572375393 ) ) ;
#10585=CARTESIAN_POINT ( 'NONE',  ( -30.81806926056962226, 30.22187500034139518, 42.41743335407647209 ) ) ;
#10592=CARTESIAN_POINT ( 'NONE',  ( -50.00000000000000000, 38.00000000000000711, 0.000000000000000000 ) ) ;
#10598=CARTESIAN_POINT ( 'NONE',  ( -40.34137639590981195, 28.05937500034139731, 29.30972558990012189 ) ) ;
#10601=CARTESIAN_POINT ( 'NONE',  ( -40.34137639590981195, 42.05937500034139731, 29.30972558990012189 ) ) ;
#10604=FACE_OUTER_BOUND ( 'NONE', #11407, .T. ) ;
#10610=CARTESIAN_POINT ( 'NONE',  ( 40.45084971874737789, 40.80000000000000426, 29.38926261462365375 ) ) ;
#10612=CARTESIAN_POINT ( 'NONE',  ( -15.40903463028480580, 42.32187500034139305, 47.42413220539094709 ) ) ;
#10615=DIRECTION ( 'NONE',  ( 0.000000000000000000, 0.000000000000000000, -1.000000000000000000 ) ) ;
#10617=CARTESIAN_POINT ( 'NONE',  ( 30.90169943749474157, 29.08125000068280031, -42.53254041760200721 ) ) ;
#10625=DIRECTION ( 'NONE',  ( -0.000000000000000000, -1.000000000000000000, -0.000000000000000000 ) ) ;
#10627=CIRCLE ( 'NONE', #5589, 63.16733765196516970 ) ;
#10632=CARTESIAN_POINT ( 'NONE',  ( -49.86468353124999453, 41.82187500034140015, -16.20201782572375393 ) ) ;
#10633=EDGE_CURVE ( 'NONE', #2524, #14905, #1203, .T. ) ;
#10641=CARTESIAN_POINT ( 'NONE',  ( 50.00000000000000711, 48.68125000068279462, 16.24598481164530739 ) ) ;
#10642=LINE ( 'NONE', #393, #10865 ) ;
#10643=CARTESIAN_POINT ( 'NONE',  ( -40.45084971874737079, 46.20000000000000284, 29.38926261462367151 ) ) ;
#10644=CARTESIAN_POINT ( 'NONE',  ( 7.919222016226822092, 48.55125428154684641, 49.99999999999999289 ) ) ;
#10646=( BOUNDED_CURVE ( )  B_SPLINE_CURVE ( 2, ( #10380, #15356, #11532, #10300, #7877, #5398, #13033, #3976, #9125, #7796, #10213, #9299, #2894 ),
 .UNSPECIFIED., .F., .F. ) 
 B_SPLINE_CURVE_WITH_KNOTS ( ( 3, 2, 2, 2, 2, 2, 3 ),
 ( 0.6833333333333333481, 0.6866666666666666474, 0.6933333333333333570, 0.6999999999999999556, 0.7066666666666666652, 0.7133333333333333748, 0.7166666666666666741 ),
 .UNSPECIFIED. ) 
 CURVE ( )  GEOMETRIC_REPRESENTATION_ITEM ( )  RATIONAL_B_SPLINE_CURVE ( ( 0.9755282581475768211, 0.9755282581475768211, 1.000000000000000000, 0.9510565162951535312, 1.000000000000000000, 0.9510565162951535312, 1.000000000000000000, 0.9510565162951535312, 1.000000000000000000, 0.9510565162951535312, 1.000000000000000000, 0.9755282581475768211, 0.9755282581475768211 ) ) 
 REPRESENTATION_ITEM ( '' )  );
#10651=CARTESIAN_POINT ( 'NONE',  ( 30.81806926056964002, 40.55937500034139731, 42.41743335407647209 ) ) ;
#10652=ORIENTED_EDGE ( 'NONE', *, *, #41, .T. ) ;
#10653=EDGE_LOOP ( 'NONE', ( #8197, #7479 ) ) ;
#10654=CARTESIAN_POINT ( 'NONE',  ( -49.99999999999999289, 47.68125000068280173, -16.24598481164531449 ) ) ;
#10656=CARTESIAN_POINT ( 'NONE',  ( 9.631387414534489405E-15, 24.35937500034139802, 52.43083105670540789 ) ) ;
#10658=CARTESIAN_POINT ( 'NONE',  ( -15.45084971874737256, 47.60000000000000142, -47.55282581475767500 ) ) ;
#10661=CARTESIAN_POINT ( 'NONE',  ( 30.81806926056962936, 25.22187500034139873, -42.41743335407646498 ) ) ;
#10669=CARTESIAN_POINT ( 'NONE',  ( 40.45084971874737079, 37.20000000000000284, -29.38926261462366440 ) ) ;
#10673=CARTESIAN_POINT ( 'NONE',  ( 9.631387414534489405E-15, 30.35937500034139092, 52.43083105670540789 ) ) ;
#10677=CARTESIAN_POINT ( 'NONE',  ( 49.86468353125000164, 44.85937500034140157, -6.106662507704105588E-15 ) ) ;
#10683=CARTESIAN_POINT ( 'NONE',  ( -30.90169943749474868, 39.70000000000000284, -42.53254041760200721 ) ) ;
#10685=CARTESIAN_POINT ( 'NONE',  ( -15.40903463028481646, 41.52187500034139589, -47.42413220539093999 ) ) ;
#10688=CARTESIAN_POINT ( 'NONE',  ( 49.86468353125001585, 46.75937500034140015, 16.20201782572375038 ) ) ;
#10690=CARTESIAN_POINT ( 'NONE',  ( 30.90169943749475578, 28.48125000068280244, 42.53254041760200010 ) ) ;
#10692=CYLINDRICAL_SURFACE ( 'NONE', #5218, 50.00000000000000000 ) ;
#10696=CARTESIAN_POINT ( 'NONE',  ( -3.210462471511496205E-15, 41.42187500034139447, -52.43083105670540789 ) ) ;
#10704=CARTESIAN_POINT ( 'NONE',  ( -49.86468353124999453, 43.82187500034140015, -16.20201782572375393 ) ) ;
#10705=VERTEX_POINT ( 'NONE', #2730 ) ;
#10711=CYLINDRICAL_SURFACE ( 'NONE', #16195, 50.00000000000000000 ) ;
#10716=CARTESIAN_POINT ( 'NONE',  ( -49.99999999999999289, 33.88125000068280457, 16.24598481164533226 ) ) ;
#10718=FACE_OUTER_BOUND ( 'NONE', #13337, .T. ) ;
#10723=CARTESIAN_POINT ( 'NONE',  ( 30.81806926056962936, 33.15937500034139873, -42.41743335407647209 ) ) ;
#10727=EDGE_CURVE ( 'NONE', #15172, #2810, #684, .T. ) ;
#10729=CARTESIAN_POINT ( 'NONE',  ( -3.219174618344376363E-15, 49.28125000068278894, -52.57311121191334990 ) ) ;
#10732=CARTESIAN_POINT ( 'NONE',  ( -30.81806926056963292, 23.55937500034139376, -42.41743335407647209 ) ) ;
#10733=ORIENTED_EDGE ( 'NONE', *, *, #2952, .T. ) ;
#10737=CARTESIAN_POINT ( 'NONE',  ( -40.34137639590981195, 28.12187500034139731, 29.30972558990012189 ) ) ;
#10745=AXIS2_PLACEMENT_3D ( 'NONE', #6728, #5478, #11774 ) ;
#10746=CARTESIAN_POINT ( 'NONE',  ( -3.219174618344376363E-15, 35.50000000000000000, -52.57311121191334990 ) ) ;
#10748=CARTESIAN_POINT ( 'NONE',  ( -49.86468353124999453, 47.75937500034139305, -16.20201782572375393 ) ) ;
#10749=ORIENTED_EDGE ( 'NONE', *, *, #7880, .F. ) ;
#10750=CARTESIAN_POINT ( 'NONE',  ( -49.86468353125000164, 31.85937500034139447, 0.000000000000000000 ) ) ;
#10753=CARTESIAN_POINT ( 'NONE',  ( 49.86468353124999453, 44.95937500034139589, -16.20201782572376459 ) ) ;
#10761=CARTESIAN_POINT ( 'NONE',  ( -49.86468353125000164, 29.92187500034139802, 0.000000000000000000 ) ) ;
#10762=CARTESIAN_POINT ( 'NONE',  ( -49.99999999999999289, 41.90000000000001279, -16.24598481164531449 ) ) ;
#10764=CARTESIAN_POINT ( 'NONE',  ( 9.631387414534489405E-15, 42.42187500034140157, 52.43083105670540789 ) ) ;
#10766=VECTOR ( 'NONE', #2882, 1000.000000000000000 ) ;
#10769=CARTESIAN_POINT ( 'NONE',  ( 0.000000000000000000, 193.4213562373095385, 0.000000000000000000 ) ) ;
#10772=CARTESIAN_POINT ( 'NONE',  ( 15.45084971874737789, 28.38125000068279746, 47.55282581475767500 ) ) ;
#10774=CIRCLE ( 'NONE', #8920, 50.00000000000000000 ) ;
#10778=CARTESIAN_POINT ( 'NONE',  ( -49.86468353125000164, 37.92187500034140157, 0.000000000000000000 ) ) ;
#10793=CARTESIAN_POINT ( 'NONE',  ( 30.81806926056962936, 45.22187500034139873, -42.41743335407647209 ) ) ;
#10806=CARTESIAN_POINT ( 'NONE',  ( -49.99999999999999289, 30.10000000000000497, 16.24598481164533226 ) ) ;
#10813=CARTESIAN_POINT ( 'NONE',  ( -49.86468353125000164, 33.85937500034139447, 0.000000000000000000 ) ) ;
#10818=CARTESIAN_POINT ( 'NONE',  ( 15.45084971874737789, 44.38125000068279746, 47.55282581475767500 ) ) ;
#10820=CARTESIAN_POINT ( 'NONE',  ( 49.86468353125000164, 20.85937500034139802, -6.106662507704105588E-15 ) ) ;
#10821=EDGE_LOOP ( 'NONE', ( #15879, #3410, #12272, #8528 ) ) ;
#10823=DIRECTION ( 'NONE',  ( 0.000000000000000000, 0.000000000000000000, 1.000000000000000000 ) ) ;
#10824=CARTESIAN_POINT ( 'NONE',  ( -3.111920190527341144E-15, 45.28125000068279604, -50.00000000000000000 ) ) ;
#10825=CARTESIAN_POINT ( 'NONE',  ( -15.40903463028481646, 29.52187500034139589, -47.42413220539093999 ) ) ;
#10831=CARTESIAN_POINT ( 'NONE',  ( -30.90169943749474868, 31.70000000000000639, -42.53254041760200721 ) ) ;
#10836=ADVANCED_FACE ( 'NONE', ( #12795 ), #7728, .T. ) ;
#10838=DIRECTION ( 'NONE',  ( 0.000000000000000000, 0.000000000000000000, -1.000000000000000000 ) ) ;
#10840=CARTESIAN_POINT ( 'NONE',  ( 30.81806926056962936, 43.15937500034140584, -42.41743335407647209 ) ) ;
#10846=CARTESIAN_POINT ( 'NONE',  ( 40.34137639590981195, 33.12187500034139731, -29.30972558990011834 ) ) ;
#10849=CARTESIAN_POINT ( 'NONE',  ( 15.40903463028481113, 43.32187500034139305, -47.42413220539094709 ) ) ;
#10852=CARTESIAN_POINT ( 'NONE',  ( 9.631387414534489405E-15, 48.35937500034139447, 52.43083105670540789 ) ) ;
#10855=CARTESIAN_POINT ( 'NONE',  ( 15.45084971874736723, 31.18125000068279817, -47.55282581475768211 ) ) ;
#10858=CARTESIAN_POINT ( 'NONE',  ( 40.34137639590981195, 41.12187500034139731, -29.30972558990011834 ) ) ;
#10860=CARTESIAN_POINT ( 'NONE',  ( -49.99999999999999289, 39.68125000068280173, -16.24598481164531449 ) ) ;
#10865=VECTOR ( 'NONE', #4245, 1000.000000000000000 ) ;
#10868=EDGE_LOOP ( 'NONE', ( #3816, #1875, #4574, #4686 ) ) ;
#10869=CARTESIAN_POINT ( 'NONE',  ( -15.40903463028481646, 39.52187500034139589, -47.42413220539093999 ) ) ;
#10872=ORIENTED_EDGE ( 'NONE', *, *, #8453, .F. ) ;
#10875=CARTESIAN_POINT ( 'NONE',  ( -1.240322475938754499E-13, 40.50000000000000000, 50.00000000000000000 ) ) ;
#10882=FACE_OUTER_BOUND ( 'NONE', #6197, .T. ) ;
#10885=CARTESIAN_POINT ( 'NONE',  ( 50.00000000000000000, 37.00000000000000711, -6.123233995736766085E-15 ) ) ;
#10886=VERTEX_POINT ( 'NONE', #6135 ) ;
#10887=EDGE_CURVE ( 'NONE', #15132, #14942, #3407, .T. ) ;
#10888=CARTESIAN_POINT ( 'NONE',  ( 49.86468353125000164, 32.85937500034139447, -6.106662507704105588E-15 ) ) ;
#10892=CARTESIAN_POINT ( 'NONE',  ( -30.90169943749473802, 44.08125000068279320, 42.53254041760200721 ) ) ;
#10902=CARTESIAN_POINT ( 'NONE',  ( 15.45084971874736723, 39.40000000000000568, -47.55282581475768211 ) ) ;
#10908=CARTESIAN_POINT ( 'NONE',  ( -49.99999999999999289, 28.10000000000000497, 16.24598481164533226 ) ) ;
#10910=CARTESIAN_POINT ( 'NONE',  ( 40.34137639590981195, 49.05937500034139731, -29.30972558990011834 ) ) ;
#10913=LINE ( 'NONE', #6256, #14989 ) ;
#10916=CARTESIAN_POINT ( 'NONE',  ( -49.86468353124999453, 33.95937500034139589, 16.20201782572377525 ) ) ;
#10924=CARTESIAN_POINT ( 'NONE',  ( 49.86468353125000164, 30.92187500034139802, -6.106662507704105588E-15 ) ) ;
#10927=CARTESIAN_POINT ( 'NONE',  ( -3.210462471511496205E-15, 37.42187500034140157, -52.43083105670540789 ) ) ;
#10931=CARTESIAN_POINT ( 'NONE',  ( -49.86468353125000164, 39.85937500034139447, 0.000000000000000000 ) ) ;
#10933=CARTESIAN_POINT ( 'NONE',  ( -49.99999999999999289, 25.88125000068280102, 16.24598481164533226 ) ) ;
#10934=ORIENTED_EDGE ( 'NONE', *, *, #3807, .T. ) ;
#10935=CARTESIAN_POINT ( 'NONE',  ( -15.45084971874737256, 35.60000000000000142, -47.55282581475767500 ) ) ;
#10936=CARTESIAN_POINT ( 'NONE',  ( -30.81806926056963292, 41.62187500034139020, -42.41743335407646498 ) ) ;
#10938=CARTESIAN_POINT ( 'NONE',  ( 40.45084971874737079, 31.20000000000000284, -29.38926261462366440 ) ) ;
#10939=CARTESIAN_POINT ( 'NONE',  ( -49.86468353124999453, 22.02187500034139589, 16.20201782572377525 ) ) ;
#10946=CARTESIAN_POINT ( 'NONE',  ( -49.86468353124999453, 44.02187500034139589, 16.20201782572377525 ) ) ;
#10947=CARTESIAN_POINT ( 'NONE',  ( 2.600676159226420495E-13, 31.28125000068279604, -49.99999999999999289 ) ) ;
#10949=VERTEX_POINT ( 'NONE', #13841 ) ;
#10952=DIRECTION ( 'NONE',  ( -0.000000000000000000, -1.000000000000000000, -0.000000000000000000 ) ) ;
#10958=DIRECTION ( 'NONE',  ( 0.000000000000000000, 0.000000000000000000, 1.000000000000000000 ) ) ;
#10960=DIRECTION ( 'NONE',  ( 0.000000000000000000, -0.000000000000000000, 1.000000000000000000 ) ) ;
#10964=CARTESIAN_POINT ( 'NONE',  ( 50.00000000000000711, 36.89999999999999858, 16.24598481164530739 ) ) ;
#10966=CARTESIAN_POINT ( 'NONE',  ( 9.631387414534489405E-15, 32.35937500034139447, 52.43083105670540789 ) ) ;
#10969=ORIENTED_EDGE ( 'NONE', *, *, #9196, .F. ) ;
#10970=CARTESIAN_POINT ( 'NONE',  ( -50.00000000000000000, 41.78125000068280315, 0.000000000000000000 ) ) ;
#10979=FACE_OUTER_BOUND ( 'NONE', #13395, .T. ) ;
#10986=CARTESIAN_POINT ( 'NONE',  ( 0.000000000000000000, 193.4213562373095385, 0.000000000000000000 ) ) ;
#10987=CARTESIAN_POINT ( 'NONE',  ( 30.90169943749474157, 29.30000000000000071, -42.53254041760200721 ) ) ;
#10990=EDGE_CURVE ( 'NONE', #3473, #15357, #5126, .T. ) ;
#10992=EDGE_CURVE ( 'NONE', #12352, #7158, #11069, .T. ) ;
#10993=CARTESIAN_POINT ( 'NONE',  ( -49.86468353125000164, 47.85937500034139447, 0.000000000000000000 ) ) ;
#10996=CARTESIAN_POINT ( 'NONE',  ( 40.34137639590981195, 25.05937500034139376, -29.30972558990011834 ) ) ;
#11000=CARTESIAN_POINT ( 'NONE',  ( -40.34137639590981195, 38.05937500034139731, 29.30972558990012189 ) ) ;
#11001=LINE ( 'NONE', #924, #1488 ) ;
#11007=CARTESIAN_POINT ( 'NONE',  ( -40.34137639590981905, 31.72187500034139873, -29.30972558990011478 ) ) ;
#11008=CARTESIAN_POINT ( 'NONE',  ( 50.00000000000000000, 33.00000000000000000, -6.123233995736766085E-15 ) ) ;
#11010=CARTESIAN_POINT ( 'NONE',  ( -3.210462471511496205E-15, 39.42187500034140157, -52.43083105670540789 ) ) ;
#11014=CARTESIAN_POINT ( 'NONE',  ( -30.81806926056963292, 45.55937500034139731, -42.41743335407646498 ) ) ;
#11017=CARTESIAN_POINT ( 'NONE',  ( 9.657523855033129090E-15, 22.28125000068279959, 52.57311121191334990 ) ) ;
#11019=CARTESIAN_POINT ( 'NONE',  ( -1.240322475938754499E-13, 36.50000000000000711, 50.00000000000000000 ) ) ;
#11020=CARTESIAN_POINT ( 'NONE',  ( -30.81806926056962226, 40.22187500034139873, 42.41743335407647209 ) ) ;
#11022=CARTESIAN_POINT ( 'NONE',  ( 30.90169943749473802, 41.30000000000000426, -42.53254041760200721 ) ) ;
#11024=CARTESIAN_POINT ( 'NONE',  ( 49.86468353125000164, 20.92187500034139802, -6.106662507704105588E-15 ) ) ;
#11027=( BOUNDED_CURVE ( )  B_SPLINE_CURVE ( 2, ( #3571, #8626, #7232, #5990, #11386, #1136, #2315, #6230, #11058, #11301, #16363, #15111, #3736 ),
 .UNSPECIFIED., .F., .T. ) 
 B_SPLINE_CURVE_WITH_KNOTS ( ( 3, 2, 2, 2, 2, 2, 3 ),
 ( 0.05000000000000000278, 0.05333333333333333676, 0.05999999999999999778, 0.06666666666666666574, 0.07333333333333333370, 0.08000000000000000167, 0.08333333333333334259 ),
 .UNSPECIFIED. ) 
 CURVE ( )  GEOMETRIC_REPRESENTATION_ITEM ( )  RATIONAL_B_SPLINE_CURVE ( ( 0.9755282581475768211, 0.9755282581475768211, 1.000000000000000000, 0.9510565162951535312, 1.000000000000000000, 0.9510565162951535312, 1.000000000000000000, 0.9510565162951535312, 1.000000000000000000, 0.9510565162951535312, 1.000000000000000000, 0.9755282581475767101, 0.9755282581475768211 ) ) 
 REPRESENTATION_ITEM ( '' )  );
#11031=CARTESIAN_POINT ( 'NONE',  ( -49.86468353124999453, 38.02187500034140299, 16.20201782572377525 ) ) ;
#11034=ORIENTED_EDGE ( 'NONE', *, *, #12206, .T. ) ;
#11046=( NAMED_UNIT ( * ) SI_UNIT ( $, .STERADIAN. ) SOLID_ANGLE_UNIT ( ) );
#11049=DIRECTION ( 'NONE',  ( -0.000000000000000000, -1.000000000000000000, -0.000000000000000000 ) ) ;
#11052=CARTESIAN_POINT ( 'NONE',  ( 49.99999999999999289, 42.88125000068279036, -16.24598481164532160 ) ) ;
#11056=CARTESIAN_POINT ( 'NONE',  ( 15.40903463028482356, 32.45937500034138878, 47.42413220539093999 ) ) ;
#11058=CARTESIAN_POINT ( 'NONE',  ( -40.45084971874737789, 47.58125000068280031, -29.38926261462365730 ) ) ;
#11061=CARTESIAN_POINT ( 'NONE',  ( 49.99999999999999289, 40.88125000068279036, -16.24598481164532160 ) ) ;
#11066=CYLINDRICAL_SURFACE ( 'NONE', #3452, 50.00000000000000000 ) ;
#11069=( BOUNDED_CURVE ( )  B_SPLINE_CURVE ( 2, ( #3387, #8454, #16103, #9793, #13517, #14841, #2121, #11206, #7210, #12271, #4816, #3470, #9869 ),
 .UNSPECIFIED., .F., .F. ) 
 B_SPLINE_CURVE_WITH_KNOTS ( ( 3, 2, 2, 2, 2, 2, 3 ),
 ( 0.1833333333333333481, 0.1866666666666666752, 0.1933333333333333293, 0.2000000000000000111, 0.2066666666666666652, 0.2133333333333333470, 0.2166666666666666741 ),
 .UNSPECIFIED. ) 
 CURVE ( )  GEOMETRIC_REPRESENTATION_ITEM ( )  RATIONAL_B_SPLINE_CURVE ( ( 0.9755282581475767101, 0.9755282581475768211, 1.000000000000000000, 0.9510565162951535312, 1.000000000000000000, 0.9510565162951535312, 1.000000000000000000, 0.9510565162951535312, 1.000000000000000000, 0.9510565162951535312, 1.000000000000000000, 0.9755282581475768211, 0.9755282581475768211 ) ) 
 REPRESENTATION_ITEM ( '' )  );
#11073=DIRECTION ( 'NONE',  ( 0.000000000000000000, 0.000000000000000000, 1.000000000000000000 ) ) ;
#11077=CARTESIAN_POINT ( 'NONE',  ( -40.45084971874737079, 28.20000000000000284, 29.38926261462367151 ) ) ;
#11083=CARTESIAN_POINT ( 'NONE',  ( 30.81806926056964002, 48.55937500034138310, 42.41743335407647209 ) ) ;
#11087=VERTEX_POINT ( 'NONE', #13906 ) ;
#11089=CARTESIAN_POINT ( 'NONE',  ( -49.86468353125000164, 35.85937500034140157, 0.000000000000000000 ) ) ;
#11091=CARTESIAN_POINT ( 'NONE',  ( 15.45084971874736723, 41.18125000068280173, -47.55282581475768211 ) ) ;
#11096=EDGE_CURVE ( 'NONE', #4982, #495, #10535, .T. ) ;
#11097=DIRECTION ( 'NONE',  ( 0.000000000000000000, 0.000000000000000000, -1.000000000000000000 ) ) ;
#11106=CARTESIAN_POINT ( 'NONE',  ( 49.86468353125000164, 38.92187500034139447, -6.106662507704105588E-15 ) ) ;
#11110=CARTESIAN_POINT ( 'NONE',  ( -49.86468353125000164, 43.85937500034140157, 0.000000000000000000 ) ) ;
#11112=CARTESIAN_POINT ( 'NONE',  ( 49.99999999999999289, 26.88125000068280102, -16.24598481164532160 ) ) ;
#11114=CARTESIAN_POINT ( 'NONE',  ( -30.90169943749474513, 35.69999999999999574, -42.53254041760200721 ) ) ;
#11115=CARTESIAN_POINT ( 'NONE',  ( 49.86468353125001585, 34.82187500034139305, 16.20201782572375038 ) ) ;
#11118=CARTESIAN_POINT ( 'NONE',  ( 30.90169943749475223, 40.69999999999999574, 42.53254041760199300 ) ) ;
#11119=CARTESIAN_POINT ( 'NONE',  ( 49.86468353125000164, 24.92187500034139802, -6.106662507704105588E-15 ) ) ;
#11126=CARTESIAN_POINT ( 'NONE',  ( 49.86468353124999453, 37.02187500034138878, -16.20201782572376459 ) ) ;
#11140=( LENGTH_UNIT ( ) NAMED_UNIT ( * ) SI_UNIT ( .MILLI., .METRE. ) );
#11145=CARTESIAN_POINT ( 'NONE',  ( 15.40903463028482356, 22.45937500034139589, 47.42413220539093999 ) ) ;
#11149=CARTESIAN_POINT ( 'NONE',  ( 9.657523855033129090E-15, 42.28125000068278894, 52.57311121191334990 ) ) ;
#11152=FACE_OUTER_BOUND ( 'NONE', #402, .T. ) ;
#11161=CARTESIAN_POINT ( 'NONE',  ( 1.293669679204937499E-13, 37.28125000068280315, -50.00000000000000000 ) ) ;
#11162=CARTESIAN_POINT ( 'NONE',  ( -30.90169943749474513, 41.70000000000000284, -42.53254041760200721 ) ) ;
#11166=CARTESIAN_POINT ( 'NONE',  ( -40.45084971874737789, 27.80000000000000071, -29.38926261462365730 ) ) ;
#11170=CARTESIAN_POINT ( 'NONE',  ( 49.86468353124999453, 42.95937500034139589, -16.20201782572376459 ) ) ;
#11175=CARTESIAN_POINT ( 'NONE',  ( -15.40903463028480580, 32.25937500034140015, 47.42413220539094709 ) ) ;
#11176=ADVANCED_FACE ( 'NONE', ( #12070 ), #4445, .T. ) ;
#11177=FACE_OUTER_BOUND ( 'NONE', #16452, .T. ) ;
#11179=CARTESIAN_POINT ( 'NONE',  ( -6.668400408272873429E-15, 49.50000000000000000, -50.00000000000000000 ) ) ;
#11186=CARTESIAN_POINT ( 'NONE',  ( -30.81806926056962226, 40.22187500034139873, 42.41743335407647919 ) ) ;
#11187=( BOUNDED_CURVE ( )  B_SPLINE_CURVE ( 2, ( #13286, #14523, #8220, #5650, #4489, #10716, #394, #11794, #8297, #15777, #9555, #6906, #14286 ),
 .UNSPECIFIED., .F., .F. ) 
 B_SPLINE_CURVE_WITH_KNOTS ( ( 3, 2, 2, 2, 2, 2, 3 ),
 ( 0.5166666666666667185, 0.5200000000000000178, 0.5266666666666666163, 0.5333333333333333259, 0.5400000000000000355, 0.5466666666666666341, 0.5500000000000000444 ),
 .UNSPECIFIED. ) 
 CURVE ( )  GEOMETRIC_REPRESENTATION_ITEM ( )  RATIONAL_B_SPLINE_CURVE ( ( 0.9755282581475768211, 0.9755282581475771542, 1.000000000000000000, 0.9510565162951535312, 1.000000000000000000, 0.9510565162951535312, 1.000000000000000000, 0.9510565162951535312, 1.000000000000000000, 0.9510565162951535312, 1.000000000000000000, 0.9755282581475763770, 0.9755282581475768211 ) ) 
 REPRESENTATION_ITEM ( '' )  );
#11192=CARTESIAN_POINT ( 'NONE',  ( 30.81806926056962936, 45.15937500034139873, -42.41743335407646498 ) ) ;
#11194=CARTESIAN_POINT ( 'NONE',  ( 50.00000000000000000, 22.78125000068279959, -6.123233995736766085E-15 ) ) ;
#11198=CARTESIAN_POINT ( 'NONE',  ( 30.90169943749473802, 31.30000000000000071, -42.53254041760200721 ) ) ;
#11200=CARTESIAN_POINT ( 'NONE',  ( -30.81806926056963292, 21.62187500034139376, -42.41743335407647209 ) ) ;
#11205=CARTESIAN_POINT ( 'NONE',  ( -15.40903463028481646, 35.52187500034139589, -47.42413220539093999 ) ) ;
#11206=CARTESIAN_POINT ( 'NONE',  ( -49.99999999999999289, 43.68125000068280173, -16.24598481164531449 ) ) ;
#11210=VERTEX_POINT ( 'NONE', #15728 ) ;
#11212=CARTESIAN_POINT ( 'NONE',  ( 49.99999999999999289, 45.10000000000000142, -16.24598481164532160 ) ) ;
#11213=CARTESIAN_POINT ( 'NONE',  ( 0.000000000000000000, 193.4213562373095385, 0.000000000000000000 ) ) ;
#11219=CARTESIAN_POINT ( 'NONE',  ( -49.99999999999999289, 35.68125000068279462, -16.24598481164531449 ) ) ;
#11221=CARTESIAN_POINT ( 'NONE',  ( 15.40903463028481113, 23.25937500034139660, -47.42413220539094709 ) ) ;
#11227=CARTESIAN_POINT ( 'NONE',  ( -40.45084971874737079, 39.98125000068279888, 29.38926261462367151 ) ) ;
#11229=LINE ( 'NONE', #11307, #4383 ) ;
#11240=CARTESIAN_POINT ( 'NONE',  ( 40.45084971874737079, 49.20000000000000284, -29.38926261462366440 ) ) ;
#11242=DIRECTION ( 'NONE',  ( 0.000000000000000000, 0.000000000000000000, -1.000000000000000000 ) ) ;
#11243=CARTESIAN_POINT ( 'NONE',  ( -50.00000000000000000, 30.00000000000000355, 0.000000000000000000 ) ) ;
#11246=CARTESIAN_POINT ( 'NONE',  ( 30.81806926056962936, 47.15937500034138452, -42.41743335407647209 ) ) ;
#11251=CARTESIAN_POINT ( 'NONE',  ( -40.34137639590981195, 36.05937500034139731, 29.30972558990012189 ) ) ;
#11256=CARTESIAN_POINT ( 'NONE',  ( 46.06840506420055448, 24.99999999999999289, -19.08445694769665124 ) ) ;
#11257=CARTESIAN_POINT ( 'NONE',  ( 50.00000000000000000, 46.78125000068279604, -6.123233995736766085E-15 ) ) ;
#11262=CARTESIAN_POINT ( 'NONE',  ( -2.547328955960238000E-13, 30.28125000068279604, 49.99999999999999289 ) ) ;
#11266=CARTESIAN_POINT ( 'NONE',  ( 49.86468353125001585, 38.82187500034140015, 16.20201782572375038 ) ) ;
#11269=CARTESIAN_POINT ( 'NONE',  ( -3.210462471511496205E-15, 43.35937500034139447, -52.43083105670540789 ) ) ;
#11270=ORIENTED_EDGE ( 'NONE', *, *, #13663, .T. ) ;
#11271=CARTESIAN_POINT ( 'NONE',  ( 15.45084971874737789, 24.38125000068279746, 47.55282581475767500 ) ) ;
#11276=CARTESIAN_POINT ( 'NONE',  ( 50.00000000000000000, 31.00000000000000355, -6.123233995736766085E-15 ) ) ;
#11277=CARTESIAN_POINT ( 'NONE',  ( -50.00000000000000000, 50.00000000000000000, 0.000000000000000000 ) ) ;
#11282=CARTESIAN_POINT ( 'NONE',  ( -49.86468353125000164, 33.92187500034139447, 0.000000000000000000 ) ) ;
#11286=CARTESIAN_POINT ( 'NONE',  ( -7.919222016226688865, 31.55125428154684286, -50.00000000000003553 ) ) ;
#11289=DIRECTION ( 'NONE',  ( -0.000000000000000000, -1.000000000000000000, -0.000000000000000000 ) ) ;
#11295=DIRECTION ( 'NONE',  ( 0.000000000000000000, 1.000000000000000000, 0.000000000000000000 ) ) ;
#11300=CARTESIAN_POINT ( 'NONE',  ( 30.81806926056964002, 26.55937500034139376, 42.41743335407647209 ) ) ;
#11301=CARTESIAN_POINT ( 'NONE',  ( -30.90169943749474513, 47.48125000068279888, -42.53254041760200721 ) ) ;
#11305=CARTESIAN_POINT ( 'NONE',  ( -3.219174618344376363E-15, 39.28125000068279604, -52.57311121191334990 ) ) ;
#11307=CARTESIAN_POINT ( 'NONE',  ( 6.123233995736766085E-15, 193.4213562373095385, 50.00000000000000000 ) ) ;
#11321=CARTESIAN_POINT ( 'NONE',  ( 15.45084971874736723, 21.40000000000000213, -47.55282581475768211 ) ) ;
#11323=CARTESIAN_POINT ( 'NONE',  ( -3.111920190527341144E-15, 43.50000000000000711, -50.00000000000000000 ) ) ;
#11324=CARTESIAN_POINT ( 'NONE',  ( -49.86468353125000164, 41.85937500034139447, 0.000000000000000000 ) ) ;
#11333=CARTESIAN_POINT ( 'NONE',  ( -49.86468353125000164, 27.85937500034139447, 0.000000000000000000 ) ) ;
#11335=CARTESIAN_POINT ( 'NONE',  ( -50.00000000000000000, 49.78125000068280315, 0.000000000000000000 ) ) ;
#11336=CARTESIAN_POINT ( 'NONE',  ( 46.44184698740882311, 25.00000000000000000, -18.15679736478467987 ) ) ;
#11337=CARTESIAN_POINT ( 'NONE',  ( 7.919222016226693306, 30.33250428222964246, 50.00000000000003553 ) ) ;
#11347=CARTESIAN_POINT ( 'NONE',  ( 49.86468353125001585, 28.82187500034139305, 16.20201782572375038 ) ) ;
#11351=CARTESIAN_POINT ( 'NONE',  ( 15.40903463028482356, 36.45937500034139589, 47.42413220539093999 ) ) ;
#11355=CARTESIAN_POINT ( 'NONE',  ( 15.40903463028481113, 45.25937500034140015, -47.42413220539094709 ) ) ;
#11357=CARTESIAN_POINT ( 'NONE',  ( 40.34137639590981195, 25.12187500034139376, -29.30972558990011834 ) ) ;
#11358=CARTESIAN_POINT ( 'NONE',  ( 0.000000000000000000, 52.00000000000000711, 0.000000000000000000 ) ) ;
#11360=CARTESIAN_POINT ( 'NONE',  ( -30.90169943749473447, 26.08125000068279320, 42.53254041760200721 ) ) ;
#11361=CARTESIAN_POINT ( 'NONE',  ( 15.45084971874736723, 49.39999999999999858, -47.55282581475768211 ) ) ;
#11363=CARTESIAN_POINT ( 'NONE',  ( -15.40903463028481646, 49.52187500034140299, -47.42413220539093999 ) ) ;
#11366=DIRECTION ( 'NONE',  ( 0.000000000000000000, 0.000000000000000000, 1.000000000000000000 ) ) ;
#11369=ORIENTED_EDGE ( 'NONE', *, *, #13093, .F. ) ;
#11371=CARTESIAN_POINT ( 'NONE',  ( 40.45084971874737079, 45.20000000000000284, -29.38926261462366440 ) ) ;
#11375=DIRECTION ( 'NONE',  ( 0.000000000000000000, 1.000000000000000000, 0.000000000000000000 ) ) ;
#11379=CARTESIAN_POINT ( 'NONE',  ( -15.45084971874737256, 39.60000000000000142, -47.55282581475767500 ) ) ;
#11382=CARTESIAN_POINT ( 'NONE',  ( 38.60409515610501074, 25.00000000000000000, -31.77615201968907144 ) ) ;
#11383=ORIENTED_EDGE ( 'NONE', *, *, #8247, .F. ) ;
#11384=CARTESIAN_POINT ( 'NONE',  ( 30.81806926056964002, 22.55937500034139020, 42.41743335407647209 ) ) ;
#11385=VERTEX_POINT ( 'NONE', #13484 ) ;
#11386=CARTESIAN_POINT ( 'NONE',  ( -40.45084971874737079, 47.98125000068279888, 29.38926261462367151 ) ) ;
#11396=DIRECTION ( 'NONE',  ( 0.000000000000000000, 0.000000000000000000, -1.000000000000000000 ) ) ;
#11402=CARTESIAN_POINT ( 'NONE',  ( 40.45084971874737079, 21.19999999999999929, -29.38926261462366440 ) ) ;
#11405=CARTESIAN_POINT ( 'NONE',  ( 30.81806926056962936, 41.15937500034139873, -42.41743335407647209 ) ) ;
#11407=EDGE_LOOP ( 'NONE', ( #2607, #2123, #12380, #12045, #15407, #7661 ) ) ;
#11408=EDGE_CURVE ( 'NONE', #14050, #14905, #4691, .T. ) ;
#11412=CARTESIAN_POINT ( 'NONE',  ( -40.34137639590981195, 32.05937500034139731, 29.30972558990012189 ) ) ;
#11414=CARTESIAN_POINT ( 'NONE',  ( 0.000000000000000000, 54.00000000000000711, 63.16733765196516970 ) ) ;
#11416=CARTESIAN_POINT ( 'NONE',  ( 47.79496856443405761, 24.99999999999999289, -14.21716018044656238 ) ) ;
#11417=CARTESIAN_POINT ( 'NONE',  ( -49.86468353125000164, 35.92187500034140157, 0.000000000000000000 ) ) ;
#11425=CARTESIAN_POINT ( 'NONE',  ( 30.81806926056964002, 34.62187500034139731, 42.41743335407647209 ) ) ;
#11429=CARTESIAN_POINT ( 'NONE',  ( 49.86468353124999453, 34.95937500034138878, -16.20201782572376104 ) ) ;
#11430=ORIENTED_EDGE ( 'NONE', *, *, #5900, .T. ) ;
#11434=CARTESIAN_POINT ( 'NONE',  ( 40.34137639590981195, 45.05937500034139731, -29.30972558990011834 ) ) ;
#11436=CARTESIAN_POINT ( 'NONE',  ( -3.210462471511496205E-15, 21.42187500034139802, -52.43083105670540789 ) ) ;
#11439=DIRECTION ( 'NONE',  ( 0.000000000000000000, 0.000000000000000000, 1.000000000000000000 ) ) ;
#11440=CARTESIAN_POINT ( 'NONE',  ( 50.00000000000000000, 47.00000000000000000, -6.123233995736766085E-15 ) ) ;
#11458=CARTESIAN_POINT ( 'NONE',  ( -3.210462471511496205E-15, 23.35937500034139802, -52.43083105670540789 ) ) ;
#11462=ORIENTED_EDGE ( 'NONE', *, *, #15446, .T. ) ;
#11478=CARTESIAN_POINT ( 'NONE',  ( 49.86468353124999453, 46.95937500034139589, -16.20201782572376459 ) ) ;
#11479=ORIENTED_EDGE ( 'NONE', *, *, #13723, .T. ) ;
#11482=CARTESIAN_POINT ( 'NONE',  ( -30.81806926056962226, 32.15937500034139873, 42.41743335407647919 ) ) ;
#11486=DIRECTION ( 'NONE',  ( -0.000000000000000000, -1.000000000000000000, -0.000000000000000000 ) ) ;
#11488=CARTESIAN_POINT ( 'NONE',  ( 47.18644234407140203, 25.00000000000000711, -16.12223069495473737 ) ) ;
#11489=CARTESIAN_POINT ( 'NONE',  ( 40.34137639590981905, 36.72187500034139163, 29.30972558990010768 ) ) ;
#11499=CARTESIAN_POINT ( 'NONE',  ( 40.34137639590981905, 30.72187500034139518, 29.30972558990010768 ) ) ;
#11501=ORIENTED_EDGE ( 'NONE', *, *, #14515, .T. ) ;
#11503=CARTESIAN_POINT ( 'NONE',  ( -3.210462471511496205E-15, 33.35937500034139447, -52.43083105670540789 ) ) ;
#11504=ORIENTED_EDGE ( 'NONE', *, *, #15379, .F. ) ;
#11507=CARTESIAN_POINT ( 'NONE',  ( 49.86468353125000164, 48.85937500034139447, -6.106662507704105588E-15 ) ) ;
#11509=CARTESIAN_POINT ( 'NONE',  ( -49.86468353125000164, 25.92187500034139802, 0.000000000000000000 ) ) ;
#11515=CARTESIAN_POINT ( 'NONE',  ( 9.657523855033129090E-15, 48.50000000000000000, 52.57311121191334990 ) ) ;
#11525=CARTESIAN_POINT ( 'NONE',  ( -40.34137639590981905, 49.72187500034139873, -29.30972558990011478 ) ) ;
#11527=( LENGTH_UNIT ( ) NAMED_UNIT ( * ) SI_UNIT ( .MILLI., .METRE. ) );
#11528=AXIS2_PLACEMENT_3D ( 'NONE', #3973, #9215, #130 ) ;
#11532=CARTESIAN_POINT ( 'NONE',  ( 15.45084971874736723, 29.18125000068279817, -47.55282581475768211 ) ) ;
#11534=CARTESIAN_POINT ( 'NONE',  ( -49.86468353125000164, 47.92187500034139447, 0.000000000000000000 ) ) ;
#11542=CARTESIAN_POINT ( 'NONE',  ( -30.90169943749473447, 28.29999999999999716, 42.53254041760200721 ) ) ;
#11546=CARTESIAN_POINT ( 'NONE',  ( 40.45084971874737079, 26.98125000068279888, -29.38926261462366440 ) ) ;
#11553=CARTESIAN_POINT ( 'NONE',  ( 40.45084971874737789, 20.80000000000000426, 29.38926261462365375 ) ) ;
#11557=CARTESIAN_POINT ( 'NONE',  ( 49.86468353124999453, 38.95937500034139589, -16.20201782572376459 ) ) ;
#11561=CARTESIAN_POINT ( 'NONE',  ( 9.631387414534489405E-15, 30.35937500034139447, 52.43083105670540789 ) ) ;
#11567=CARTESIAN_POINT ( 'NONE',  ( 46.79661121261624146, 25.00000000000000711, -17.22183559214831661 ) ) ;
#11568=CARTESIAN_POINT ( 'NONE',  ( -15.40903463028481646, 31.52187500034139944, -47.42413220539093999 ) ) ;
#11569=EDGE_CURVE ( 'NONE', #6385, #1639, #7665, .T. ) ;
#11580=CARTESIAN_POINT ( 'NONE',  ( -49.86468353124999453, 29.82187500034139660, -16.20201782572375393 ) ) ;
#11585=STYLED_ITEM ( 'NONE', ( #8298 ), #1259 ) ;
#11586=CARTESIAN_POINT ( 'NONE',  ( -40.34137639590981905, 33.65937500034139873, -29.30972558990011478 ) ) ;
#11592=CARTESIAN_POINT ( 'NONE',  ( 15.40903463028482356, 48.45937500034140299, 47.42413220539093999 ) ) ;
#11596=CARTESIAN_POINT ( 'NONE',  ( 9.631387414534489405E-15, 24.42187500034139447, 52.43083105670540789 ) ) ;
#11602=CARTESIAN_POINT ( 'NONE',  ( -30.90169943749473802, 46.30000000000000426, 42.53254041760200721 ) ) ;
#11608=AXIS2_PLACEMENT_3D ( 'NONE', #11679, #15333, #11439 ) ;
#11611=ORIENTED_EDGE ( 'NONE', *, *, #13150, .F. ) ;
#11612=CARTESIAN_POINT ( 'NONE',  ( -30.90169943749473802, 36.08125000068280031, 42.53254041760200721 ) ) ;
#11617=CARTESIAN_POINT ( 'NONE',  ( -3.210462471511496205E-15, 45.42187500034138736, -52.43083105670540789 ) ) ;
#11619=DIRECTION ( 'NONE',  ( 0.000000000000000000, 0.000000000000000000, -1.000000000000000000 ) ) ;
#11620=CARTESIAN_POINT ( 'NONE',  ( -50.00000000000000000, 50.00000000000000000, 0.000000000000000000 ) ) ;
#11622=SHAPE_DEFINITION_REPRESENTATION ( #7990, #13496 ) ;
#11623=CARTESIAN_POINT ( 'NONE',  ( 50.00000000000000711, 34.68125000068279462, 16.24598481164530739 ) ) ;
#11628=CARTESIAN_POINT ( 'NONE',  ( 30.81806926056962936, 47.22187500034139873, -42.41743335407647209 ) ) ;
#11631=CARTESIAN_POINT ( 'NONE',  ( -49.99999999999999289, 25.89999999999999858, -16.24598481164531449 ) ) ;
#11633=ORIENTED_EDGE ( 'NONE', *, *, #1725, .T. ) ;
#11647=CARTESIAN_POINT ( 'NONE',  ( 30.90169943749475578, 20.69999999999999574, 42.53254041760200010 ) ) ;
#11649=CARTESIAN_POINT ( 'NONE',  ( -30.81806926056963292, 39.55937500034139731, -42.41743335407647209 ) ) ;
#11652=CARTESIAN_POINT ( 'NONE',  ( 30.81806926056962936, 29.15937500034139518, -42.41743335407647209 ) ) ;
#11654=LINE ( 'NONE', #7825, #6286 ) ;
#11657=CARTESIAN_POINT ( 'NONE',  ( -3.210462471511496205E-15, 33.42187500034139447, -52.43083105670540789 ) ) ;
#11667=CARTESIAN_POINT ( 'NONE',  ( 49.86468353125000164, 30.92187500034139802, -6.106662507704105588E-15 ) ) ;
#11669=CARTESIAN_POINT ( 'NONE',  ( -30.81806926056963292, 33.55937500034139020, -42.41743335407646498 ) ) ;
#11672=CARTESIAN_POINT ( 'NONE',  ( -40.34137639590981195, 48.05937500034139731, 29.30972558990012189 ) ) ;
#11679=CARTESIAN_POINT ( 'NONE',  ( 0.000000000000000000, 55.00000000000000711, 0.000000000000000000 ) ) ;
#11680=CARTESIAN_POINT ( 'NONE',  ( 15.45084971874737789, 38.60000000000000142, 47.55282581475767500 ) ) ;
#11687=CARTESIAN_POINT ( 'NONE',  ( 40.45084971874737789, 34.58125000068280031, 29.38926261462365375 ) ) ;
#11688=ORIENTED_EDGE ( 'NONE', *, *, #6754, .T. ) ;
#11704=CARTESIAN_POINT ( 'NONE',  ( -40.34137639590981195, 46.12187500034139731, 29.30972558990012189 ) ) ;
#11709=VECTOR ( 'NONE', #9654, 1000.000000000000000 ) ;
#11724=CARTESIAN_POINT ( 'NONE',  ( -15.40903463028481646, 35.45937500034139589, -47.42413220539093999 ) ) ;
#11727=CARTESIAN_POINT ( 'NONE',  ( -30.90169943749473802, 48.08125000068278609, 42.53254041760200721 ) ) ;
#11729=CARTESIAN_POINT ( 'NONE',  ( 15.40903463028482356, 20.45937500034139589, 47.42413220539093999 ) ) ;
#11734=CARTESIAN_POINT ( 'NONE',  ( 40.34137639590981905, 28.72187500034139873, 29.30972558990010768 ) ) ;
#11740=CARTESIAN_POINT ( 'NONE',  ( 50.00000000000000711, 36.89999999999999858, 16.24598481164530739 ) ) ;
#11746=CARTESIAN_POINT ( 'NONE',  ( 15.40903463028481113, 31.25937500034140015, -47.42413220539094709 ) ) ;
#11750=CARTESIAN_POINT ( 'NONE',  ( -15.40903463028480580, 40.25937500034139305, 47.42413220539094709 ) ) ;
#11757=CARTESIAN_POINT ( 'NONE',  ( 15.45084971874737789, 42.60000000000000142, 47.55282581475767500 ) ) ;
#11761=CARTESIAN_POINT ( 'NONE',  ( 49.86468353125001585, 44.82187500034138594, 16.20201782572375038 ) ) ;
#11763=CARTESIAN_POINT ( 'NONE',  ( -3.210462471511496205E-15, 49.35937500034138736, -52.43083105670540789 ) ) ;
#11764=VERTEX_POINT ( 'NONE', #1586 ) ;
#11765=CARTESIAN_POINT ( 'NONE',  ( -30.90169943749473802, 34.08125000068279320, 42.53254041760200721 ) ) ;
#11770=CARTESIAN_POINT ( 'NONE',  ( 30.81806926056964002, 48.62187500034139731, 42.41743335407646498 ) ) ;
#11774=DIRECTION ( 'NONE',  ( 0.000000000000000000, 0.000000000000000000, -1.000000000000000000 ) ) ;
#11780=CARTESIAN_POINT ( 'NONE',  ( -49.86468353124999453, 19.95937500034138878, 16.20201782572377525 ) ) ;
#11781=EDGE_LOOP ( 'NONE', ( #13466, #8629, #13827, #2643 ) ) ;
#11794=CARTESIAN_POINT ( 'NONE',  ( -49.99999999999999289, 33.68125000068278752, -16.24598481164531449 ) ) ;
#11804=CARTESIAN_POINT ( 'NONE',  ( 40.34137639590981905, 38.65937500034139873, 29.30972558990010768 ) ) ;
#11807=CARTESIAN_POINT ( 'NONE',  ( 15.45084971874736723, 49.18125000068279462, -47.55282581475768211 ) ) ;
#11809=CARTESIAN_POINT ( 'NONE',  ( -40.34137639590981905, 23.65937500034139518, -29.30972558990011478 ) ) ;
#11814=CARTESIAN_POINT ( 'NONE',  ( 9.631387414534489405E-15, 30.42187500034139447, 52.43083105670540789 ) ) ;
#11820=CARTESIAN_POINT ( 'NONE',  ( -49.99999999999999289, 36.10000000000000853, 16.24598481164533226 ) ) ;
#11824=ORIENTED_EDGE ( 'NONE', *, *, #5536, .T. ) ;
#11826=CARTESIAN_POINT ( 'NONE',  ( 9.631387414534489405E-15, 32.35937500034139447, 52.43083105670540789 ) ) ;
#11827=ORIENTED_EDGE ( 'NONE', *, *, #125, .T. ) ;
#11829=CARTESIAN_POINT ( 'NONE',  ( -49.86468353125000164, 41.85937500034139447, 0.000000000000000000 ) ) ;
#11838=CARTESIAN_POINT ( 'NONE',  ( -3.219174618344376363E-15, 41.49999999999999289, -52.57311121191334990 ) ) ;
#11843=CARTESIAN_POINT ( 'NONE',  ( 49.86468353124999453, 47.02187500034139589, -16.20201782572376459 ) ) ;
#11844=( GEOMETRIC_REPRESENTATION_CONTEXT ( 3 ) GLOBAL_UNCERTAINTY_ASSIGNED_CONTEXT ( ( #8253 ) ) GLOBAL_UNIT_ASSIGNED_CONTEXT ( ( #9805, #809, #11046 ) ) REPRESENTATION_CONTEXT ( 'NONE', 'WORKASPACE' ) );
#11853=CARTESIAN_POINT ( 'NONE',  ( -3.219174618344376363E-15, 33.28125000068280315, -52.57311121191334990 ) ) ;
#11857=CARTESIAN_POINT ( 'NONE',  ( 40.34137639590981195, 49.12187500034139731, -29.30972558990011834 ) ) ;
#11859=CARTESIAN_POINT ( 'NONE',  ( -30.90169943749473447, 40.08125000068279320, 42.53254041760200721 ) ) ;
#11867=CARTESIAN_POINT ( 'NONE',  ( 49.86468353125001585, 20.75937500034140015, 16.20201782572375038 ) ) ;
#11874=CARTESIAN_POINT ( 'NONE',  ( 0.000000000000000000, 252.1309828287255357, 0.000000000000000000 ) ) ;
#11875=AXIS2_PLACEMENT_3D ( 'NONE', #12360, #6974, #12114 ) ;
#11876=DIRECTION ( 'NONE',  ( 0.000000000000000000, 0.000000000000000000, -1.000000000000000000 ) ) ;
#11882=CARTESIAN_POINT ( 'NONE',  ( 50.00000000000000711, 48.90000000000000568, 16.24598481164530739 ) ) ;
#11889=ORIENTED_EDGE ( 'NONE', *, *, #5900, .F. ) ;
#11890=CARTESIAN_POINT ( 'NONE',  ( -3.210462471511496205E-15, 37.35937500034139447, -52.43083105670540789 ) ) ;
#11893=CARTESIAN_POINT ( 'NONE',  ( -40.45084971874737789, 49.58125000068280031, -29.38926261462365730 ) ) ;
#11895=CARTESIAN_POINT ( 'NONE',  ( -49.86468353124999453, 25.75937500034140015, -16.20201782572375393 ) ) ;
#11901=CARTESIAN_POINT ( 'NONE',  ( -30.81806926056963292, 29.62187500034139376, -42.41743335407646498 ) ) ;
#11909=CARTESIAN_POINT ( 'NONE',  ( 15.45084971874737789, 34.60000000000000853, 47.55282581475767500 ) ) ;
#11916=CARTESIAN_POINT ( 'NONE',  ( -3.210462471511496205E-15, 27.35937500034139447, -52.43083105670540789 ) ) ;
#11917=VERTEX_POINT ( 'NONE', #4578 ) ;
#11918=DIRECTION ( 'NONE',  ( 0.000000000000000000, 0.000000000000000000, -1.000000000000000000 ) ) ;
#11919=CARTESIAN_POINT ( 'NONE',  ( 15.40903463028481113, 41.25937500034139305, -47.42413220539094709 ) ) ;
#11925=CARTESIAN_POINT ( 'NONE',  ( -50.00000000000000000, 40.00000000000000000, 0.000000000000000000 ) ) ;
#11927=CARTESIAN_POINT ( 'NONE',  ( -49.86468353124999453, 41.82187500034140015, -16.20201782572375393 ) ) ;
#11930=EDGE_CURVE ( 'NONE', #5627, #12134, #10204, .T. ) ;
#11931=CARTESIAN_POINT ( 'NONE',  ( 49.86468353124999453, 46.95937500034139589, -16.20201782572376104 ) ) ;
#11933=CARTESIAN_POINT ( 'NONE',  ( -30.90169943749473802, 30.08125000068279675, 42.53254041760200721 ) ) ;
#11937=CARTESIAN_POINT ( 'NONE',  ( 15.40903463028481113, 43.32187500034139305, -47.42413220539094709 ) ) ;
#11939=CARTESIAN_POINT ( 'NONE',  ( -50.00000000000000000, 39.78125000068279604, 0.000000000000000000 ) ) ;
#11948=CARTESIAN_POINT ( 'NONE',  ( 15.40903463028481113, 43.32187500034139305, -47.42413220539094709 ) ) ;
#11958=FACE_OUTER_BOUND ( 'NONE', #10653, .T. ) ;
#11959=CARTESIAN_POINT ( 'NONE',  ( -49.99999999999999289, 45.90000000000000568, -16.24598481164531449 ) ) ;
#11965=CARTESIAN_POINT ( 'NONE',  ( 40.45084971874737079, 37.20000000000000284, -29.38926261462366440 ) ) ;
#11967=CARTESIAN_POINT ( 'NONE',  ( 49.86468353124999453, 30.95937500034139944, -16.20201782572376459 ) ) ;
#11970=ORIENTED_EDGE ( 'NONE', *, *, #320, .F. ) ;
#11973=CARTESIAN_POINT ( 'NONE',  ( -3.210462471511496205E-15, 23.35937500034139802, -52.43083105670540789 ) ) ;
#11979=CARTESIAN_POINT ( 'NONE',  ( -49.86468353125000164, 29.92187500034139802, 0.000000000000000000 ) ) ;
#11985=CARTESIAN_POINT ( 'NONE',  ( -15.45084971874737256, 37.60000000000000142, -47.55282581475767500 ) ) ;
#11987=CARTESIAN_POINT ( 'NONE',  ( 0.000000000000000000, 193.4213562373095385, 0.000000000000000000 ) ) ;
#11990=CARTESIAN_POINT ( 'NONE',  ( 40.34137639590981905, 30.65937500034139518, 29.30972558990010768 ) ) ;
#11994=CARTESIAN_POINT ( 'NONE',  ( -40.34137639590981905, 43.65937500034139163, -29.30972558990011478 ) ) ;
#11996=EDGE_CURVE ( 'NONE', #15793, #5080, #15034, .T. ) ;
#12002=CARTESIAN_POINT ( 'NONE',  ( -30.81806926056963292, 27.62187500034139731, -42.41743335407647209 ) ) ;
#12003=CARTESIAN_POINT ( 'NONE',  ( -30.90169943749473802, 40.30000000000000426, 42.53254041760200721 ) ) ;
#12006=CARTESIAN_POINT ( 'NONE',  ( 9.631387414534489405E-15, 44.42187500034140157, 52.43083105670540789 ) ) ;
#12009=CARTESIAN_POINT ( 'NONE',  ( -49.86468353125000164, 45.85937500034140157, 0.000000000000000000 ) ) ;
#12011=CARTESIAN_POINT ( 'NONE',  ( 9.657523855033129090E-15, 28.28125000068279249, 52.57311121191334990 ) ) ;
#12013=CARTESIAN_POINT ( 'NONE',  ( -30.90169943749474513, 49.48125000068279178, -42.53254041760200721 ) ) ;
#12015=CARTESIAN_POINT ( 'NONE',  ( -15.40903463028481646, 43.52187500034139589, -47.42413220539093999 ) ) ;
#12024=CARTESIAN_POINT ( 'NONE',  ( -30.81806926056962226, 40.22187500034139873, 42.41743335407647919 ) ) ;
#12042=CARTESIAN_POINT ( 'NONE',  ( -49.86468353124999453, 33.95937500034139589, 16.20201782572377525 ) ) ;
#12045=ORIENTED_EDGE ( 'NONE', *, *, #12429, .F. ) ;
#12048=CARTESIAN_POINT ( 'NONE',  ( 50.00000000000000711, 44.68125000068278752, 16.24598481164530739 ) ) ;
#12050=CARTESIAN_POINT ( 'NONE',  ( 40.34137639590981195, 23.05937500034139731, -29.30972558990011834 ) ) ;
#12055=CARTESIAN_POINT ( 'NONE',  ( -49.86468353125000164, 27.92187500034139447, 0.000000000000000000 ) ) ;
#12057=( BOUNDED_CURVE ( )  B_SPLINE_CURVE ( 2, ( #11019, #4884, #8594, #8354, #9940, #9688, #7287, #16087, #3628, #11114, #10935, #4722, #9783 ),
 .UNSPECIFIED., .F., .T. ) 
 B_SPLINE_CURVE_WITH_KNOTS ( ( 3, 2, 2, 2, 2, 2, 3 ),
 ( 0.4500000000000000111, 0.4533333333333333104, 0.4600000000000000200, 0.4666666666666666741, 0.4733333333333333282, 0.4799999999999999822, 0.4833333333333333370 ),
 .UNSPECIFIED. ) 
 CURVE ( )  GEOMETRIC_REPRESENTATION_ITEM ( )  RATIONAL_B_SPLINE_CURVE ( ( 0.9755282581475768211, 0.9755282581475770431, 1.000000000000000000, 0.9510565162951535312, 1.000000000000000000, 0.9510565162951535312, 1.000000000000000000, 0.9510565162951535312, 1.000000000000000000, 0.9510565162951535312, 1.000000000000000000, 0.9755282581475768211, 0.9755282581475768211 ) ) 
 REPRESENTATION_ITEM ( '' )  );
#12063=CARTESIAN_POINT ( 'NONE',  ( -49.99999999999999289, 31.89999999999999858, -16.24598481164531449 ) ) ;
#12068=CARTESIAN_POINT ( 'NONE',  ( 30.81806926056964002, 28.55937500034139376, 42.41743335407646498 ) ) ;
#12070=FACE_OUTER_BOUND ( 'NONE', #9661, .T. ) ;
#12071=CARTESIAN_POINT ( 'NONE',  ( 9.631387414534489405E-15, 44.35937500034140157, 52.43083105670540789 ) ) ;
#12073=CARTESIAN_POINT ( 'NONE',  ( 50.00000000000000000, 44.78125000068280315, -6.123233995736766085E-15 ) ) ;
#12077=CARTESIAN_POINT ( 'NONE',  ( -49.86468353124999453, 28.02187500034139234, 16.20201782572377525 ) ) ;
#12081=CARTESIAN_POINT ( 'NONE',  ( -30.81806926056963292, 45.62187500034139020, -42.41743335407647209 ) ) ;
#12088=CARTESIAN_POINT ( 'NONE',  ( 40.34137639590981905, 48.65937500034139873, 29.30972558990010768 ) ) ;
#12091=CARTESIAN_POINT ( 'NONE',  ( -15.45084971874737256, 33.38125000068280457, -47.55282581475767500 ) ) ;
#12096=CARTESIAN_POINT ( 'NONE',  ( -40.34137639590981905, 43.72187500034139873, -29.30972558990011478 ) ) ;
#12099=CARTESIAN_POINT ( 'NONE',  ( 1.293669679204937499E-13, 39.28125000068280315, -50.00000000000000000 ) ) ;
#12107=EDGE_LOOP ( 'NONE', ( #14125, #2566, #10135, #6237 ) ) ;
#12109=CARTESIAN_POINT ( 'NONE',  ( 15.40903463028481113, 45.32187500034140015, -47.42413220539094709 ) ) ;
#12114=DIRECTION ( 'NONE',  ( 0.000000000000000000, 0.000000000000000000, 1.000000000000000000 ) ) ;
#12123=CARTESIAN_POINT ( 'NONE',  ( -7.919222016226816763, 29.55125428154684286, -49.99999999999999289 ) ) ;
#12129=CARTESIAN_POINT ( 'NONE',  ( 7.919222016226875382, 37.44874571845315359, -49.99999999999997158 ) ) ;
#12131=CARTESIAN_POINT ( 'NONE',  ( -15.40903463028480580, 28.25937500034139660, 47.42413220539094709 ) ) ;
#12132=AXIS2_PLACEMENT_3D ( 'NONE', #12726, #1077, #11242 ) ;
#12134=VERTEX_POINT ( 'NONE', #6402 ) ;
#12136=ADVANCED_FACE ( 'NONE', ( #59 ), #5164, .T. ) ;
#12137=AXIS2_PLACEMENT_3D ( 'NONE', #3053, #4395, #14516 ) ;
#12138=CARTESIAN_POINT ( 'NONE',  ( 50.00000000000000000, 44.78125000068280315, -6.123233995736766085E-15 ) ) ;
#12139=CARTESIAN_POINT ( 'NONE',  ( 7.919222016226807881, 46.55125428154685352, 50.00000000000000000 ) ) ;
#12149=CARTESIAN_POINT ( 'NONE',  ( 7.919222016226758143, 36.33250428222963535, 50.00000000000000711 ) ) ;
#12150=CARTESIAN_POINT ( 'NONE',  ( -40.45084971874737079, 42.20000000000000284, 29.38926261462367151 ) ) ;
#12153=CARTESIAN_POINT ( 'NONE',  ( -15.45084971874737256, 29.60000000000000142, -47.55282581475767500 ) ) ;
#12161=CARTESIAN_POINT ( 'NONE',  ( -49.86468353124999453, 37.95937500034140299, 16.20201782572377525 ) ) ;
#12164=CARTESIAN_POINT ( 'NONE',  ( 8.446640517145639571E-15, 48.49999999999999289, 50.00000000000000000 ) ) ;
#12169=CARTESIAN_POINT ( 'NONE',  ( 49.86468353125001585, 32.82187500034139305, 16.20201782572375038 ) ) ;
#12170=CARTESIAN_POINT ( 'NONE',  ( 15.45084971874736723, 33.39999999999999858, -47.55282581475768211 ) ) ;
#12173=CARTESIAN_POINT ( 'NONE',  ( 40.34137639590981905, 38.72187500034139873, 29.30972558990010768 ) ) ;
#12177=CARTESIAN_POINT ( 'NONE',  ( -49.86468353124999453, 39.95937500034139589, 16.20201782572377169 ) ) ;
#12179=CARTESIAN_POINT ( 'NONE',  ( 15.45084971874737789, 32.38125000068280457, 47.55282581475767500 ) ) ;
#12181=ORIENTED_EDGE ( 'NONE', *, *, #14234, .T. ) ;
#12183=CARTESIAN_POINT ( 'NONE',  ( -15.40903463028481646, 41.52187500034139589, -47.42413220539093999 ) ) ;
#12186=CARTESIAN_POINT ( 'NONE',  ( -3.210462471511496205E-15, 23.42187500034139802, -52.43083105670540789 ) ) ;
#12193=CARTESIAN_POINT ( 'NONE',  ( -40.34137639590981905, 41.72187500034139873, -29.30972558990011478 ) ) ;
#12194=ORIENTED_EDGE ( 'NONE', *, *, #13332, .F. ) ;
#12205=CARTESIAN_POINT ( 'NONE',  ( -3.111920190527341144E-15, 25.50000000000000355, -50.00000000000000000 ) ) ;
#12206=EDGE_CURVE ( 'NONE', #1863, #13641, #12962, .T. ) ;
#12215=CARTESIAN_POINT ( 'NONE',  ( -3.210462471511496205E-15, 31.35937500034139092, -52.43083105670540789 ) ) ;
#12219=CARTESIAN_POINT ( 'NONE',  ( 50.00000000000000711, 46.68125000068278752, 16.24598481164530739 ) ) ;
#12228=CARTESIAN_POINT ( 'NONE',  ( 45.11452830843730766, 25.00000000000000355, -21.24066852005663719 ) ) ;
#12229=CARTESIAN_POINT ( 'NONE',  ( 0.000000000000000000, 272.0000000000000000, -82.49773270518484480 ) ) ;
#12230=CARTESIAN_POINT ( 'NONE',  ( -7.919222016226773242, 42.44874571845315359, 50.00000000000000711 ) ) ;
#12234=CARTESIAN_POINT ( 'NONE',  ( -15.45084971874736368, 26.40000000000000213, 47.55282581475768211 ) ) ;
#12237=CARTESIAN_POINT ( 'NONE',  ( -15.40903463028480580, 48.25937500034140015, 47.42413220539094709 ) ) ;
#12239=CARTESIAN_POINT ( 'NONE',  ( -15.40903463028481646, 25.45937500034139589, -47.42413220539093999 ) ) ;
#12240=EDGE_LOOP ( 'NONE', ( #7258, #268, #6440, #9343 ) ) ;
#12242=CARTESIAN_POINT ( 'NONE',  ( -3.210462471511496205E-15, 33.35937500034140157, -52.43083105670540789 ) ) ;
#12249=CARTESIAN_POINT ( 'NONE',  ( -3.210462471511496205E-15, 27.42187500034139092, -52.43083105670540789 ) ) ;
#12252=CARTESIAN_POINT ( 'NONE',  ( 15.40903463028482356, 38.52187500034139589, 47.42413220539093999 ) ) ;
#12257=CARTESIAN_POINT ( 'NONE',  ( -15.40903463028481646, 39.45937500034139589, -47.42413220539093999 ) ) ;
#12259=CARTESIAN_POINT ( 'NONE',  ( -30.90169943749473802, 24.08125000068279675, 42.53254041760200721 ) ) ;
#12262=CARTESIAN_POINT ( 'NONE',  ( -49.86468353124999453, 42.02187500034139589, 16.20201782572377169 ) ) ;
#12265=CARTESIAN_POINT ( 'NONE',  ( 40.34137639590981195, 25.12187500034139376, -29.30972558990011834 ) ) ;
#12270=CARTESIAN_POINT ( 'NONE',  ( 49.86468353124999453, 45.02187500034138878, -16.20201782572376459 ) ) ;
#12271=CARTESIAN_POINT ( 'NONE',  ( -30.90169943749474513, 43.48125000068279178, -42.53254041760200721 ) ) ;
#12272=ORIENTED_EDGE ( 'NONE', *, *, #9667, .F. ) ;
#12278=CARTESIAN_POINT ( 'NONE',  ( -15.45084971874737256, 49.60000000000000853, -47.55282581475767500 ) ) ;
#12282=CARTESIAN_POINT ( 'NONE',  ( -30.90169943749473447, 30.29999999999999716, 42.53254041760200721 ) ) ;
#12289=CARTESIAN_POINT ( 'NONE',  ( -49.86468353124999453, 31.95937500034139944, 16.20201782572377525 ) ) ;
#12295=CARTESIAN_POINT ( 'NONE',  ( -50.00000000000000000, 43.78125000068280315, 0.000000000000000000 ) ) ;
#12305=CARTESIAN_POINT ( 'NONE',  ( 0.000000000000000000, 193.4213562373095385, 0.000000000000000000 ) ) ;
#12307=CARTESIAN_POINT ( 'NONE',  ( -30.90169943749473447, 42.30000000000000426, 42.53254041760200721 ) ) ;
#12310=EDGE_CURVE ( 'NONE', #326, #5251, #8425, .T. ) ;
#12311=CARTESIAN_POINT ( 'NONE',  ( 15.45084971874737789, 28.60000000000000142, 47.55282581475767500 ) ) ;
#12313=CARTESIAN_POINT ( 'NONE',  ( -15.45084971874736368, 44.39999999999999858, 47.55282581475768211 ) ) ;
#12320=CARTESIAN_POINT ( 'NONE',  ( -15.40903463028481646, 35.45937500034139589, -47.42413220539093999 ) ) ;
#12329=CARTESIAN_POINT ( 'NONE',  ( -15.40903463028480580, 32.32187500034139305, 47.42413220539094709 ) ) ;
#12331=CARTESIAN_POINT ( 'NONE',  ( 30.90169943749475223, 32.70000000000000284, 42.53254041760199300 ) ) ;
#12333=CARTESIAN_POINT ( 'NONE',  ( -49.86468353125000164, 39.92187500034139447, 0.000000000000000000 ) ) ;
#12334=( BOUNDED_CURVE ( )  B_SPLINE_CURVE ( 2, ( #2141, #5820, #2389, #9965, #11382 ),
 .UNSPECIFIED., .F., .F. ) 
 B_SPLINE_CURVE_WITH_KNOTS ( ( 3, 2, 3 ),
 ( 0.8166666666666666519, 0.8199999999999999512, 0.8260183939300572709 ),
 .UNSPECIFIED. ) 
 CURVE ( )  GEOMETRIC_REPRESENTATION_ITEM ( )  RATIONAL_B_SPLINE_CURVE ( ( 0.9755282581475768211, 0.9755282581475768211, 1.000000000000000000, 0.9558158252132341604, 0.9914069812288468508 ) ) 
 REPRESENTATION_ITEM ( '' )  );
#12336=AXIS2_PLACEMENT_3D ( 'NONE', #3130, #6807, #2963 ) ;
#12339=CARTESIAN_POINT ( 'NONE',  ( 49.86468353125000164, 40.85937500034139447, -6.106662507704105588E-15 ) ) ;
#12341=CARTESIAN_POINT ( 'NONE',  ( -40.45084971874737789, 23.58125000068280031, -29.38926261462365730 ) ) ;
#12342=ORIENTED_EDGE ( 'NONE', *, *, #12648, .F. ) ;
#12344=CARTESIAN_POINT ( 'NONE',  ( 49.86468353124999453, 33.02187500034139589, -16.20201782572376104 ) ) ;
#12348=CARTESIAN_POINT ( 'NONE',  ( -49.86468353124999453, 25.82187500034139305, -16.20201782572375393 ) ) ;
#12352=VERTEX_POINT ( 'NONE', #1807 ) ;
#12353=CARTESIAN_POINT ( 'NONE',  ( 40.34137639590981905, 36.72187500034139163, 29.30972558990010768 ) ) ;
#12355=ORIENTED_EDGE ( 'NONE', *, *, #10, .T. ) ;
#12360=CARTESIAN_POINT ( 'NONE',  ( 0.000000000000000000, 25.00000000000000000, 0.000000000000000000 ) ) ;
#12370=CLOSED_SHELL ( 'NONE', ( #6843, #13924, #14241, #6326, #15892, #5552, #15815, #5444, #4734, #9524, #1142, #2547, #4836, #6376, #12514, #12136, #13671, #1024, #1916, #723, #3997, #10836, #8422, #11176, #3793, #5323, #15167, #9896, #7638, #13011, #7720, #4895, #3371, #15249, #5423, #15789, #8760, #4471, #2886, #8329, #7123, #13666, #8859, #6559, #7204, #13048, #1632, #15243, #8794, #7230 ) ) ;
#12371=SURFACE_STYLE_USAGE ( .BOTH. , #13287 ) ;
#12374=CARTESIAN_POINT ( 'NONE',  ( 0.000000000000000000, 272.0000000000000000, 0.000000000000000000 ) ) ;
#12376=CARTESIAN_POINT ( 'NONE',  ( -50.00000000000000000, 34.00000000000000000, 0.000000000000000000 ) ) ;
#12379=COLOUR_RGB ( '', 0.09019608, 0.27058824, 0.51372549) ;
#12380=ORIENTED_EDGE ( 'NONE', *, *, #2982, .F. ) ;
#12381=CARTESIAN_POINT ( 'NONE',  ( -49.86468353124999453, 21.95937500034138878, 16.20201782572377525 ) ) ;
#12383=ORIENTED_EDGE ( 'NONE', *, *, #1806, .T. ) ;
#12386=CARTESIAN_POINT ( 'NONE',  ( 40.45084971874737789, 40.58125000068280031, 29.38926261462365375 ) ) ;
#12391=CARTESIAN_POINT ( 'NONE',  ( 15.45084971874737789, 46.60000000000000142, 47.55282581475767500 ) ) ;
#12399=CARTESIAN_POINT ( 'NONE',  ( 43.39327851764676325, 25.00000000000000355, -25.00490296284272773 ) ) ;
#12400=DIRECTION ( 'NONE',  ( 0.000000000000000000, 0.000000000000000000, -1.000000000000000000 ) ) ;
#12402=CARTESIAN_POINT ( 'NONE',  ( -15.45084971874736368, 42.39999999999999858, 47.55282581475768211 ) ) ;
#12406=CARTESIAN_POINT ( 'NONE',  ( 40.45084971874737789, 26.80000000000000071, 29.38926261462365375 ) ) ;
#12410=CARTESIAN_POINT ( 'NONE',  ( -15.40903463028480580, 46.25937500034140015, 47.42413220539094709 ) ) ;
#12412=CARTESIAN_POINT ( 'NONE',  ( 15.40903463028481113, 25.25937500034139660, -47.42413220539094709 ) ) ;
#12413=ORIENTED_EDGE ( 'NONE', *, *, #12648, .T. ) ;
#12415=CARTESIAN_POINT ( 'NONE',  ( 30.81806926056964002, 32.55937500034139731, 42.41743335407647209 ) ) ;
#12421=CARTESIAN_POINT ( 'NONE',  ( 30.90169943749473802, 45.08125000068280031, -42.53254041760200721 ) ) ;
#12426=CARTESIAN_POINT ( 'NONE',  ( 30.90169943749473802, 33.30000000000000426, -42.53254041760200721 ) ) ;
#12428=CARTESIAN_POINT ( 'NONE',  ( -15.40903463028480580, 40.32187500034140015, 47.42413220539094709 ) ) ;
#12429=EDGE_CURVE ( 'NONE', #5870, #6547, #710, .T. ) ;
#12431=ORIENTED_EDGE ( 'NONE', *, *, #7014, .T. ) ;
#12432=CARTESIAN_POINT ( 'NONE',  ( -3.210462471511496205E-15, 45.35937500034139447, -52.43083105670540789 ) ) ;
#12434=CARTESIAN_POINT ( 'NONE',  ( -49.99999999999999289, 21.68125000068280173, -16.24598481164531449 ) ) ;
#12439=( BOUNDED_CURVE ( )  B_SPLINE_CURVE ( 2, ( #15833, #15918, #4461, #14489, #9527, #11763, #7032, #1787, #9439, #13017, #9603, #8271, #12088, #692, #5785, #10852, #363, #4372, #4540, #14651, #1619, #8101, #6713, #3122, #6878, #5465, #531, #10531, #9282, #11931, #5626, #10688, #14336, #2953, #8020, #15744, #8193, #13260, #1860, #6955, #12009, #14990, #8681, #11014, #4620, #12432, #16169, #11192, #2361, #13579, #4878, #13499, #13413, #14906, #5952, #7367, #7445, #16079, #6037, #938, #11110, #2185, #4714, #8514, #9776, #11269, #6196, #8588, #7280, #859, #3534, #13748, #9935, #5869, #12510, #3366, #3453, #14823, #2107, #777, #1025, #16245, #2026, #4801, #1102, #7119, #9854, #13661, #6120, #2272, #12339, #3619, #16327, #7194, #4964, #9684, #10023, #3280, #8350, #12177, #10931, #15994, #14734, #8436, #12257, #2521, #267, #9093, #16416, #10181, #6616, #2609, #15154, #10342, #9015, #15076, #14150, #15232, #5050, #7761, #7685, #8842, #13825, #2768, #7843, #14072, #12920, #8763, #13903, #5372, #1526, #3705, #7601, #2686, #11351, #6444, #12832, #1436, #8929, #15406, #1351, #6365, #101, #12676, #10102, #3780, #5128, #1274, #2437, #11429, #7515, #12586, #5204, #1183, #6281, #3860, #6525, #22, #10263, #13990, #5293, #4023, #11586, #11669, #12755, #11503, #15321, #3943, #187, #3101, #14237, #5609, #4276, #4199, #6697, #11826, #9420, #9509, #4105, #5681, #10750, #8176, #15810, #4442, #14557, #1683, #11746, #13243, #6866, #1842, #3181, #9342, #11990, #9263, #9176, #10673, #13079, #14466, #8254, #6781, #13157, #13318, #1768, #14393, #435, #15653, #5537, #1919, #7012, #15726, #3014, #8004, #4356, #12068, #588, #13000, #669, #10510, #10598, #8084, #14318, #10427, #6938, #15482, #2858, #11916, #7926, #1604, #514, #348, #5447, #15573, #2938, #8416, #13482, #9662, #7422, #7101, #13727, #2089, #16057, #2341, #7177, #4689, #12239, #5933, #12412, #8569, #10996, #15976, #4524 ),
 .UNSPECIFIED., .F., .F. ) 
 B_SPLINE_CURVE_WITH_KNOTS ( ( 3, 2, 2, 2, 2, 2, 2, 2, 2, 2, 2, 2, 2, 2, 2, 2, 2, 2, 2, 2, 2, 2, 2, 2, 2, 2, 2, 2, 2, 2, 2, 2, 2, 2, 2, 2, 2, 2, 2, 2, 2, 2, 2, 2, 2, 2, 2, 2, 2, 2, 2, 2, 2, 2, 2, 2, 2, 2, 2, 2, 2, 2, 2, 2, 2, 2, 2, 2, 2, 2, 2, 2, 2, 2, 2, 2, 2, 2, 2, 2, 2, 2, 2, 2, 2, 2, 2, 2, 2, 2, 2, 2, 2, 2, 2, 2, 2, 2, 2, 2, 2, 2, 2, 2, 2, 2, 2, 2, 2, 2, 2, 2, 2, 2, 2, 2, 2, 2, 2, 2, 2, 2, 2, 2, 2, 3 ),
 ( 0.000000000000000000, 0.006666666666666667095, 0.01333333333333333419, 0.02000000000000000042, 0.02666666666666666838, 0.03333333333333333287, 0.04000000000000000083, 0.04666666666666666879, 0.05333333333333333676, 0.05999999999999999778, 0.06666666666666666574, 0.07333333333333333370, 0.08000000000000000167, 0.08666666666666666963, 0.09333333333333333759, 0.1000000000000000056, 0.1066666666666666735, 0.1133333333333333276, 0.1199999999999999956, 0.1266666666666666774, 0.1333333333333333315, 0.1400000000000000133, 0.1466666666666666674, 0.1533333333333333215, 0.1600000000000000033, 0.1666666666666666574, 0.1733333333333333393, 0.1799999999999999933, 0.1866666666666666752, 0.1933333333333333293, 0.2000000000000000111, 0.2066666666666666652, 0.2133333333333333470, 0.2200000000000000011, 0.2266666666666666552, 0.2333333333333333370, 0.2399999999999999911, 0.2466666666666666730, 0.2533333333333333548, 0.2600000000000000089, 0.2666666666666666630, 0.2733333333333333171, 0.2800000000000000266, 0.2866666666666666807, 0.2933333333333333348, 0.2999999999999999889, 0.3066666666666666430, 0.3133333333333333526, 0.3200000000000000067, 0.3266666666666666607, 0.3333333333333333148, 0.3400000000000000244, 0.3466666666666666785, 0.3533333333333333326, 0.3599999999999999867, 0.3666666666666666408, 0.3733333333333333504, 0.3800000000000000044, 0.3866666666666666585, 0.3933333333333333126, 0.4000000000000000222, 0.4066666666666666763, 0.4133333333333333304, 0.4199999999999999845, 0.4266666666666666941, 0.4333333333333333481, 0.4400000000000000022, 0.4466666666666666563, 0.4533333333333333104, 0.4600000000000000200, 0.4666666666666666741, 0.4733333333333333282, 0.4799999999999999822, 0.4866666666666666918, 0.4933333333333333459, 0.5000000000000000000, 0.5066666666666667096, 0.5133333333333333082, 0.5200000000000000178, 0.5266666666666666163, 0.5333333333333333259, 0.5400000000000000355, 0.5466666666666666341, 0.5533333333333333437, 0.5600000000000000533, 0.5666666666666666519, 0.5733333333333333615, 0.5799999999999999600, 0.5866666666666666696, 0.5933333333333333792, 0.5999999999999999778, 0.6066666666666665764, 0.6133333333333332860, 0.6200000000000001066, 0.6266666666666667052, 0.6333333333333334147, 0.6400000000000000133, 0.6466666666666667229, 0.6533333333333333215, 0.6599999999999999201, 0.6666666666666666297, 0.6733333333333332282, 0.6800000000000000488, 0.6866666666666667584, 0.6933333333333333570, 0.7000000000000000666, 0.7066666666666666652, 0.7133333333333332638, 0.7199999999999999734, 0.7266666666666665719, 0.7333333333333332815, 0.7400000000000001021, 0.7466666666666667007, 0.7533333333333334103, 0.7600000000000000089, 0.7666666666666666075, 0.7733333333333333171, 0.7799999999999999156, 0.7866666666666666252, 0.7933333333333332238, 0.8000000000000000444, 0.8066666666666667540, 0.8133333333333333526, 0.8200000000000000622, 0.8266666666666666607, 0.8286737259468953676 ),
 .UNSPECIFIED. ) 
 CURVE ( )  GEOMETRIC_REPRESENTATION_ITEM ( )  RATIONAL_B_SPLINE_CURVE ( ( 1.000000000000000000, 0.9510565162951535312, 1.000000000000000000, 0.9510565162951535312, 1.000000000000000000, 0.9510565162951535312, 1.000000000000000000, 0.9510565162951535312, 1.000000000000000000, 0.9510565162951535312, 1.000000000000000000, 0.9510565162951535312, 1.000000000000000000, 0.9510565162951535312, 1.000000000000000000, 0.9510565162951535312, 1.000000000000000000, 0.9510565162951535312, 1.000000000000000000, 0.9510565162951535312, 1.000000000000000000, 0.9510565162951535312, 1.000000000000000000, 0.9510565162951535312, 1.000000000000000000, 0.9510565162951535312, 1.000000000000000000, 0.9510565162951535312, 1.000000000000000000, 0.9510565162951535312, 1.000000000000000000, 0.9510565162951535312, 1.000000000000000000, 0.9510565162951535312, 1.000000000000000000, 0.9510565162951535312, 1.000000000000000000, 0.9510565162951535312, 1.000000000000000000, 0.9510565162951535312, 1.000000000000000000, 0.9510565162951535312, 1.000000000000000000, 0.9510565162951535312, 1.000000000000000000, 0.9510565162951535312, 1.000000000000000000, 0.9510565162951535312, 1.000000000000000000, 0.9510565162951535312, 1.000000000000000000, 0.9510565162951535312, 1.000000000000000000, 0.9510565162951535312, 1.000000000000000000, 0.9510565162951535312, 1.000000000000000000, 0.9510565162951535312, 1.000000000000000000, 0.9510565162951535312, 1.000000000000000000, 0.9510565162951535312, 1.000000000000000000, 0.9510565162951535312, 1.000000000000000000, 0.9510565162951535312, 1.000000000000000000, 0.9510565162951535312, 1.000000000000000000, 0.9510565162951535312, 1.000000000000000000, 0.9510565162951535312, 1.000000000000000000, 0.9510565162951535312, 1.000000000000000000, 0.9510565162951535312, 1.000000000000000000, 0.9510565162951535312, 1.000000000000000000, 0.9510565162951535312, 1.000000000000000000, 0.9510565162951535312, 1.000000000000000000, 0.9510565162951535312, 1.000000000000000000, 0.9510565162951535312, 1.000000000000000000, 0.9510565162951535312, 1.000000000000000000, 0.9510565162951535312, 1.000000000000000000, 0.9510565162951535312, 1.000000000000000000, 0.9510565162951535312, 1.000000000000000000, 0.9510565162951535312, 1.000000000000000000, 0.9510565162951535312, 1.000000000000000000, 0.9510565162951535312, 1.000000000000000000, 0.9510565162951535312, 1.000000000000000000, 0.9510565162951535312, 1.000000000000000000, 0.9510565162951535312, 1.000000000000000000, 0.9510565162951535312, 1.000000000000000000, 0.9510565162951535312, 1.000000000000000000, 0.9510565162951535312, 1.000000000000000000, 0.9510565162951535312, 1.000000000000000000, 0.9510565162951535312, 1.000000000000000000, 0.9510565162951535312, 1.000000000000000000, 0.9510565162951535312, 1.000000000000000000, 0.9510565162951535312, 1.000000000000000000, 0.9510565162951535312, 1.000000000000000000, 0.9510565162951535312, 1.000000000000000000, 0.9510565162951535312, 1.000000000000000000, 0.9510565162951535312, 1.000000000000000000, 0.9510565162951535312, 1.000000000000000000, 0.9510565162951535312, 1.000000000000000000, 0.9510565162951535312, 1.000000000000000000, 0.9510565162951535312, 1.000000000000000000, 0.9510565162951535312, 1.000000000000000000, 0.9510565162951535312, 1.000000000000000000, 0.9510565162951535312, 1.000000000000000000, 0.9510565162951535312, 1.000000000000000000, 0.9510565162951535312, 1.000000000000000000, 0.9510565162951535312, 1.000000000000000000, 0.9510565162951535312, 1.000000000000000000, 0.9510565162951535312, 1.000000000000000000, 0.9510565162951535312, 1.000000000000000000, 0.9510565162951535312, 1.000000000000000000, 0.9510565162951535312, 1.000000000000000000, 0.9510565162951535312, 1.000000000000000000, 0.9510565162951535312, 1.000000000000000000, 0.9510565162951535312, 1.000000000000000000, 0.9510565162951535312, 1.000000000000000000, 0.9510565162951535312, 1.000000000000000000, 0.9510565162951535312, 1.000000000000000000, 0.9510565162951535312, 1.000000000000000000, 0.9510565162951535312, 1.000000000000000000, 0.9510565162951535312, 1.000000000000000000, 0.9510565162951535312, 1.000000000000000000, 0.9510565162951535312, 1.000000000000000000, 0.9510565162951535312, 1.000000000000000000, 0.9510565162951535312, 1.000000000000000000, 0.9510565162951535312, 1.000000000000000000, 0.9510565162951535312, 1.000000000000000000, 0.9510565162951535312, 1.000000000000000000, 0.9510565162951535312, 1.000000000000000000, 0.9510565162951535312, 1.000000000000000000, 0.9510565162951535312, 1.000000000000000000, 0.9510565162951535312, 1.000000000000000000, 0.9510565162951535312, 1.000000000000000000, 0.9510565162951535312, 1.000000000000000000, 0.9510565162951535312, 1.000000000000000000, 0.9510565162951535312, 1.000000000000000000, 0.9510565162951535312, 1.000000000000000000, 0.9510565162951535312, 1.000000000000000000, 0.9510565162951535312, 1.000000000000000000, 0.9510565162951535312, 1.000000000000000000, 0.9510565162951535312, 1.000000000000000000, 0.9510565162951535312, 1.000000000000000000, 0.9510565162951535312, 1.000000000000000000, 0.9510565162951535312, 1.000000000000000000, 0.9510565162951535312, 1.000000000000000000, 0.9510565162951535312, 1.000000000000000000, 0.9510565162951535312, 1.000000000000000000, 0.9510565162951535312, 1.000000000000000000, 0.9510565162951535312, 1.000000000000000000, 0.9510565162951535312, 1.000000000000000000, 0.9510565162951535312, 1.000000000000000000, 0.9510565162951535312, 1.000000000000000000, 0.9510565162951535312, 1.000000000000000000, 0.9510565162951535312, 1.000000000000000000, 0.9510565162951535312, 1.000000000000000000, 0.9510565162951535312, 1.000000000000000000, 0.9852651290235199255, 0.9794023859079349359 ) ) 
 REPRESENTATION_ITEM ( '' )  );
#12440=CARTESIAN_POINT ( 'NONE',  ( -40.34137639590981905, 21.72187500034139518, -29.30972558990011478 ) ) ;
#12446=CARTESIAN_POINT ( 'NONE',  ( 49.86468353125000164, 36.92187500034140157, -6.106662507704105588E-15 ) ) ;
#12449=ORIENTED_EDGE ( 'NONE', *, *, #10633, .F. ) ;
#12453=CARTESIAN_POINT ( 'NONE',  ( -6.668400408272873429E-15, 49.50000000000000000, -50.00000000000000000 ) ) ;
#12461=EDGE_CURVE ( 'NONE', #495, #2810, #16191, .T. ) ;
#12463=CARTESIAN_POINT ( 'NONE',  ( -30.90169943749473447, 34.29999999999999005, 42.53254041760200721 ) ) ;
#12467=CARTESIAN_POINT ( 'NONE',  ( -40.34137639590981195, 24.05937500034139731, 29.30972558990012189 ) ) ;
#12471=CARTESIAN_POINT ( 'NONE',  ( -30.90169943749473802, 40.08125000068279320, 42.53254041760200721 ) ) ;
#12483=CARTESIAN_POINT ( 'NONE',  ( 30.90169943749473802, 49.29999999999999716, -42.53254041760200721 ) ) ;
#12486=CARTESIAN_POINT ( 'NONE',  ( -3.219174618344376363E-15, 31.50000000000000000, -52.57311121191334990 ) ) ;
#12489=CARTESIAN_POINT ( 'NONE',  ( -49.86468353124999453, 43.75937500034140015, -16.20201782572375393 ) ) ;
#12494=CARTESIAN_POINT ( 'NONE',  ( 30.81806926056962936, 37.15937500034139873, -42.41743335407647209 ) ) ;
#12495=CARTESIAN_POINT ( 'NONE',  ( 50.00000000000000711, 40.68125000068280173, 16.24598481164530739 ) ) ;
#12497=CARTESIAN_POINT ( 'NONE',  ( 47.84248829804716507, 24.99999999999999289, -14.05740927763599757 ) ) ;
#12498=CARTESIAN_POINT ( 'NONE',  ( 40.45084971874737079, 46.98125000068280599, -29.38926261462366440 ) ) ;
#12506=CARTESIAN_POINT ( 'NONE',  ( 40.34137639590981905, 40.72187500034139873, 29.30972558990010768 ) ) ;
#12510=CARTESIAN_POINT ( 'NONE',  ( 15.40903463028482356, 42.45937500034140299, 47.42413220539093999 ) ) ;
#12512=CARTESIAN_POINT ( 'NONE',  ( -15.45084971874736368, 24.18125000068279817, 47.55282581475768211 ) ) ;
#12514=ADVANCED_FACE ( 'NONE', ( #4559 ), #8607, .T. ) ;
#12518=CARTESIAN_POINT ( 'NONE',  ( 49.99999999999999289, 31.09999999999999787, -16.24598481164532160 ) ) ;
#12519=CARTESIAN_POINT ( 'NONE',  ( 30.81806926056964002, 26.62187500034139731, 42.41743335407647209 ) ) ;
#12524=CARTESIAN_POINT ( 'NONE',  ( -30.81806926056962226, 34.22187500034139873, 42.41743335407647919 ) ) ;
#12525=CARTESIAN_POINT ( 'NONE',  ( -15.45084971874737256, 41.38125000068279746, -47.55282581475767500 ) ) ;
#12536=DIRECTION ( 'NONE',  ( 1.000000000000000000, 0.000000000000000000, 0.000000000000000000 ) ) ;
#12540=CARTESIAN_POINT ( 'NONE',  ( 30.81806926056964002, 24.55937500034139376, 42.41743335407647209 ) ) ;
#12544=CARTESIAN_POINT ( 'NONE',  ( 40.45084971874737079, 36.98125000068279888, -29.38926261462366440 ) ) ;
#12548=CARTESIAN_POINT ( 'NONE',  ( 50.00000000000000711, 38.68125000068280173, 16.24598481164530739 ) ) ;
#12551=CARTESIAN_POINT ( 'NONE',  ( 0.000000000000000000, 193.4213562373095385, 0.000000000000000000 ) ) ;
#12552=CARTESIAN_POINT ( 'NONE',  ( 15.45084971874737789, 26.38125000068280102, 47.55282581475767500 ) ) ;
#12557=DIRECTION ( 'NONE',  ( -0.000000000000000000, -1.000000000000000000, -0.000000000000000000 ) ) ;
#12560=CARTESIAN_POINT ( 'NONE',  ( -49.99999999999999289, 22.09999999999999787, 16.24598481164533226 ) ) ;
#12563=CARTESIAN_POINT ( 'NONE',  ( 49.86468353125001585, 46.75937500034140015, 16.20201782572375038 ) ) ;
#12569=CARTESIAN_POINT ( 'NONE',  ( -3.210462471511496205E-15, 31.35937500034139092, -52.43083105670540789 ) ) ;
#12570=CARTESIAN_POINT ( 'NONE',  ( 7.919222016226875382, 41.22999571913594963, -49.99999999999997158 ) ) ;
#12572=CARTESIAN_POINT ( 'NONE',  ( 47.65000835890761266, 25.00000000000000711, -14.69569212618958787 ) ) ;
#12573=CARTESIAN_POINT ( 'NONE',  ( 15.45084971874736723, 47.18125000068280173, -47.55282581475768211 ) ) ;
#12576=CARTESIAN_POINT ( 'NONE',  ( 30.90169943749473802, 43.30000000000000426, -42.53254041760200721 ) ) ;
#12582=CARTESIAN_POINT ( 'NONE',  ( 30.81806926056962936, 31.22187500034139873, -42.41743335407647209 ) ) ;
#12586=CARTESIAN_POINT ( 'NONE',  ( 49.86468353125001585, 34.75937500034138594, 16.20201782572375038 ) ) ;
#12590=CARTESIAN_POINT ( 'NONE',  ( 30.90169943749475578, 24.48125000068280244, 42.53254041760200010 ) ) ;
#12593=CARTESIAN_POINT ( 'NONE',  ( 49.86468353124999453, 23.02187500034139944, -16.20201782572376459 ) ) ;
#12598=CARTESIAN_POINT ( 'NONE',  ( 9.657523855033129090E-15, 46.50000000000000711, 52.57311121191334990 ) ) ;
#12604=CARTESIAN_POINT ( 'NONE',  ( -30.81806926056963292, 33.62187500034139731, -42.41743335407647209 ) ) ;
#12624=CARTESIAN_POINT ( 'NONE',  ( 49.86468353124999453, 22.95937500034139589, -16.20201782572376459 ) ) ;
#12632=CARTESIAN_POINT ( 'NONE',  ( -3.111920190527341144E-15, 29.50000000000000000, -50.00000000000000000 ) ) ;
#12633=CARTESIAN_POINT ( 'NONE',  ( -30.90169943749474513, 37.70000000000000284, -42.53254041760200721 ) ) ;
#12636=AXIS2_PLACEMENT_3D ( 'NONE', #15862, #14433, #9465 ) ;
#12640=AXIS2_PLACEMENT_3D ( 'NONE', #4848, #6560, #11619 ) ;
#12641=DIRECTION ( 'NONE',  ( -0.000000000000000000, -1.000000000000000000, -0.000000000000000000 ) ) ;
#12646=CARTESIAN_POINT ( 'NONE',  ( 9.657523855033129090E-15, 22.50000000000000355, 52.57311121191334990 ) ) ;
#12648=EDGE_CURVE ( 'NONE', #1121, #10705, #9132, .T. ) ;
#12650=CARTESIAN_POINT ( 'NONE',  ( -15.40903463028481646, 41.45937500034140299, -47.42413220539093999 ) ) ;
#12659=CARTESIAN_POINT ( 'NONE',  ( 49.86468353124999453, 26.95937500034139944, -16.20201782572376459 ) ) ;
#12660=CARTESIAN_POINT ( 'NONE',  ( 15.45084971874737789, 26.60000000000000142, 47.55282581475767500 ) ) ;
#12662=CARTESIAN_POINT ( 'NONE',  ( 48.24365308685505482, 25.00000000000000000, -12.61207274728973005 ) ) ;
#12663=CARTESIAN_POINT ( 'NONE',  ( -30.81806926056962226, 36.22187500034139163, 42.41743335407647209 ) ) ;
#12664=CARTESIAN_POINT ( 'NONE',  ( 30.90169943749475223, 30.48125000068279533, 42.53254041760199300 ) ) ;
#12669=DIRECTION ( 'NONE',  ( 0.000000000000000000, -1.000000000000000000, 0.000000000000000000 ) ) ;
#12672=CARTESIAN_POINT ( 'NONE',  ( -15.40903463028480580, 30.32187500034140015, 47.42413220539094709 ) ) ;
#12674=ORIENTED_EDGE ( 'NONE', *, *, #14806, .T. ) ;
#12676=CARTESIAN_POINT ( 'NONE',  ( -30.81806926056963292, 35.55937500034139020, -42.41743335407646498 ) ) ;
#12682=CARTESIAN_POINT ( 'NONE',  ( -49.86468353125000164, 45.85937500034140157, 0.000000000000000000 ) ) ;
#12683=CARTESIAN_POINT ( 'NONE',  ( 1.293669679204937499E-13, 39.28125000068280315, -50.00000000000000000 ) ) ;
#12684=CARTESIAN_POINT ( 'NONE',  ( -40.34137639590981905, 21.72187500034139518, -29.30972558990011478 ) ) ;
#12685=CARTESIAN_POINT ( 'NONE',  ( 0.000000000000000000, 272.0000000000000000, -79.49773270518484480 ) ) ;
#12687=CARTESIAN_POINT ( 'NONE',  ( -40.45084971874737079, 25.98125000068279888, 29.38926261462367151 ) ) ;
#12688=CARTESIAN_POINT ( 'NONE',  ( -30.81806926056962226, 20.22187500034139163, 42.41743335407647919 ) ) ;
#12690=CARTESIAN_POINT ( 'NONE',  ( 30.81806926056962936, 49.22187500034139873, -42.41743335407647209 ) ) ;
#12702=CARTESIAN_POINT ( 'NONE',  ( -1.240322475938754499E-13, 40.50000000000000000, 50.00000000000000000 ) ) ;
#12707=CARTESIAN_POINT ( 'NONE',  ( 9.631387414534489405E-15, 22.35937500034139802, 52.43083105670540789 ) ) ;
#12710=EDGE_LOOP ( 'NONE', ( #10041, #6553, #4739, #5082 ) ) ;
#12726=CARTESIAN_POINT ( 'NONE',  ( 0.000000000000000000, 193.4213562373095385, 0.000000000000000000 ) ) ;
#12730=( BOUNDED_CURVE ( )  B_SPLINE_CURVE ( 2, ( #5083, #1640, #1390, #6736, #14106, #13038, #12959, #11631, #56, #10304, #5404, #3980, #10384 ),
 .UNSPECIFIED., .F., .F. ) 
 B_SPLINE_CURVE_WITH_KNOTS ( ( 3, 2, 2, 2, 2, 2, 3 ),
 ( 0.7833333333333333259, 0.7866666666666666252, 0.7933333333333333348, 0.8000000000000000444, 0.8066666666666666430, 0.8133333333333333526, 0.8166666666666666519 ),
 .UNSPECIFIED. ) 
 CURVE ( )  GEOMETRIC_REPRESENTATION_ITEM ( )  RATIONAL_B_SPLINE_CURVE ( ( 0.9755282581475768211, 0.9755282581475768211, 1.000000000000000000, 0.9510565162951535312, 1.000000000000000000, 0.9510565162951535312, 1.000000000000000000, 0.9510565162951535312, 1.000000000000000000, 0.9510565162951535312, 1.000000000000000000, 0.9755282581475768211, 0.9755282581475768211 ) ) 
 REPRESENTATION_ITEM ( '' )  );
#12731=CARTESIAN_POINT ( 'NONE',  ( -30.81806926056963292, 45.55937500034139731, -42.41743335407647209 ) ) ;
#12736=CARTESIAN_POINT ( 'NONE',  ( -30.81806926056962226, 26.15937500034139163, 42.41743335407647919 ) ) ;
#12737=ORIENTED_EDGE ( 'NONE', *, *, #5847, .T. ) ;
#12741=CARTESIAN_POINT ( 'NONE',  ( -49.86468353125000164, 33.92187500034139447, 0.000000000000000000 ) ) ;
#12745=CYLINDRICAL_SURFACE ( 'NONE', #480, 79.49773270518484480 ) ;
#12747=CARTESIAN_POINT ( 'NONE',  ( -49.99999999999999289, 29.68125000068279817, -16.24598481164531449 ) ) ;
#12750=CARTESIAN_POINT ( 'NONE',  ( -49.86468353124999453, 32.02187500034139589, 16.20201782572377525 ) ) ;
#12755=CARTESIAN_POINT ( 'NONE',  ( -15.40903463028481646, 33.45937500034139589, -47.42413220539093999 ) ) ;
#12759=CARTESIAN_POINT ( 'NONE',  ( -49.86468353124999453, 45.95937500034138878, 16.20201782572377525 ) ) ;
#12761=CARTESIAN_POINT ( 'NONE',  ( 15.40903463028482356, 24.52187500034139589, 47.42413220539093999 ) ) ;
#12766=CARTESIAN_POINT ( 'NONE',  ( -3.219174618344376363E-15, 47.49999999999999289, -52.57311121191334990 ) ) ;
#12769=FACE_OUTER_BOUND ( 'NONE', #5787, .T. ) ;
#12782=CARTESIAN_POINT ( 'NONE',  ( -3.111920190527341144E-15, 35.28125000068280315, -50.00000000000000000 ) ) ;
#12785=CARTESIAN_POINT ( 'NONE',  ( -40.34137639590981195, 48.12187500034139731, 29.30972558990012189 ) ) ;
#12793=CARTESIAN_POINT ( 'NONE',  ( 0.000000000000000000, 25.00000000000000000, 0.000000000000000000 ) ) ;
#12795=FACE_OUTER_BOUND ( 'NONE', #7963, .T. ) ;
#12802=CARTESIAN_POINT ( 'NONE',  ( -15.45084971874736368, 24.40000000000000213, 47.55282581475768211 ) ) ;
#12803=LINE ( 'NONE', #6673, #8822 ) ;
#12805=VERTEX_POINT ( 'NONE', #9114 ) ;
#12806=CARTESIAN_POINT ( 'NONE',  ( 49.86468353125000164, 38.85937500034139447, -6.106662507704105588E-15 ) ) ;
#12807=ORIENTED_EDGE ( 'NONE', *, *, #9049, .F. ) ;
#12811=CARTESIAN_POINT ( 'NONE',  ( -49.86468353124999453, 27.95937500034139944, 16.20201782572377525 ) ) ;
#12813=EDGE_LOOP ( 'NONE', ( #6462, #7687, #6921, #4463 ) ) ;
#12816=CARTESIAN_POINT ( 'NONE',  ( 47.02241032844496971, 25.00000000000000000, -16.59456509147096881 ) ) ;
#12817=CARTESIAN_POINT ( 'NONE',  ( -30.81806926056963292, 31.62187500034140086, -42.41743335407646498 ) ) ;
#12823=( BOUNDED_CURVE ( )  B_SPLINE_CURVE ( 2, ( #12205, #13688, #3224, #807, #3562, #9881, #13364 ),
 .UNSPECIFIED., .F., .F. ) 
 B_SPLINE_CURVE_WITH_KNOTS ( ( 3, 2, 2, 3 ),
 ( 0.8166666666666666519, 0.8199999999999999512, 0.8266666666666666607, 0.8333333333333333703 ),
 .UNSPECIFIED. ) 
 CURVE ( )  GEOMETRIC_REPRESENTATION_ITEM ( )  RATIONAL_B_SPLINE_CURVE ( ( 0.9755282581475768211, 0.9755282581475768211, 1.000000000000000000, 0.9510565162951535312, 1.000000000000000000, 0.9510565162951535312, 1.000000000000000000 ) ) 
 REPRESENTATION_ITEM ( '' )  );
#12824=FACE_OUTER_BOUND ( 'NONE', #9892, .T. ) ;
#12827=CARTESIAN_POINT ( 'NONE',  ( -15.40903463028481646, 31.52187500034139944, -47.42413220539093999 ) ) ;
#12832=CARTESIAN_POINT ( 'NONE',  ( -15.40903463028480580, 36.25937500034140015, 47.42413220539094709 ) ) ;
#12836=CARTESIAN_POINT ( 'NONE',  ( 9.631387414534489405E-15, 46.35937500034139447, 52.43083105670540789 ) ) ;
#12838=CARTESIAN_POINT ( 'NONE',  ( -49.86468353124999453, 25.82187500034139305, -16.20201782572375393 ) ) ;
#12840=AXIS2_PLACEMENT_3D ( 'NONE', #1905, #14874, #5755 ) ;
#12845=CARTESIAN_POINT ( 'NONE',  ( -49.99999999999999289, 47.89999999999999858, -16.24598481164531449 ) ) ;
#12853=CARTESIAN_POINT ( 'NONE',  ( 50.00000000000000711, 36.68125000068280173, 16.24598481164530739 ) ) ;
#12856=LINE ( 'NONE', #1624, #13420 ) ;
#12858=CARTESIAN_POINT ( 'NONE',  ( 15.40903463028482356, 46.52187500034139589, 47.42413220539093999 ) ) ;
#12861=AXIS2_PLACEMENT_3D ( 'NONE', #376, #3623, #15328 ) ;
#12868=CARTESIAN_POINT ( 'NONE',  ( 40.34137639590981195, 49.12187500034139731, -29.30972558990011834 ) ) ;
#12869=ORIENTED_EDGE ( 'NONE', *, *, #320, .T. ) ;
#12877=CARTESIAN_POINT ( 'NONE',  ( 50.00000000000000000, 29.00000000000000000, -6.123233995736766085E-15 ) ) ;
#12887=CARTESIAN_POINT ( 'NONE',  ( 15.45084971874737789, 24.60000000000000142, 47.55282581475767500 ) ) ;
#12891=CARTESIAN_POINT ( 'NONE',  ( -49.86468353124999453, 35.95937500034139589, 16.20201782572377525 ) ) ;
#12896=CARTESIAN_POINT ( 'NONE',  ( -49.86468353124999453, 31.95937500034139944, 16.20201782572377525 ) ) ;
#12898=ORIENTED_EDGE ( 'NONE', *, *, #16428, .F. ) ;
#12904=CARTESIAN_POINT ( 'NONE',  ( -30.81806926056963292, 35.62187500034140442, -42.41743335407646498 ) ) ;
#12909=CYLINDRICAL_SURFACE ( 'NONE', #3367, 50.00000000000000000 ) ;
#12913=AXIS2_PLACEMENT_3D ( 'NONE', #13649, #3351, #8260 ) ;
#12914=CARTESIAN_POINT ( 'NONE',  ( -30.81806926056963292, 29.62187500034139376, -42.41743335407647209 ) ) ;
#12920=CARTESIAN_POINT ( 'NONE',  ( 15.40903463028481113, 37.25937500034140015, -47.42413220539094709 ) ) ;
#12923=CARTESIAN_POINT ( 'NONE',  ( 50.00000000000000711, 20.68125000068280173, 16.24598481164530739 ) ) ;
#12928=CARTESIAN_POINT ( 'NONE',  ( -49.86468353125000164, 23.92187500034139447, 0.000000000000000000 ) ) ;
#12932=CARTESIAN_POINT ( 'NONE',  ( -49.99999999999999289, 25.68125000068279817, -16.24598481164531449 ) ) ;
#12933=CARTESIAN_POINT ( 'NONE',  ( -15.40903463028480580, 20.32187500034139660, 47.42413220539094709 ) ) ;
#12936=CARTESIAN_POINT ( 'NONE',  ( 40.34137639590981905, 48.72187500034139873, 29.30972558990010768 ) ) ;
#12942=CARTESIAN_POINT ( 'NONE',  ( -49.99999999999999289, 35.88125000068279746, 16.24598481164533226 ) ) ;
#12952=CYLINDRICAL_SURFACE ( 'NONE', #10745, 50.00000000000000000 ) ;
#12956=CARTESIAN_POINT ( 'NONE',  ( 30.81806926056964002, 20.55937500034139376, 42.41743335407647209 ) ) ;
#12959=CARTESIAN_POINT ( 'NONE',  ( -50.00000000000000000, 26.00000000000000355, 0.000000000000000000 ) ) ;
#12962=LINE ( 'NONE', #4154, #2586 ) ;
#12968=PLANE ( 'NONE',  #13774 ) ;
#12979=CARTESIAN_POINT ( 'NONE',  ( 30.81806926056962936, 39.15937500034139873, -42.41743335407647209 ) ) ;
#12983=CARTESIAN_POINT ( 'NONE',  ( 49.86468353124999453, 22.95937500034139589, -16.20201782572376459 ) ) ;
#12988=CARTESIAN_POINT ( 'NONE',  ( 40.34137639590981195, 29.12187500034139376, -29.30972558990011834 ) ) ;
#12997=CARTESIAN_POINT ( 'NONE',  ( -49.86468353124999453, 28.02187500034139234, 16.20201782572377525 ) ) ;
#13000=CARTESIAN_POINT ( 'NONE',  ( 9.631387414534489405E-15, 28.35937500034139447, 52.43083105670540789 ) ) ;
#13003=CARTESIAN_POINT ( 'NONE',  ( 30.81806926056964002, 46.55937500034139020, 42.41743335407647209 ) ) ;
#13011=ADVANCED_FACE ( 'NONE', ( #11177 ), #8573, .T. ) ;
#13012=CARTESIAN_POINT ( 'NONE',  ( -30.90169943749473802, 38.29999999999999716, 42.53254041760200721 ) ) ;
#13014=CARTESIAN_POINT ( 'NONE',  ( 30.81806926056962936, 45.22187500034139873, -42.41743335407647209 ) ) ;
#13017=CARTESIAN_POINT ( 'NONE',  ( 49.86468353124999453, 48.95937500034140299, -16.20201782572376104 ) ) ;
#13019=CARTESIAN_POINT ( 'NONE',  ( -50.00000000000000000, 39.78125000068279604, 0.000000000000000000 ) ) ;
#13021=EDGE_CURVE ( 'NONE', #15674, #1275, #11001, .T. ) ;
#13023=DIRECTION ( 'NONE',  ( 0.000000000000000000, 0.000000000000000000, -1.000000000000000000 ) ) ;
#13025=CARTESIAN_POINT ( 'NONE',  ( 49.86468353125000164, 44.92187500034140157, -6.106662507704105588E-15 ) ) ;
#13033=CARTESIAN_POINT ( 'NONE',  ( 50.00000000000000000, 28.78125000068279959, -6.123233995736766085E-15 ) ) ;
#13035=CARTESIAN_POINT ( 'NONE',  ( 49.86468353125000164, 46.92187500034139447, -6.106662507704105588E-15 ) ) ;
#13038=CARTESIAN_POINT ( 'NONE',  ( -49.99999999999999289, 26.10000000000000142, 16.24598481164533226 ) ) ;
#13048=ADVANCED_FACE ( 'NONE', ( #14974 ), #10257, .T. ) ;
#13051=DIRECTION ( 'NONE',  ( 0.000000000000000000, 0.000000000000000000, 1.000000000000000000 ) ) ;
#13057=CARTESIAN_POINT ( 'NONE',  ( 15.40903463028482356, 38.45937500034139589, 47.42413220539093999 ) ) ;
#13059=EDGE_LOOP ( 'NONE', ( #2671, #15856, #2108, #5798 ) ) ;
#13060=CARTESIAN_POINT ( 'NONE',  ( -49.99999999999999289, 47.88125000068280457, 16.24598481164533226 ) ) ;
#13062=CARTESIAN_POINT ( 'NONE',  ( 9.631387414534489405E-15, 20.35937500034139092, 52.43083105670540789 ) ) ;
#13067=DIRECTION ( 'NONE',  ( -0.000000000000000000, -1.000000000000000000, -0.000000000000000000 ) ) ;
#13068=CARTESIAN_POINT ( 'NONE',  ( -49.86468353125000164, 25.92187500034139802, 0.000000000000000000 ) ) ;
#13069=( BOUNDED_CURVE ( )  B_SPLINE_CURVE ( 2, ( #5922, #5671, #10902, #14792, #8559, #8486, #7169, #13552, #9498, #16140, #9651, #15799, #14703 ),
 .UNSPECIFIED., .F., .T. ) 
 B_SPLINE_CURVE_WITH_KNOTS ( ( 3, 2, 2, 2, 2, 2, 3 ),
 ( 0.3500000000000000333, 0.3533333333333333326, 0.3599999999999999867, 0.3666666666666666408, 0.3733333333333333504, 0.3800000000000000044, 0.3833333333333333592 ),
 .UNSPECIFIED. ) 
 CURVE ( )  GEOMETRIC_REPRESENTATION_ITEM ( )  RATIONAL_B_SPLINE_CURVE ( ( 0.9755282581475768211, 0.9755282581475770431, 1.000000000000000000, 0.9510565162951535312, 1.000000000000000000, 0.9510565162951535312, 1.000000000000000000, 0.9510565162951535312, 1.000000000000000000, 0.9510565162951535312, 1.000000000000000000, 0.9755282581475765991, 0.9755282581475768211 ) ) 
 REPRESENTATION_ITEM ( '' )  );
#13074=CARTESIAN_POINT ( 'NONE',  ( -30.90169943749473802, 32.30000000000000426, 42.53254041760200721 ) ) ;
#13079=CARTESIAN_POINT ( 'NONE',  ( -15.40903463028480580, 30.25937500034140015, 47.42413220539094709 ) ) ;
#13080=ORIENTED_EDGE ( 'NONE', *, *, #1432, .F. ) ;
#13082=CARTESIAN_POINT ( 'NONE',  ( -49.86468353124999453, 39.75937500034139305, -16.20201782572375393 ) ) ;
#13089=CARTESIAN_POINT ( 'NONE',  ( -30.90169943749473802, 42.30000000000000426, 42.53254041760200721 ) ) ;
#13090=AXIS2_PLACEMENT_3D ( 'NONE', #9268, #3185, #14562 ) ;
#13092=CARTESIAN_POINT ( 'NONE',  ( 49.86468353124999453, 43.02187500034138878, -16.20201782572376459 ) ) ;
#13093=EDGE_CURVE ( 'NONE', #14942, #7759, #6279, .T. ) ;
#13097=ORIENTED_EDGE ( 'NONE', *, *, #2891, .F. ) ;
#13098=CARTESIAN_POINT ( 'NONE',  ( -15.45084971874736368, 30.18125000068280173, 47.55282581475768211 ) ) ;
#13100=EDGE_LOOP ( 'NONE', ( #6614, #9283 ) ) ;
#13103=CARTESIAN_POINT ( 'NONE',  ( -49.86468353125000164, 49.92187500034140157, 0.000000000000000000 ) ) ;
#13105=EDGE_CURVE ( 'NONE', #8121, #13641, #7246, .T. ) ;
#13106=LINE ( 'NONE', #1710, #15782 ) ;
#13110=CARTESIAN_POINT ( 'NONE',  ( -30.90169943749473447, 46.08125000068279320, 42.53254041760200721 ) ) ;
#13112=CARTESIAN_POINT ( 'NONE',  ( 49.86468353124999453, 20.95937500034138878, -16.20201782572376459 ) ) ;
#13114=DIRECTION ( 'NONE',  ( 0.000000000000000000, 1.000000000000000000, 0.000000000000000000 ) ) ;
#13124=DIRECTION ( 'NONE',  ( 0.000000000000000000, 0.000000000000000000, -1.000000000000000000 ) ) ;
#13125=EDGE_CURVE ( 'NONE', #4476, #12134, #11654, .T. ) ;
#13128=CARTESIAN_POINT ( 'NONE',  ( -3.111920190527341144E-15, 43.50000000000000711, -50.00000000000000000 ) ) ;
#13131=DIRECTION ( 'NONE',  ( -0.000000000000000000, -1.000000000000000000, -0.000000000000000000 ) ) ;
#13133=AXIS2_PLACEMENT_3D ( 'NONE', #1370, #6383, #11366 ) ;
#13134=CARTESIAN_POINT ( 'NONE',  ( 40.34137639590981195, 37.05937500034139731, -29.30972558990011834 ) ) ;
#13139=CARTESIAN_POINT ( 'NONE',  ( 49.86468353125000164, 24.85937500034139802, -6.106662507704105588E-15 ) ) ;
#13145=CARTESIAN_POINT ( 'NONE',  ( -30.81806926056963292, 27.62187500034139731, -42.41743335407646498 ) ) ;
#13149=DIRECTION ( 'NONE',  ( 0.000000000000000000, 0.000000000000000000, -1.000000000000000000 ) ) ;
#13150=EDGE_CURVE ( 'NONE', #10026, #4982, #2820, .T. ) ;
#13152=CARTESIAN_POINT ( 'NONE',  ( 49.99999999999999289, 37.10000000000000142, -16.24598481164532160 ) ) ;
#13154=CARTESIAN_POINT ( 'NONE',  ( 7.513064459987437071E-14, 42.28125000068280315, 50.00000000000000000 ) ) ;
#13157=CARTESIAN_POINT ( 'NONE',  ( -49.86468353125000164, 29.85937500034139802, 0.000000000000000000 ) ) ;
#13161=CARTESIAN_POINT ( 'NONE',  ( -30.81806926056962226, 44.15937500034139163, 42.41743335407647919 ) ) ;
#13174=CARTESIAN_POINT ( 'NONE',  ( 15.45084971874736723, 39.40000000000000568, -47.55282581475768211 ) ) ;
#13176=CARTESIAN_POINT ( 'NONE',  ( -49.86468353125000164, 41.92187500034139447, 0.000000000000000000 ) ) ;
#13179=DIRECTION ( 'NONE',  ( -0.000000000000000000, -1.000000000000000000, -0.000000000000000000 ) ) ;
#13185=CARTESIAN_POINT ( 'NONE',  ( -30.90169943749473802, 32.08125000068280031, 42.53254041760200721 ) ) ;
#13188=CARTESIAN_POINT ( 'NONE',  ( 2.600676159226420495E-13, 33.28125000068279604, -49.99999999999999289 ) ) ;
#13189=CARTESIAN_POINT ( 'NONE',  ( -49.86468353124999453, 49.82187500034139305, -16.20201782572375393 ) ) ;
#13197=CARTESIAN_POINT ( 'NONE',  ( -7.919222016226816763, 45.33250428222963535, -49.99999999999999289 ) ) ;
#13199=CARTESIAN_POINT ( 'NONE',  ( 40.34137639590981195, 45.12187500034139731, -29.30972558990011834 ) ) ;
#13204=DIRECTION ( 'NONE',  ( 0.000000000000000000, 0.000000000000000000, 1.000000000000000000 ) ) ;
#13208=CARTESIAN_POINT ( 'NONE',  ( -1.240322475938754499E-13, 38.50000000000000711, 50.00000000000000000 ) ) ;
#13218=CARTESIAN_POINT ( 'NONE',  ( -49.86468353125000164, 29.85937500034139802, 0.000000000000000000 ) ) ;
#13223=PLANE ( 'NONE',  #10498 ) ;
#13225=CARTESIAN_POINT ( 'NONE',  ( -49.86468353125000164, 19.85937500034139447, 0.000000000000000000 ) ) ;
#13229=CARTESIAN_POINT ( 'NONE',  ( -40.45084971874737789, 47.80000000000000426, -29.38926261462365730 ) ) ;
#13230=CARTESIAN_POINT ( 'NONE',  ( -3.111920190527341144E-15, 35.50000000000000000, -50.00000000000000000 ) ) ;
#13239=CARTESIAN_POINT ( 'NONE',  ( -40.45084971874737079, 32.20000000000000284, 29.38926261462367151 ) ) ;
#13243=CARTESIAN_POINT ( 'NONE',  ( 30.81806926056962936, 31.15937500034139163, -42.41743335407646498 ) ) ;
#13246=CARTESIAN_POINT ( 'NONE',  ( 49.86468353124999453, 40.95937500034140299, -16.20201782572376459 ) ) ;
#13252=CARTESIAN_POINT ( 'NONE',  ( 15.40903463028481113, 29.32187500034139660, -47.42413220539094709 ) ) ;
#13253=CARTESIAN_POINT ( 'NONE',  ( -50.00000000000000000, 42.00000000000000000, 0.000000000000000000 ) ) ;
#13255=CARTESIAN_POINT ( 'NONE',  ( 40.34137639590981195, 47.12187500034140442, -29.30972558990011834 ) ) ;
#13260=CARTESIAN_POINT ( 'NONE',  ( -30.81806926056962226, 46.15937500034139873, 42.41743335407647209 ) ) ;
#13262=CARTESIAN_POINT ( 'NONE',  ( 9.657523855033129090E-15, 30.28125000068279604, 52.57311121191334990 ) ) ;
#13265=CARTESIAN_POINT ( 'NONE',  ( 50.00000000000000711, 32.68125000068279462, 16.24598481164530739 ) ) ;
#13266=CARTESIAN_POINT ( 'NONE',  ( -49.86468353124999453, 38.02187500034139589, 16.20201782572377169 ) ) ;
#13276=CARTESIAN_POINT ( 'NONE',  ( 30.81806926056962936, 41.22187500034139873, -42.41743335407647209 ) ) ;
#13281=LINE ( 'NONE', #8292, #6915 ) ;
#13286=CARTESIAN_POINT ( 'NONE',  ( -2.547328955960238000E-13, 34.28125000068279604, 49.99999999999999289 ) ) ;
#13287=SURFACE_SIDE_STYLE ('',( #16118 ) ) ;
#13291=CARTESIAN_POINT ( 'NONE',  ( 30.90169943749473802, 37.29999999999999716, -42.53254041760200721 ) ) ;
#13294=CARTESIAN_POINT ( 'NONE',  ( -15.40903463028481646, 29.45937500034139589, -47.42413220539093999 ) ) ;
#13298=CARTESIAN_POINT ( 'NONE',  ( 30.90169943749475578, 40.48125000068279888, 42.53254041760200010 ) ) ;
#13300=CARTESIAN_POINT ( 'NONE',  ( -40.34137639590981195, 24.05937500034139731, 29.30972558990012189 ) ) ;
#13303=CARTESIAN_POINT ( 'NONE',  ( -40.45084971874737079, 48.20000000000000284, 29.38926261462367151 ) ) ;
#13306=CARTESIAN_POINT ( 'NONE',  ( 40.34137639590981195, 31.12187500034139731, -29.30972558990011834 ) ) ;
#13310=CARTESIAN_POINT ( 'NONE',  ( -49.99999999999999289, 42.09999999999999432, 16.24598481164533226 ) ) ;
#13313=CARTESIAN_POINT ( 'NONE',  ( 40.45084971874737789, 32.80000000000000426, 29.38926261462365375 ) ) ;
#13318=CARTESIAN_POINT ( 'NONE',  ( -49.86468353124999453, 29.75937500034139305, -16.20201782572375393 ) ) ;
#13321=CARTESIAN_POINT ( 'NONE',  ( -49.86468353124999453, 43.75937500034140015, -16.20201782572375393 ) ) ;
#13324=CARTESIAN_POINT ( 'NONE',  ( -5.823736356558307894E-14, 44.28125000068280315, 50.00000000000000000 ) ) ;
#13328=CARTESIAN_POINT ( 'NONE',  ( 15.40903463028482356, 30.52187500034139589, 47.42413220539093999 ) ) ;
#13329=CARTESIAN_POINT ( 'NONE',  ( 49.99999999999999289, 41.10000000000000853, -16.24598481164532160 ) ) ;
#13331=CARTESIAN_POINT ( 'NONE',  ( 40.34137639590981905, 44.72187500034139163, 29.30972558990010768 ) ) ;
#13332=EDGE_CURVE ( 'NONE', #4817, #5627, #8300, .T. ) ;
#13337=EDGE_LOOP ( 'NONE', ( #10749, #9304, #16101, #16453 ) ) ;
#13338=CARTESIAN_POINT ( 'NONE',  ( -49.99999999999999289, 27.88125000068279746, 16.24598481164533226 ) ) ;
#13343=CARTESIAN_POINT ( 'NONE',  ( -15.40903463028481646, 39.52187500034139589, -47.42413220539093999 ) ) ;
#13345=DIRECTION ( 'NONE',  ( 0.000000000000000000, 1.000000000000000000, 0.000000000000000000 ) ) ;
#13348=EDGE_CURVE ( 'NONE', #3492, #1639, #2016, .T. ) ;
#13354=CARTESIAN_POINT ( 'NONE',  ( -15.40903463028480580, 42.32187500034139305, 47.42413220539094709 ) ) ;
#13355=ORIENTED_EDGE ( 'NONE', *, *, #11930, .T. ) ;
#13364=CARTESIAN_POINT ( 'NONE',  ( 50.00000000000000000, 25.00000000000000000, -6.123233995736766085E-15 ) ) ;
#13365=DIRECTION ( 'NONE',  ( 0.000000000000000000, -0.000000000000000000, 1.000000000000000000 ) ) ;
#13372=CARTESIAN_POINT ( 'NONE',  ( -49.86468353125000164, 31.85937500034139447, 0.000000000000000000 ) ) ;
#13376=CARTESIAN_POINT ( 'NONE',  ( 40.45084971874737079, 44.98125000068279888, -29.38926261462366440 ) ) ;
#13381=CARTESIAN_POINT ( 'NONE',  ( 40.45084971874737789, 34.80000000000000426, 29.38926261462365375 ) ) ;
#13385=CARTESIAN_POINT ( 'NONE',  ( 40.45084971874737079, 36.98125000068279888, -29.38926261462366440 ) ) ;
#13389=CARTESIAN_POINT ( 'NONE',  ( 40.45084971874737789, 30.80000000000000071, 29.38926261462365375 ) ) ;
#13391=CARTESIAN_POINT ( 'NONE',  ( 15.40903463028481113, 47.25937500034140015, -47.42413220539094709 ) ) ;
#13392=ORIENTED_EDGE ( 'NONE', *, *, #1880, .F. ) ;
#13395=EDGE_LOOP ( 'NONE', ( #11824, #15234, #6054, #16261 ) ) ;
#13397=CARTESIAN_POINT ( 'NONE',  ( 15.40903463028482356, 38.45937500034139589, 47.42413220539093999 ) ) ;
#13400=CARTESIAN_POINT ( 'NONE',  ( 7.919222016226809657, 45.22999571913594963, -50.00000000000000000 ) ) ;
#13403=CARTESIAN_POINT ( 'NONE',  ( 9.631387414534489405E-15, 30.42187500034139447, 52.43083105670540789 ) ) ;
#13406=CARTESIAN_POINT ( 'NONE',  ( -30.81806926056963292, 35.62187500034140442, -42.41743335407647209 ) ) ;
#13407=VECTOR ( 'NONE', #13786, 1000.000000000000000 ) ;
#13411=VERTEX_POINT ( 'NONE', #4424 ) ;
#13413=CARTESIAN_POINT ( 'NONE',  ( 40.34137639590981905, 44.65937500034139163, 29.30972558990010768 ) ) ;
#13415=CARTESIAN_POINT ( 'NONE',  ( 50.00000000000000711, 30.68125000068279462, 16.24598481164530739 ) ) ;
#13420=VECTOR ( 'NONE', #5470, 1000.000000000000000 ) ;
#13424=CARTESIAN_POINT ( 'NONE',  ( 49.86468353125000164, 38.92187500034139447, -6.106662507704105588E-15 ) ) ;
#13428=CARTESIAN_POINT ( 'NONE',  ( -40.34137639590981195, 24.12187500034139731, 29.30972558990012189 ) ) ;
#13437=CARTESIAN_POINT ( 'NONE',  ( 40.34137639590981195, 39.12187500034139731, -29.30972558990011834 ) ) ;
#13442=DIRECTION ( 'NONE',  ( 1.067350013832299517E-17, 0.9961946980917455452, -0.08715574274765836016 ) ) ;
#13443=CARTESIAN_POINT ( 'NONE',  ( 0.000000000000000000, 193.4213562373095385, 0.000000000000000000 ) ) ;
#13450=CARTESIAN_POINT ( 'NONE',  ( -40.45084971874737789, 29.80000000000000071, -29.38926261462365730 ) ) ;
#13458=CARTESIAN_POINT ( 'NONE',  ( -40.34137639590981905, 29.65937500034139518, -29.30972558990011478 ) ) ;
#13463=CARTESIAN_POINT ( 'NONE',  ( -49.99999999999999289, 45.68125000068280173, -16.24598481164531449 ) ) ;
#13464=CARTESIAN_POINT ( 'NONE',  ( -2.445080149700054274E-14, 46.50000000000000711, 50.00000000000000000 ) ) ;
#13466=ORIENTED_EDGE ( 'NONE', *, *, #7735, .T. ) ;
#13470=DIRECTION ( 'NONE',  ( -0.000000000000000000, -1.000000000000000000, -0.000000000000000000 ) ) ;
#13478=CARTESIAN_POINT ( 'NONE',  ( 15.45084971874736723, 25.40000000000000213, -47.55282581475768211 ) ) ;
#13480=CARTESIAN_POINT ( 'NONE',  ( 9.631387414534489405E-15, 48.35937500034140157, 52.43083105670540789 ) ) ;
#13481=VERTEX_POINT ( 'NONE', #13710 ) ;
#13482=CARTESIAN_POINT ( 'NONE',  ( 15.40903463028482356, 26.45937500034139589, 47.42413220539093999 ) ) ;
#13483=ORIENTED_EDGE ( 'NONE', *, *, #4203, .T. ) ;
#13484=CARTESIAN_POINT ( 'NONE',  ( -3.111920190527341144E-15, 45.50000000000000000, -50.00000000000000000 ) ) ;
#13485=CARTESIAN_POINT ( 'NONE',  ( 40.34137639590981195, 33.05937500034139731, -29.30972558990011834 ) ) ;
#13486=CARTESIAN_POINT ( 'NONE',  ( 40.45084971874737789, 40.58125000068280031, 29.38926261462365375 ) ) ;
#13492=CARTESIAN_POINT ( 'NONE',  ( 30.81806926056964002, 28.62187500034140086, 42.41743335407647209 ) ) ;
#13495=CARTESIAN_POINT ( 'NONE',  ( -15.40903463028481646, 39.52187500034139589, -47.42413220539093999 ) ) ;
#13496=SHAPE_REPRESENTATION ( 'Heavy Glass Blender Jar Body', ( #15812 ), #11844 ) ;
#13499=CARTESIAN_POINT ( 'NONE',  ( 49.86468353125001585, 44.75937500034139305, 16.20201782572375038 ) ) ;
#13500=EDGE_LOOP ( 'NONE', ( #11383, #1642, #2219, #10969 ) ) ;
#13501=CARTESIAN_POINT ( 'NONE',  ( 9.657523855033129090E-15, 24.28125000068279959, 52.57311121191334990 ) ) ;
#13505=CARTESIAN_POINT ( 'NONE',  ( 15.40903463028482356, 40.52187500034139589, 47.42413220539093999 ) ) ;
#13507=CARTESIAN_POINT ( 'NONE',  ( 2.600676159226420495E-13, 31.49999999999999289, -49.99999999999999289 ) ) ;
#13508=CARTESIAN_POINT ( 'NONE',  ( -30.81806926056963292, 23.62187500034139731, -42.41743335407647209 ) ) ;
#13516=CARTESIAN_POINT ( 'NONE',  ( -40.34137639590981195, 42.12187500034139731, 29.30972558990012189 ) ) ;
#13517=CARTESIAN_POINT ( 'NONE',  ( -40.45084971874737079, 43.98125000068279888, 29.38926261462367151 ) ) ;
#13520=B_SPLINE_CURVE_WITH_KNOTS ( 'NONE', 3,
 ( #12228, #12399, #9903, #3330 ),
 .UNSPECIFIED., .F., .F.,
 ( 4, 4 ),
 ( 0.000000000000000000, 0.01241723871866257621 ),
 .UNSPECIFIED. ) ;
#13532=CARTESIAN_POINT ( 'NONE',  ( 1.293669679204937499E-13, 37.50000000000000711, -50.00000000000000000 ) ) ;
#13538=CARTESIAN_POINT ( 'NONE',  ( -15.40903463028480580, 34.25937500034139305, 47.42413220539094709 ) ) ;
#13542=CARTESIAN_POINT ( 'NONE',  ( -15.45084971874737256, 41.38125000068279746, -47.55282581475767500 ) ) ;
#13543=CARTESIAN_POINT ( 'NONE',  ( 2.978552182361884590E-14, 47.50000000000000711, -50.00000000000000000 ) ) ;
#13552=CARTESIAN_POINT ( 'NONE',  ( 50.00000000000000711, 38.89999999999999858, 16.24598481164530739 ) ) ;
#13553=CARTESIAN_POINT ( 'NONE',  ( 1.293669679204937499E-13, 41.50000000000000000, -50.00000000000000000 ) ) ;
#13556=CARTESIAN_POINT ( 'NONE',  ( -30.90169943749473802, 30.29999999999999716, 42.53254041760200721 ) ) ;
#13564=CARTESIAN_POINT ( 'NONE',  ( 49.86468353125000164, 36.85937500034139447, -6.106662507704105588E-15 ) ) ;
#13567=CARTESIAN_POINT ( 'NONE',  ( -15.45084971874737256, 49.38125000068280457, -47.55282581475767500 ) ) ;
#13569=DIRECTION ( 'NONE',  ( -0.000000000000000000, -1.000000000000000000, -0.000000000000000000 ) ) ;
#13573=CARTESIAN_POINT ( 'NONE',  ( -49.86468353124999453, 29.82187500034139660, -16.20201782572375393 ) ) ;
#13576=CARTESIAN_POINT ( 'NONE',  ( 15.40903463028482356, 36.52187500034139589, 47.42413220539093999 ) ) ;
#13579=CARTESIAN_POINT ( 'NONE',  ( 49.86468353124999453, 44.95937500034139589, -16.20201782572376104 ) ) ;
#13581=CARTESIAN_POINT ( 'NONE',  ( 49.99999999999999289, 22.88125000068280102, -16.24598481164532160 ) ) ;
#13584=CARTESIAN_POINT ( 'NONE',  ( 49.86468353125001585, 36.82187500034140015, 16.20201782572375038 ) ) ;
#13586=CARTESIAN_POINT ( 'NONE',  ( 15.45084971874737789, 30.60000000000000142, 47.55282581475767500 ) ) ;
#13587=( BOUNDED_CURVE ( )  B_SPLINE_CURVE ( 2, ( #13507, #16179, #4808, #11198, #10938, #12518, #11276, #2283, #13755, #7451, #13586, #3378, #1108 ),
 .UNSPECIFIED., .F., .F. ) 
 B_SPLINE_CURVE_WITH_KNOTS ( ( 3, 2, 2, 2, 2, 2, 3 ),
 ( 0.6166666666666666963, 0.6199999999999999956, 0.6266666666666667052, 0.6333333333333333037, 0.6400000000000000133, 0.6466666666666666119, 0.6500000000000000222 ),
 .UNSPECIFIED. ) 
 CURVE ( )  GEOMETRIC_REPRESENTATION_ITEM ( )  RATIONAL_B_SPLINE_CURVE ( ( 0.9755282581475768211, 0.9755282581475771542, 1.000000000000000000, 0.9510565162951535312, 1.000000000000000000, 0.9510565162951535312, 1.000000000000000000, 0.9510565162951535312, 1.000000000000000000, 0.9510565162951535312, 1.000000000000000000, 0.9755282581475763770, 0.9755282581475768211 ) ) 
 REPRESENTATION_ITEM ( '' )  );
#13589=CARTESIAN_POINT ( 'NONE',  ( 9.631387414534489405E-15, 26.42187500034139447, 52.43083105670540789 ) ) ;
#13594=CARTESIAN_POINT ( 'NONE',  ( 49.86468353125000164, 38.92187500034139447, -6.106662507704105588E-15 ) ) ;
#13595=CARTESIAN_POINT ( 'NONE',  ( -15.45084971874736368, 32.18125000068279462, 47.55282581475768211 ) ) ;
#13607=DIRECTION ( 'NONE',  ( 0.000000000000000000, 1.000000000000000000, 0.000000000000000000 ) ) ;
#13610=AXIS2_PLACEMENT_3D ( 'NONE', #11987, #5066, #8250 ) ;
#13611=CARTESIAN_POINT ( 'NONE',  ( -15.45084971874737256, 33.60000000000000142, -47.55282581475767500 ) ) ;
#13613=VERTEX_POINT ( 'NONE', #10143 ) ;
#13615=CARTESIAN_POINT ( 'NONE',  ( -40.34137639590981905, 23.65937500034139518, -29.30972558990011478 ) ) ;
#13619=CARTESIAN_POINT ( 'NONE',  ( -3.219174618344376363E-15, 41.28125000068280315, -52.57311121191334990 ) ) ;
#13631=CARTESIAN_POINT ( 'NONE',  ( -40.45084971874737789, 41.80000000000000426, -29.38926261462365730 ) ) ;
#13633=DIRECTION ( 'NONE',  ( -0.000000000000000000, -1.000000000000000000, -0.000000000000000000 ) ) ;
#13634=CARTESIAN_POINT ( 'NONE',  ( -30.90169943749473802, 28.30000000000000071, 42.53254041760200721 ) ) ;
#13638=CARTESIAN_POINT ( 'NONE',  ( 15.40903463028482356, 48.45937500034140299, 47.42413220539093999 ) ) ;
#13641=VERTEX_POINT ( 'NONE', #8890 ) ;
#13643=CARTESIAN_POINT ( 'NONE',  ( -49.86468353124999453, 35.75937500034140015, -16.20201782572375393 ) ) ;
#13645=CARTESIAN_POINT ( 'NONE',  ( -6.668400408272873429E-15, 49.28125000068279604, -50.00000000000000000 ) ) ;
#13649=CARTESIAN_POINT ( 'NONE',  ( 0.000000000000000000, 193.4213562373095385, 0.000000000000000000 ) ) ;
#13657=CARTESIAN_POINT ( 'NONE',  ( 49.86468353124999453, 39.02187500034138878, -16.20201782572376459 ) ) ;
#13661=CARTESIAN_POINT ( 'NONE',  ( 30.81806926056962936, 41.15937500034139873, -42.41743335407646498 ) ) ;
#13662=ORIENTED_EDGE ( 'NONE', *, *, #7579, .F. ) ;
#13663=EDGE_CURVE ( 'NONE', #9685, #10949, #11187, .T. ) ;
#13664=CARTESIAN_POINT ( 'NONE',  ( -15.45084971874736368, 22.18125000068279817, 47.55282581475768211 ) ) ;
#13666=ADVANCED_FACE ( 'NONE', ( #3061, #4323 ), #14602, .T. ) ;
#13671=ADVANCED_FACE ( 'NONE', ( #4402 ), #5502, .T. ) ;
#13672=CARTESIAN_POINT ( 'NONE',  ( -15.40903463028481646, 23.52187500034139944, -47.42413220539093999 ) ) ;
#13676=CARTESIAN_POINT ( 'NONE',  ( -49.86468353124999453, 37.82187500034139305, -16.20201782572375393 ) ) ;
#13677=CARTESIAN_POINT ( 'NONE',  ( -40.45084971874737789, 41.58125000068280031, -29.38926261462365730 ) ) ;
#13682=CARTESIAN_POINT ( 'NONE',  ( 0.000000000000000000, 193.4213562373095385, 0.000000000000000000 ) ) ;
#13688=CARTESIAN_POINT ( 'NONE',  ( 7.919222016226809657, 25.44874571845315359, -50.00000000000000000 ) ) ;
#13691=VECTOR ( 'NONE', #15676, 1000.000000000000114 ) ;
#13697=CARTESIAN_POINT ( 'NONE',  ( -30.81806926056962226, 26.15937500034139163, 42.41743335407647919 ) ) ;
#13698=ORIENTED_EDGE ( 'NONE', *, *, #14806, .F. ) ;
#13701=CARTESIAN_POINT ( 'NONE',  ( 40.45084971874737789, 36.58125000068280031, 29.38926261462365375 ) ) ;
#13710=CARTESIAN_POINT ( 'NONE',  ( 2.978552182361884590E-14, 47.28125000068279604, -50.00000000000000000 ) ) ;
#13717=CYLINDRICAL_SURFACE ( 'NONE', #12132, 50.00000000000000000 ) ;
#13719=CARTESIAN_POINT ( 'NONE',  ( 50.00000000000000000, 29.00000000000000000, -6.123233995736766085E-15 ) ) ;
#13723=EDGE_CURVE ( 'NONE', #12134, #11385, #6627, .T. ) ;
#13725=CARTESIAN_POINT ( 'NONE',  ( -40.34137639590981905, 45.65937500034139873, -29.30972558990011478 ) ) ;
#13726=ORIENTED_EDGE ( 'NONE', *, *, #41, .F. ) ;
#13727=CARTESIAN_POINT ( 'NONE',  ( -40.34137639590981195, 26.05937500034139731, 29.30972558990012189 ) ) ;
#13731=CARTESIAN_POINT ( 'NONE',  ( 49.86468353124999453, 36.95937500034139589, -16.20201782572376459 ) ) ;
#13733=CARTESIAN_POINT ( 'NONE',  ( -3.111920190527341144E-15, 27.50000000000000000, -50.00000000000000000 ) ) ;
#13736=CARTESIAN_POINT ( 'NONE',  ( 2.978552182361884590E-14, 47.28125000068279604, -50.00000000000000000 ) ) ;
#13744=CARTESIAN_POINT ( 'NONE',  ( 15.40903463028481113, 35.32187500034139305, -47.42413220539094709 ) ) ;
#13748=CARTESIAN_POINT ( 'NONE',  ( 49.86468353125001585, 42.75937500034138594, 16.20201782572375038 ) ) ;
#13750=CARTESIAN_POINT ( 'NONE',  ( -50.00000000000000000, 21.78125000068279959, 0.000000000000000000 ) ) ;
#13755=CARTESIAN_POINT ( 'NONE',  ( 40.45084971874737789, 30.80000000000000071, 29.38926261462365375 ) ) ;
#13756=CARTESIAN_POINT ( 'NONE',  ( -30.81806926056962226, 22.22187500034139163, 42.41743335407647919 ) ) ;
#13761=CARTESIAN_POINT ( 'NONE',  ( 40.34137639590981905, 34.72187500034139873, 29.30972558990010768 ) ) ;
#13762=CARTESIAN_POINT ( 'NONE',  ( -15.45084971874736368, 42.18125000068279462, 47.55282581475768211 ) ) ;
#13767=CARTESIAN_POINT ( 'NONE',  ( -50.00000000000000000, 32.00000000000000000, 0.000000000000000000 ) ) ;
#13774=AXIS2_PLACEMENT_3D ( 'NONE', #5581, #10566, #6746 ) ;
#13777=CARTESIAN_POINT ( 'NONE',  ( -50.00000000000000000, 49.89062500034140157, 0.000000000000000000 ) ) ;
#13779=CARTESIAN_POINT ( 'NONE',  ( -15.40903463028480580, 26.25937500034140015, 47.42413220539094709 ) ) ;
#13781=ORIENTED_EDGE ( 'NONE', *, *, #4819, .T. ) ;
#13784=CARTESIAN_POINT ( 'NONE',  ( 30.90169943749475578, 38.48125000068279178, 42.53254041760200010 ) ) ;
#13785=AXIS2_PLACEMENT_3D ( 'NONE', #971, #13607, #10958 ) ;
#13786=DIRECTION ( 'NONE',  ( -0.000000000000000000, -1.000000000000000000, -0.000000000000000000 ) ) ;
#13788=CARTESIAN_POINT ( 'NONE',  ( 50.00000000000000000, 38.78125000068279604, -6.123233995736766085E-15 ) ) ;
#13800=CARTESIAN_POINT ( 'NONE',  ( 30.90169943749475578, 24.69999999999999929, 42.53254041760200010 ) ) ;
#13804=CARTESIAN_POINT ( 'NONE',  ( 15.40903463028481113, 43.25937500034139305, -47.42413220539094709 ) ) ;
#13808=CARTESIAN_POINT ( 'NONE',  ( 49.86468353124999453, 30.95937500034139944, -16.20201782572376459 ) ) ;
#13812=CARTESIAN_POINT ( 'NONE',  ( 45.74278786629302118, 25.00000000000000000, -19.85154960931340185 ) ) ;
#13813=CARTESIAN_POINT ( 'NONE',  ( 2.600676159226420495E-13, 31.28125000068279604, -49.99999999999999289 ) ) ;
#13821=CARTESIAN_POINT ( 'NONE',  ( -15.40903463028480580, 34.32187500034139305, 47.42413220539094709 ) ) ;
#13825=CARTESIAN_POINT ( 'NONE',  ( -40.34137639590981905, 37.65937500034139873, -29.30972558990011478 ) ) ;
#13827=ORIENTED_EDGE ( 'NONE', *, *, #10633, .T. ) ;
#13828=CARTESIAN_POINT ( 'NONE',  ( 50.00000000000000711, 24.68125000068279462, 16.24598481164530739 ) ) ;
#13830=CARTESIAN_POINT ( 'NONE',  ( -3.210462471511496205E-15, 25.42187500034139092, -52.43083105670540789 ) ) ;
#13834=CARTESIAN_POINT ( 'NONE',  ( 50.00000000000000711, 46.90000000000000568, 16.24598481164530739 ) ) ;
#13840=CARTESIAN_POINT ( 'NONE',  ( 49.86468353125001585, 38.82187500034140015, 16.20201782572375038 ) ) ;
#13841=CARTESIAN_POINT ( 'NONE',  ( 2.600676159226421000E-13, 33.28125000068279604, -49.99999999999999289 ) ) ;
#13844=APPLICATION_CONTEXT ( 'automotive_design' ) ;
#13857=ORIENTED_EDGE ( 'NONE', *, *, #4003, .T. ) ;
#13859=CARTESIAN_POINT ( 'NONE',  ( 49.86468353125000164, 24.85937500034139802, -6.106662507704105588E-15 ) ) ;
#13866=CARTESIAN_POINT ( 'NONE',  ( 7.919222016226758143, 38.33250428222964246, 50.00000000000000711 ) ) ;
#13867=CARTESIAN_POINT ( 'NONE',  ( -49.99999999999999289, 37.90000000000000568, -16.24598481164531449 ) ) ;
#13870=CARTESIAN_POINT ( 'NONE',  ( -3.111920190527341144E-15, 27.28125000068279604, -50.00000000000000000 ) ) ;
#13872=VECTOR ( 'NONE', #13067, 1000.000000000000000 ) ;
#13873=DIRECTION ( 'NONE',  ( 0.000000000000000000, 0.000000000000000000, -1.000000000000000000 ) ) ;
#13877=CARTESIAN_POINT ( 'NONE',  ( 49.99999999999999289, 23.10000000000000497, -16.24598481164532160 ) ) ;
#13880=( BOUNDED_CURVE ( )  B_SPLINE_CURVE ( 2, ( #13736, #5113, #12573, #16315, #12498, #1091, #11257, #4950, #7502, #177, #15218, #1420, #7672 ),
 .UNSPECIFIED., .F., .T. ) 
 B_SPLINE_CURVE_WITH_KNOTS ( ( 3, 2, 2, 2, 2, 2, 3 ),
 ( 0.08333333333333334259, 0.08666666666666666963, 0.09333333333333333759, 0.1000000000000000056, 0.1066666666666666735, 0.1133333333333333276, 0.1166666666666666685 ),
 .UNSPECIFIED. ) 
 CURVE ( )  GEOMETRIC_REPRESENTATION_ITEM ( )  RATIONAL_B_SPLINE_CURVE ( ( 0.9755282581475768211, 0.9755282581475768211, 1.000000000000000000, 0.9510565162951535312, 1.000000000000000000, 0.9510565162951535312, 1.000000000000000000, 0.9510565162951535312, 1.000000000000000000, 0.9510565162951535312, 1.000000000000000000, 0.9755282581475767101, 0.9755282581475768211 ) ) 
 REPRESENTATION_ITEM ( '' )  );
#13881=CARTESIAN_POINT ( 'NONE',  ( -30.81806926056963292, 41.55937500034139731, -42.41743335407647209 ) ) ;
#13885=CARTESIAN_POINT ( 'NONE',  ( 15.40903463028481113, 27.25937500034139660, -47.42413220539094709 ) ) ;
#13888=CARTESIAN_POINT ( 'NONE',  ( 48.35726954556789536, 24.99999999999999645, -12.16803787670825265 ) ) ;
#13889=CARTESIAN_POINT ( 'NONE',  ( 30.81806926056964002, 36.62187500034139731, 42.41743335407646498 ) ) ;
#13893=CARTESIAN_POINT ( 'NONE',  ( 15.45084971874736723, 43.39999999999999858, -47.55282581475768211 ) ) ;
#13899=CARTESIAN_POINT ( 'NONE',  ( 49.86468353124999453, 31.02187500034139234, -16.20201782572376459 ) ) ;
#13903=CARTESIAN_POINT ( 'NONE',  ( 40.34137639590981195, 37.05937500034139731, -29.30972558990011834 ) ) ;
#13906=CARTESIAN_POINT ( 'NONE',  ( 1.293669679204937499E-13, 41.50000000000000000, -50.00000000000000000 ) ) ;
#13907=CARTESIAN_POINT ( 'NONE',  ( -49.86468353125000164, 47.85937500034139447, 0.000000000000000000 ) ) ;
#13910=CARTESIAN_POINT ( 'NONE',  ( -49.86468353124999453, 21.82187500034139305, -16.20201782572375393 ) ) ;
#13913=CARTESIAN_POINT ( 'NONE',  ( -1.240322475938754499E-13, 40.50000000000000000, 50.00000000000000000 ) ) ;
#13915=CARTESIAN_POINT ( 'NONE',  ( -40.45084971874737789, 47.80000000000000426, -29.38926261462365730 ) ) ;
#13917=CARTESIAN_POINT ( 'NONE',  ( -40.34137639590981905, 47.72187500034139873, -29.30972558990011478 ) ) ;
#13924=ADVANCED_FACE ( 'NONE', ( #5979 ), #3653, .F. ) ;
#13926=CARTESIAN_POINT ( 'NONE',  ( -15.45084971874736368, 32.39999999999999858, 47.55282581475768211 ) ) ;
#13934=CARTESIAN_POINT ( 'NONE',  ( -15.45084971874736368, 40.40000000000000568, 47.55282581475768211 ) ) ;
#13937=ORIENTED_EDGE ( 'NONE', *, *, #5901, .F. ) ;
#13939=CARTESIAN_POINT ( 'NONE',  ( -40.34137639590981905, 27.65937500034139873, -29.30972558990011478 ) ) ;
#13945=EDGE_CURVE ( 'NONE', #15132, #9397, #5814, .T. ) ;
#13956=MECHANICAL_DESIGN_GEOMETRIC_PRESENTATION_REPRESENTATION('',(#11585),#1494);
#13957=FACE_OUTER_BOUND ( 'NONE', #2397, .T. ) ;
#13961=CARTESIAN_POINT ( 'NONE',  ( -49.99999999999999289, 20.09999999999999787, 16.24598481164533226 ) ) ;
#13964=CARTESIAN_POINT ( 'NONE',  ( -49.86468353124999453, 45.75937500034140015, -16.20201782572375393 ) ) ;
#13965=VERTEX_POINT ( 'NONE', #13532 ) ;
#13967=VECTOR ( 'NONE', #15944, 1000.000000000000000 ) ;
#13968=AXIS2_PLACEMENT_3D ( 'NONE', #14956, #748, #5999 ) ;
#13971=CARTESIAN_POINT ( 'NONE',  ( 30.81806926056962936, 31.15937500034139518, -42.41743335407647209 ) ) ;
#13975=CARTESIAN_POINT ( 'NONE',  ( 45.40153297753701622, 25.00000000000000000, -20.62078143446418821 ) ) ;
#13976=CARTESIAN_POINT ( 'NONE',  ( -40.34137639590981905, 35.72187500034139163, -29.30972558990011478 ) ) ;
#13977=CARTESIAN_POINT ( 'NONE',  ( 0.000000000000000000, 53.82568851450475478, 65.15972704814865324 ) ) ;
#13986=CARTESIAN_POINT ( 'NONE',  ( 9.631387414534489405E-15, 34.42187500034138736, 52.43083105670540789 ) ) ;
#13989=EDGE_LOOP ( 'NONE', ( #824, #8992, #9532, #13080 ) ) ;
#13990=CARTESIAN_POINT ( 'NONE',  ( -49.86468353124999453, 33.95937500034139589, 16.20201782572377169 ) ) ;
#13996=CARTESIAN_POINT ( 'NONE',  ( 40.45084971874737789, 20.58125000068280031, 29.38926261462365375 ) ) ;
#13998=CARTESIAN_POINT ( 'NONE',  ( 49.86468353124999453, 21.02187500034139589, -16.20201782572376459 ) ) ;
#14002=CARTESIAN_POINT ( 'NONE',  ( -15.45084971874737256, 47.60000000000000142, -47.55282581475767500 ) ) ;
#14004=CARTESIAN_POINT ( 'NONE',  ( 15.40903463028482356, 48.52187500034140299, 47.42413220539093999 ) ) ;
#14016=FILL_AREA_STYLE ('',( #3808 ) ) ;
#14022=CARTESIAN_POINT ( 'NONE',  ( -49.99999999999999289, 35.88125000068279746, 16.24598481164533226 ) ) ;
#14027=CARTESIAN_POINT ( 'NONE',  ( -15.40903463028480580, 48.32187500034140015, 47.42413220539094709 ) ) ;
#14035=CARTESIAN_POINT ( 'NONE',  ( -7.919222016226804328, 28.44874571845315003, 50.00000000000000000 ) ) ;
#14036=CARTESIAN_POINT ( 'NONE',  ( -7.919222016226752814, 37.55125428154683931, -50.00000000000000711 ) ) ;
#14038=DIRECTION ( 'NONE',  ( 0.000000000000000000, 1.000000000000000000, 0.000000000000000000 ) ) ;
#14039=CARTESIAN_POINT ( 'NONE',  ( 7.919222016226809657, 27.22999571913595318, -50.00000000000000000 ) ) ;
#14043=CARTESIAN_POINT ( 'NONE',  ( 45.11452830843730766, 25.00000000000000355, -21.24066852005663719 ) ) ;
#14045=CARTESIAN_POINT ( 'NONE',  ( 40.45084971874737789, 24.80000000000000426, 29.38926261462365375 ) ) ;
#14048=CARTESIAN_POINT ( 'NONE',  ( 49.86468353125000164, 44.85937500034140157, -6.106662507704105588E-15 ) ) ;
#14049=( GEOMETRIC_REPRESENTATION_CONTEXT ( 3 ) GLOBAL_UNCERTAINTY_ASSIGNED_CONTEXT ( ( #587 ) ) GLOBAL_UNIT_ASSIGNED_CONTEXT ( ( #11527, #7545, #47 ) ) REPRESENTATION_CONTEXT ( 'NONE', 'WORKASPACE' ) );
#14050=VERTEX_POINT ( 'NONE', #8735 ) ;
#14052=DIRECTION ( 'NONE',  ( -0.000000000000000000, -1.000000000000000000, -0.000000000000000000 ) ) ;
#14054=CARTESIAN_POINT ( 'NONE',  ( 30.81806926056962936, 27.15937500034139163, -42.41743335407647209 ) ) ;
#14058=CARTESIAN_POINT ( 'NONE',  ( 47.29342682910159112, 25.00000000000000000, -15.80652463092885007 ) ) ;
#14059=CARTESIAN_POINT ( 'NONE',  ( -15.40903463028481646, 37.52187500034139589, -47.42413220539093999 ) ) ;
#14060=CARTESIAN_POINT ( 'NONE',  ( 50.00000000000000000, 30.78125000068279959, -6.123233995736766085E-15 ) ) ;
#14064=CARTESIAN_POINT ( 'NONE',  ( -2.547328955960238000E-13, 32.50000000000000000, 49.99999999999999289 ) ) ;
#14067=CARTESIAN_POINT ( 'NONE',  ( -40.34137639590981905, 33.72187500034139873, -29.30972558990011478 ) ) ;
#14072=CARTESIAN_POINT ( 'NONE',  ( -3.210462471511496205E-15, 37.35937500034140157, -52.43083105670540789 ) ) ;
#14075=CARTESIAN_POINT ( 'NONE',  ( 30.81806926056962936, 49.15937500034138452, -42.41743335407647209 ) ) ;
#14077=CARTESIAN_POINT ( 'NONE',  ( -30.81806926056962226, 26.22187500034139518, 42.41743335407647919 ) ) ;
#14081=CARTESIAN_POINT ( 'NONE',  ( -50.00000000000000000, 48.00000000000000000, 0.000000000000000000 ) ) ;
#14086=EDGE_CURVE ( 'NONE', #1062, #14577, #10153, .T. ) ;
#14087=FACE_OUTER_BOUND ( 'NONE', #3137, .T. ) ;
#14089=CARTESIAN_POINT ( 'NONE',  ( -49.99999999999999289, 37.88125000068279746, 16.24598481164533226 ) ) ;
#14090=ORIENTED_EDGE ( 'NONE', *, *, #8648, .F. ) ;
#14094=CARTESIAN_POINT ( 'NONE',  ( -15.40903463028480580, 48.32187500034140015, 47.42413220539094709 ) ) ;
#14104=CARTESIAN_POINT ( 'NONE',  ( -49.86468353124999453, 48.02187500034139589, 16.20201782572377525 ) ) ;
#14106=CARTESIAN_POINT ( 'NONE',  ( -40.45084971874737079, 26.20000000000000284, 29.38926261462367151 ) ) ;
#14111=CARTESIAN_POINT ( 'NONE',  ( -49.86468353125000164, 49.89062500034140157, 0.000000000000000000 ) ) ;
#14112=CARTESIAN_POINT ( 'NONE',  ( 8.446640517145639571E-15, 28.49999999999999645, 50.00000000000000000 ) ) ;
#14123=CARTESIAN_POINT ( 'NONE',  ( 40.45084971874737079, 25.19999999999999929, -29.38926261462366440 ) ) ;
#14125=ORIENTED_EDGE ( 'NONE', *, *, #16428, .T. ) ;
#14126=CARTESIAN_POINT ( 'NONE',  ( 15.40903463028482356, 40.45937500034139589, 47.42413220539093999 ) ) ;
#14131=CARTESIAN_POINT ( 'NONE',  ( -49.86468353125000164, 29.85937500034139802, 0.000000000000000000 ) ) ;
#14135=CARTESIAN_POINT ( 'NONE',  ( 49.99999999999999289, 27.10000000000000142, -16.24598481164532160 ) ) ;
#14137=LINE ( 'NONE', #4263, #13872 ) ;
#14138=CARTESIAN_POINT ( 'NONE',  ( 15.40903463028481113, 35.32187500034139305, -47.42413220539094709 ) ) ;
#14147=CARTESIAN_POINT ( 'NONE',  ( -49.86468353124999453, 30.02187500034139234, 16.20201782572377525 ) ) ;
#14150=CARTESIAN_POINT ( 'NONE',  ( -15.40903463028480580, 38.25937500034140015, 47.42413220539094709 ) ) ;
#14155=CARTESIAN_POINT ( 'NONE',  ( 49.99999999999999289, 20.88125000068279746, -16.24598481164532160 ) ) ;
#14158=CARTESIAN_POINT ( 'NONE',  ( 49.86468353125000164, 24.92187500034139802, -6.106662507704105588E-15 ) ) ;
#14164=CARTESIAN_POINT ( 'NONE',  ( -15.45084971874736368, 48.40000000000000568, 47.55282581475768211 ) ) ;
#14170=CARTESIAN_POINT ( 'NONE',  ( 9.657523855033129090E-15, 40.28125000068278894, 52.57311121191334990 ) ) ;
#14176=CARTESIAN_POINT ( 'NONE',  ( -15.40903463028481646, 47.52187500034139589, -47.42413220539093999 ) ) ;
#14183=FACE_OUTER_BOUND ( 'NONE', #9460, .T. ) ;
#14187=CARTESIAN_POINT ( 'NONE',  ( 15.40903463028481113, 21.25937500034139660, -47.42413220539094709 ) ) ;
#14190=ORIENTED_EDGE ( 'NONE', *, *, #10992, .F. ) ;
#14192=VECTOR ( 'NONE', #14888, 1000.000000000000000 ) ;
#14195=CARTESIAN_POINT ( 'NONE',  ( -50.00000000000000000, 28.00000000000000000, 0.000000000000000000 ) ) ;
#14199=FACE_BOUND ( 'NONE', #2523, .T. ) ;
#14207=CARTESIAN_POINT ( 'NONE',  ( 30.81806926056964002, 38.55937500034140442, 42.41743335407647209 ) ) ;
#14212=CARTESIAN_POINT ( 'NONE',  ( -49.86468353124999453, 23.95937500034138878, 16.20201782572377525 ) ) ;
#14218=CARTESIAN_POINT ( 'NONE',  ( 30.81806926056964002, 26.62187500034139731, 42.41743335407646498 ) ) ;
#14230=CARTESIAN_POINT ( 'NONE',  ( 15.40903463028481113, 27.32187500034139660, -47.42413220539094709 ) ) ;
#14234=EDGE_CURVE ( 'NONE', #15357, #436, #12803, .T. ) ;
#14237=CARTESIAN_POINT ( 'NONE',  ( 49.86468353125000164, 32.85937500034139447, -6.106662507704105588E-15 ) ) ;
#14240=CARTESIAN_POINT ( 'NONE',  ( -49.86468353124999453, 49.75937500034138594, -16.20201782572375393 ) ) ;
#14241=ADVANCED_FACE ( 'NONE', ( #1737 ), #9319, .F. ) ;
#14245=AXIS2_PLACEMENT_3D ( 'NONE', #1889, #8142, #13124 ) ;
#14251=CARTESIAN_POINT ( 'NONE',  ( -49.99999999999999289, 40.09999999999999432, 16.24598481164533226 ) ) ;
#14253=CARTESIAN_POINT ( 'NONE',  ( -3.210462471511496205E-15, 45.42187500034139447, -52.43083105670540789 ) ) ;
#14258=CARTESIAN_POINT ( 'NONE',  ( 15.45084971874736723, 35.18125000068280173, -47.55282581475768211 ) ) ;
#14263=CARTESIAN_POINT ( 'NONE',  ( 40.34137639590981905, 46.72187500034139873, 29.30972558990010768 ) ) ;
#14272=CARTESIAN_POINT ( 'NONE',  ( -15.40903463028481646, 45.52187500034139589, -47.42413220539093999 ) ) ;
#14278=EDGE_LOOP ( 'NONE', ( #5720, #565, #11889, #1739, #670, #6970, #2608, #8680, #8388, #3778, #1588, #13662, #13392, #12898, #14907, #15271, #4444, #11369, #775, #16206, #14190, #23, #13698, #5786, #5482, #15683, #14412, #13483, #3365 ) ) ;
#14281=FACE_OUTER_BOUND ( 'NONE', #12813, .T. ) ;
#14284=CARTESIAN_POINT ( 'NONE',  ( 40.45084971874737079, 48.98125000068279888, -29.38926261462366440 ) ) ;
#14286=CARTESIAN_POINT ( 'NONE',  ( 2.600676159226420495E-13, 33.28125000068279604, -49.99999999999999289 ) ) ;
#14288=FACE_BOUND ( 'NONE', #13100, .T. ) ;
#14290=CARTESIAN_POINT ( 'NONE',  ( -50.00000000000000000, 37.78125000068280315, 0.000000000000000000 ) ) ;
#14294=CARTESIAN_POINT ( 'NONE',  ( 15.40903463028482356, 36.45937500034139589, 47.42413220539093999 ) ) ;
#14296=VERTEX_POINT ( 'NONE', #486 ) ;
#14297=CARTESIAN_POINT ( 'NONE',  ( 30.90169943749474157, 47.08125000068280031, -42.53254041760200721 ) ) ;
#14300=CARTESIAN_POINT ( 'NONE',  ( 40.34137639590981195, 21.05937500034139376, -29.30972558990011834 ) ) ;
#14303=CARTESIAN_POINT ( 'NONE',  ( -2.547328955960238000E-13, 34.50000000000000000, 49.99999999999999289 ) ) ;
#14305=CARTESIAN_POINT ( 'NONE',  ( 49.86468353124999453, 31.02187500034139589, -16.20201782572376104 ) ) ;
#14314=CARTESIAN_POINT ( 'NONE',  ( -40.45084971874737079, 34.20000000000000284, 29.38926261462367151 ) ) ;
#14318=CARTESIAN_POINT ( 'NONE',  ( -49.86468353125000164, 27.85937500034139447, 0.000000000000000000 ) ) ;
#14322=CARTESIAN_POINT ( 'NONE',  ( -3.210462471511496205E-15, 41.35937500034138736, -52.43083105670540789 ) ) ;
#14326=CARTESIAN_POINT ( 'NONE',  ( 40.34137639590981905, 20.72187500034139873, 29.30972558990010768 ) ) ;
#14331=CARTESIAN_POINT ( 'NONE',  ( -30.90169943749474868, 43.70000000000000284, -42.53254041760200721 ) ) ;
#14333=CARTESIAN_POINT ( 'NONE',  ( -30.81806926056962226, 44.22187500034139163, 42.41743335407647919 ) ) ;
#14336=CARTESIAN_POINT ( 'NONE',  ( 40.34137639590981905, 46.65937500034139873, 29.30972558990010768 ) ) ;
#14338=CARTESIAN_POINT ( 'NONE',  ( -15.45084971874736368, 28.18125000068279817, 47.55282581475768211 ) ) ;
#14342=DIRECTION ( 'NONE',  ( -0.000000000000000000, -1.000000000000000000, -0.000000000000000000 ) ) ;
#14345=CARTESIAN_POINT ( 'NONE',  ( 40.34137639590981905, 44.72187500034139163, 29.30972558990010768 ) ) ;
#14350=CARTESIAN_POINT ( 'NONE',  ( 30.90169943749475223, 34.48125000068279888, 42.53254041760199300 ) ) ;
#14354=CARTESIAN_POINT ( 'NONE',  ( 9.631387414534489405E-15, 20.35937500034139092, 52.43083105670540789 ) ) ;
#14359=DIRECTION ( 'NONE',  ( -0.000000000000000000, -1.000000000000000000, -0.000000000000000000 ) ) ;
#14360=DIRECTION ( 'NONE',  ( 1.067350013832299517E-17, 0.9961946980917455452, -0.08715574274765836016 ) ) ;
#14370=CARTESIAN_POINT ( 'NONE',  ( 0.000000000000000000, 272.0000000000000000, 0.000000000000000000 ) ) ;
#14372=CARTESIAN_POINT ( 'NONE',  ( 40.34137639590981195, 35.05937500034139731, -29.30972558990011834 ) ) ;
#14377=CARTESIAN_POINT ( 'NONE',  ( -40.34137639590981905, 21.65937500034139518, -29.30972558990011478 ) ) ;
#14381=CARTESIAN_POINT ( 'NONE',  ( 50.00000000000000000, 25.00000000000000000, -6.123233995736766085E-15 ) ) ;
#14382=CARTESIAN_POINT ( 'NONE',  ( -49.86468353124999453, 25.82187500034139305, -16.20201782572375393 ) ) ;
#14388=CARTESIAN_POINT ( 'NONE',  ( 30.90169943749474157, 35.30000000000000426, -42.53254041760200721 ) ) ;
#14393=CARTESIAN_POINT ( 'NONE',  ( -30.81806926056963292, 29.55937500034139376, -42.41743335407646498 ) ) ;
#14396=CARTESIAN_POINT ( 'NONE',  ( -30.81806926056963292, 39.55937500034139731, -42.41743335407647209 ) ) ;
#14402=CARTESIAN_POINT ( 'NONE',  ( -15.45084971874737256, 39.60000000000000142, -47.55282581475767500 ) ) ;
#14405=CARTESIAN_POINT ( 'NONE',  ( -30.81806926056962226, 42.22187500034139163, 42.41743335407647919 ) ) ;
#14407=( BOUNDED_CURVE ( )  B_SPLINE_CURVE ( 2, ( #1158, #8815, #12313, #6011, #914, #5024, #8493, #3756, #4775, #9913, #4939, #7338, #11323 ),
 .UNSPECIFIED., .F., .F. ) 
 B_SPLINE_CURVE_WITH_KNOTS ( ( 3, 2, 2, 2, 2, 2, 3 ),
 ( 0.1833333333333333481, 0.1866666666666666752, 0.1933333333333333293, 0.2000000000000000111, 0.2066666666666666652, 0.2133333333333333470, 0.2166666666666666741 ),
 .UNSPECIFIED. ) 
 CURVE ( )  GEOMETRIC_REPRESENTATION_ITEM ( )  RATIONAL_B_SPLINE_CURVE ( ( 0.9755282581475767101, 0.9755282581475768211, 1.000000000000000000, 0.9510565162951535312, 1.000000000000000000, 0.9510565162951535312, 1.000000000000000000, 0.9510565162951535312, 1.000000000000000000, 0.9510565162951535312, 1.000000000000000000, 0.9755282581475768211, 0.9755282581475768211 ) ) 
 REPRESENTATION_ITEM ( '' )  );
#14410=CARTESIAN_POINT ( 'NONE',  ( -49.99999999999999289, 29.88125000068279391, 16.24598481164533226 ) ) ;
#14412=ORIENTED_EDGE ( 'NONE', *, *, #10165, .F. ) ;
#14415=EDGE_CURVE ( 'NONE', #13965, #1001, #5458, .T. ) ;
#14417=CARTESIAN_POINT ( 'NONE',  ( -30.81806926056962226, 44.22187500034139163, 42.41743335407647209 ) ) ;
#14419=CARTESIAN_POINT ( 'NONE',  ( -7.919222016226870942, 40.22999571913594963, 49.99999999999997158 ) ) ;
#14427=CARTESIAN_POINT ( 'NONE',  ( 49.86468353125000164, 42.92187500034140157, -6.106662507704105588E-15 ) ) ;
#14433=DIRECTION ( 'NONE',  ( 0.000000000000000000, 1.000000000000000000, 0.000000000000000000 ) ) ;
#14439=CARTESIAN_POINT ( 'NONE',  ( 30.90169943749475223, 48.69999999999999574, 42.53254041760199300 ) ) ;
#14445=AXIS2_PLACEMENT_3D ( 'NONE', #4505, #15882, #16209 ) ;
#14446=CARTESIAN_POINT ( 'NONE',  ( 15.40903463028482356, 34.45937500034139589, 47.42413220539093999 ) ) ;
#14449=CARTESIAN_POINT ( 'NONE',  ( 40.45084971874737079, 48.98125000068279888, -29.38926261462366440 ) ) ;
#14451=CARTESIAN_POINT ( 'NONE',  ( 40.34137639590981905, 20.65937500034139873, 29.30972558990010768 ) ) ;
#14455=CARTESIAN_POINT ( 'NONE',  ( 46.00570371104048206, 25.06239642599078365, -21.51344788172325195 ) ) ;
#14461=CARTESIAN_POINT ( 'NONE',  ( -50.00000000000000000, 34.00000000000000000, 0.000000000000000000 ) ) ;
#14466=CARTESIAN_POINT ( 'NONE',  ( -30.81806926056962226, 30.15937500034139163, 42.41743335407647209 ) ) ;
#14468=VERTEX_POINT ( 'NONE', #14606 ) ;
#14471=CARTESIAN_POINT ( 'NONE',  ( -30.81806926056962226, 40.15937500034139163, 42.41743335407647919 ) ) ;
#14481=CARTESIAN_POINT ( 'NONE',  ( 9.631387414534489405E-15, 32.42187500034139447, 52.43083105670540789 ) ) ;
#14482=AXIS2_PLACEMENT_3D ( 'NONE', #10514, #1844, #10838 ) ;
#14483=CARTESIAN_POINT ( 'NONE',  ( 40.45084971874737789, 42.80000000000000426, 29.38926261462365375 ) ) ;
#14485=CARTESIAN_POINT ( 'NONE',  ( 30.81806926056964002, 42.62187500034139731, 42.41743335407647209 ) ) ;
#14489=CARTESIAN_POINT ( 'NONE',  ( -30.81806926056963292, 49.55937500034139731, -42.41743335407646498 ) ) ;
#14495=CARTESIAN_POINT ( 'NONE',  ( 49.99999999999999289, 32.88125000068280457, -16.24598481164532160 ) ) ;
#14499=CARTESIAN_POINT ( 'NONE',  ( 30.81806926056964002, 38.62187500034139020, 42.41743335407646498 ) ) ;
#14512=CARTESIAN_POINT ( 'NONE',  ( -40.34137639590981905, 43.72187500034139873, -29.30972558990011478 ) ) ;
#14515=EDGE_CURVE ( 'NONE', #12805, #5870, #12334, .T. ) ;
#14516=DIRECTION ( 'NONE',  ( 0.000000000000000000, 0.000000000000000000, 1.000000000000000000 ) ) ;
#14523=CARTESIAN_POINT ( 'NONE',  ( -7.919222016226934890, 34.22999571913595673, 49.99999999999996447 ) ) ;
#14524=CONICAL_SURFACE ( 'NONE', #15596, 62.01141590572476758, 0.08726646259971666819 ) ;
#14532=CARTESIAN_POINT ( 'NONE',  ( -15.40903463028481646, 31.45937500034139944, -47.42413220539093999 ) ) ;
#14535=ORIENTED_EDGE ( 'NONE', *, *, #9912, .T. ) ;
#14536=CARTESIAN_POINT ( 'NONE',  ( -40.45084971874737789, 47.58125000068280031, -29.38926261462365730 ) ) ;
#14538=CARTESIAN_POINT ( 'NONE',  ( 40.34137639590981195, 25.05937500034139376, -29.30972558990011834 ) ) ;
#14540=CARTESIAN_POINT ( 'NONE',  ( -49.99999999999999289, 48.09999999999999432, 16.24598481164533226 ) ) ;
#14543=CARTESIAN_POINT ( 'NONE',  ( -15.40903463028480580, 26.32187500034140015, 47.42413220539094709 ) ) ;
#14550=CARTESIAN_POINT ( 'NONE',  ( -49.99999999999999289, 32.10000000000000142, 16.24598481164533226 ) ) ;
#14557=CARTESIAN_POINT ( 'NONE',  ( -15.40903463028481646, 31.45937500034139944, -47.42413220539093999 ) ) ;
#14560=CARTESIAN_POINT ( 'NONE',  ( 49.86468353125000164, 38.85937500034139447, -6.106662507704105588E-15 ) ) ;
#14562=DIRECTION ( 'NONE',  ( 0.000000000000000000, -0.000000000000000000, 1.000000000000000000 ) ) ;
#14567=CARTESIAN_POINT ( 'NONE',  ( 49.86468353124999453, 33.02187500034139589, -16.20201782572376459 ) ) ;
#14568=CARTESIAN_POINT ( 'NONE',  ( 50.00000000000000000, 41.00000000000000000, -6.123233995736766085E-15 ) ) ;
#14570=CARTESIAN_POINT ( 'NONE',  ( 15.40903463028481113, 41.32187500034140015, -47.42413220539094709 ) ) ;
#14573=CYLINDRICAL_SURFACE ( 'NONE', #3315, 50.00000000000000000 ) ;
#14576=CARTESIAN_POINT ( 'NONE',  ( 40.45084971874737789, 28.58125000068280031, 29.38926261462365375 ) ) ;
#14577=VERTEX_POINT ( 'NONE', #14941 ) ;
#14578=CARTESIAN_POINT ( 'NONE',  ( 7.919222016226693306, 32.33250428222964246, 50.00000000000003553 ) ) ;
#14579=CARTESIAN_POINT ( 'NONE',  ( -40.34137639590981905, 37.72187500034139873, -29.30972558990011478 ) ) ;
#14582=EDGE_CURVE ( 'NONE', #3234, #13411, #8621, .T. ) ;
#14588=CARTESIAN_POINT ( 'NONE',  ( 49.86468353124999453, 43.02187500034138878, -16.20201782572376459 ) ) ;
#14592=ORIENTED_EDGE ( 'NONE', *, *, #4336, .T. ) ;
#14602=PLANE ( 'NONE',  #4702 ) ;
#14605=CARTESIAN_POINT ( 'NONE',  ( 2.600676159226420495E-13, 33.49999999999999289, -49.99999999999999289 ) ) ;
#14606=CARTESIAN_POINT ( 'NONE',  ( 1.293669679204937499E-13, 37.28125000068280315, -50.00000000000000000 ) ) ;
#14609=CARTESIAN_POINT ( 'NONE',  ( 15.40903463028481113, 29.25937500034139660, -47.42413220539094709 ) ) ;
#14611=ORIENTED_EDGE ( 'NONE', *, *, #3039, .F. ) ;
#14613=CARTESIAN_POINT ( 'NONE',  ( 30.90169943749474157, 45.08125000068279320, -42.53254041760200721 ) ) ;
#14614=CARTESIAN_POINT ( 'NONE',  ( 7.919222016226827421, 47.44874571845315359, -50.00000000000000000 ) ) ;
#14617=CARTESIAN_POINT ( 'NONE',  ( -30.90169943749474513, 27.48125000068279888, -42.53254041760200721 ) ) ;
#14629=CARTESIAN_POINT ( 'NONE',  ( -15.45084971874736368, 36.39999999999999858, 47.55282581475768211 ) ) ;
#14631=EDGE_CURVE ( 'NONE', #5127, #1863, #10646, .T. ) ;
#14632=CARTESIAN_POINT ( 'NONE',  ( -30.81806926056962226, 48.15937500034139873, 42.41743335407647919 ) ) ;
#14638=CARTESIAN_POINT ( 'NONE',  ( -40.34137639590981905, 39.65937500034139873, -29.30972558990011478 ) ) ;
#14644=CARTESIAN_POINT ( 'NONE',  ( -15.40903463028481646, 31.52187500034139944, -47.42413220539093999 ) ) ;
#14647=CARTESIAN_POINT ( 'NONE',  ( 30.81806926056962936, 39.22187500034139873, -42.41743335407647209 ) ) ;
#14650=EDGE_LOOP ( 'NONE', ( #5051, #4295, #2248, #15859 ) ) ;
#14651=CARTESIAN_POINT ( 'NONE',  ( -49.86468353124999453, 47.95937500034138878, 16.20201782572377169 ) ) ;
#14654=CARTESIAN_POINT ( 'NONE',  ( -49.99999999999999289, 31.88125000068280102, 16.24598481164533226 ) ) ;
#14658=CARTESIAN_POINT ( 'NONE',  ( -3.210462471511496205E-15, 39.42187500034139447, -52.43083105670540789 ) ) ;
#14661=CARTESIAN_POINT ( 'NONE',  ( -3.210462471511496205E-15, 25.42187500034139092, -52.43083105670540789 ) ) ;
#14667=CARTESIAN_POINT ( 'NONE',  ( -15.40903463028480580, 44.32187500034140015, 47.42413220539094709 ) ) ;
#14676=CARTESIAN_POINT ( 'NONE',  ( -7.919222016226818539, 49.55125428154685352, -49.99999999999999289 ) ) ;
#14686=CARTESIAN_POINT ( 'NONE',  ( -1.240322475938754499E-13, 36.50000000000000711, 50.00000000000000000 ) ) ;
#14689=CARTESIAN_POINT ( 'NONE',  ( -15.40903463028480580, 32.25937500034140015, 47.42413220539094709 ) ) ;
#14695=CARTESIAN_POINT ( 'NONE',  ( 49.99999999999999289, 44.88125000068279036, -16.24598481164532160 ) ) ;
#14696=CARTESIAN_POINT ( 'NONE',  ( 30.90169943749473802, 47.29999999999999716, -42.53254041760200721 ) ) ;
#14703=CARTESIAN_POINT ( 'NONE',  ( -1.240322475938754499E-13, 38.50000000000000711, 50.00000000000000000 ) ) ;
#14707=CARTESIAN_POINT ( 'NONE',  ( -30.90169943749474868, 25.69999999999999929, -42.53254041760200721 ) ) ;
#14709=CARTESIAN_POINT ( 'NONE',  ( -3.210462471511496205E-15, 49.35937500034138736, -52.43083105670540789 ) ) ;
#14716=CARTESIAN_POINT ( 'NONE',  ( 49.86468353124999453, 34.95937500034138878, -16.20201782572376459 ) ) ;
#14717=CIRCLE ( 'NONE', #8898, 42.00000000000000711 ) ;
#14721=CYLINDRICAL_SURFACE ( 'NONE', #5497, 50.00000000000000000 ) ;
#14725=CARTESIAN_POINT ( 'NONE',  ( -49.86468353125000164, 27.92187500034139447, 0.000000000000000000 ) ) ;
#14729=CARTESIAN_POINT ( 'NONE',  ( -40.34137639590981905, 35.72187500034139163, -29.30972558990011478 ) ) ;
#14734=CARTESIAN_POINT ( 'NONE',  ( -40.34137639590981905, 39.65937500034139873, -29.30972558990011478 ) ) ;
#14736=CARTESIAN_POINT ( 'NONE',  ( -15.45084971874737256, 25.38125000068279746, -47.55282581475767500 ) ) ;
#14741=CARTESIAN_POINT ( 'NONE',  ( -30.81806926056963292, 43.62187500034139020, -42.41743335407646498 ) ) ;
#14746=CARTESIAN_POINT ( 'NONE',  ( -15.40903463028481646, 21.52187500034139589, -47.42413220539093999 ) ) ;
#14757=CARTESIAN_POINT ( 'NONE',  ( 40.34137639590981195, 43.12187500034139731, -29.30972558990011834 ) ) ;
#14776=CARTESIAN_POINT ( 'NONE',  ( 49.86468353125001585, 30.75937500034139305, 16.20201782572375038 ) ) ;
#14781=CARTESIAN_POINT ( 'NONE',  ( 9.657523855033129090E-15, 44.28125000068280315, 52.57311121191334990 ) ) ;
#14782=CARTESIAN_POINT ( 'NONE',  ( 40.45084971874737079, 47.20000000000000284, -29.38926261462366440 ) ) ;
#14786=FACE_OUTER_BOUND ( 'NONE', #1721, .T. ) ;
#14792=CARTESIAN_POINT ( 'NONE',  ( 30.90169943749473802, 39.30000000000000426, -42.53254041760200721 ) ) ;
#14793=CARTESIAN_POINT ( 'NONE',  ( -7.919222016226752814, 41.55125428154683931, -50.00000000000000711 ) ) ;
#14796=CARTESIAN_POINT ( 'NONE',  ( -40.45084971874737789, 29.80000000000000071, -29.38926261462365730 ) ) ;
#14805=CARTESIAN_POINT ( 'NONE',  ( 49.86468353125001585, 34.75937500034139305, 16.20201782572375038 ) ) ;
#14806=EDGE_CURVE ( 'NONE', #15793, #15674, #3840, .T. ) ;
#14810=DIRECTION ( 'NONE',  ( 0.000000000000000000, 0.9961946980917455452, 0.08715574274765836016 ) ) ;
#14815=CARTESIAN_POINT ( 'NONE',  ( -49.86468353124999453, 31.82187500034139305, -16.20201782572375393 ) ) ;
#14816=CARTESIAN_POINT ( 'NONE',  ( 7.919222016226940219, 33.44874571845316069, -49.99999999999996447 ) ) ;
#14818=CARTESIAN_POINT ( 'NONE',  ( 49.86468353125001585, 36.82187500034140015, 16.20201782572375038 ) ) ;
#14822=ORIENTED_EDGE ( 'NONE', *, *, #5901, .T. ) ;
#14823=CARTESIAN_POINT ( 'NONE',  ( -30.81806926056962226, 42.15937500034139163, 42.41743335407647209 ) ) ;
#14825=CARTESIAN_POINT ( 'NONE',  ( -30.90169943749473802, 26.08125000068279320, 42.53254041760200721 ) ) ;
#14829=CARTESIAN_POINT ( 'NONE',  ( -49.86468353124999453, 41.82187500034140015, -16.20201782572375393 ) ) ;
#14831=CARTESIAN_POINT ( 'NONE',  ( 50.00000000000000711, 40.89999999999999858, 16.24598481164530739 ) ) ;
#14833=CARTESIAN_POINT ( 'NONE',  ( 40.34137639590981905, 26.72187500034139518, 29.30972558990010768 ) ) ;
#14837=CARTESIAN_POINT ( 'NONE',  ( 0.000000000000000000, 52.00000000000000711, -42.00000000000000711 ) ) ;
#14839=CARTESIAN_POINT ( 'NONE',  ( -30.81806926056963292, 35.62187500034140442, -42.41743335407647209 ) ) ;
#14841=CARTESIAN_POINT ( 'NONE',  ( -49.99999999999999289, 43.88125000068279746, 16.24598481164533226 ) ) ;
#14854=CARTESIAN_POINT ( 'NONE',  ( -50.00000000000000000, 30.00000000000000355, 0.000000000000000000 ) ) ;
#14859=CARTESIAN_POINT ( 'NONE',  ( -49.99999999999999289, 33.89999999999999147, -16.24598481164531449 ) ) ;
#14861=CARTESIAN_POINT ( 'NONE',  ( -30.81806926056962226, 22.15937500034139873, 42.41743335407647919 ) ) ;
#14862=ORIENTED_EDGE ( 'NONE', *, *, #7428, .T. ) ;
#14866=CARTESIAN_POINT ( 'NONE',  ( 50.00000000000000711, 42.68125000068280173, 16.24598481164530739 ) ) ;
#14874=DIRECTION ( 'NONE',  ( -0.000000000000000000, -1.000000000000000000, -0.000000000000000000 ) ) ;
#14881=CARTESIAN_POINT ( 'NONE',  ( 30.90169943749475578, 30.70000000000000284, 42.53254041760200010 ) ) ;
#14888=DIRECTION ( 'NONE',  ( -0.000000000000000000, -1.000000000000000000, -0.000000000000000000 ) ) ;
#14891=CARTESIAN_POINT ( 'NONE',  ( -30.81806926056963292, 35.55937500034139020, -42.41743335407647209 ) ) ;
#14903=CARTESIAN_POINT ( 'NONE',  ( 49.86468353125000164, 36.92187500034140157, -6.106662507704105588E-15 ) ) ;
#14905=VERTEX_POINT ( 'NONE', #14837 ) ;
#14906=CARTESIAN_POINT ( 'NONE',  ( 30.81806926056964002, 44.55937500034139020, 42.41743335407646498 ) ) ;
#14907=ORIENTED_EDGE ( 'NONE', *, *, #1297, .F. ) ;
#14908=CARTESIAN_POINT ( 'NONE',  ( 40.45084971874737079, 24.98125000068279888, -29.38926261462366440 ) ) ;
#14914=CARTESIAN_POINT ( 'NONE',  ( -15.40903463028480580, 24.32187500034139660, 47.42413220539094709 ) ) ;
#14917=CARTESIAN_POINT ( 'NONE',  ( 6.123233995736766085E-15, 193.4213562373095385, 50.00000000000000000 ) ) ;
#14919=CARTESIAN_POINT ( 'NONE',  ( 15.40903463028481113, 35.32187500034139305, -47.42413220539094709 ) ) ;
#14920=CARTESIAN_POINT ( 'NONE',  ( -40.45084971874737079, 31.98125000068280244, 29.38926261462367151 ) ) ;
#14923=EDGE_CURVE ( 'NONE', #14296, #1767, #2118, .T. ) ;
#14934=EDGE_CURVE ( 'NONE', #7759, #16058, #15090, .T. ) ;
#14941=CARTESIAN_POINT ( 'NONE',  ( 5.755839955992560641E-15, 25.00000000000000000, 47.00000000000000000 ) ) ;
#14942=VERTEX_POINT ( 'NONE', #511 ) ;
#14943=CARTESIAN_POINT ( 'NONE',  ( -40.34137639590981905, 21.65937500034139518, -29.30972558990011478 ) ) ;
#14948=CARTESIAN_POINT ( 'NONE',  ( 30.90169943749474157, 41.08125000068280031, -42.53254041760200721 ) ) ;
#14956=CARTESIAN_POINT ( 'NONE',  ( 0.000000000000000000, 52.00000000000000711, 0.000000000000000000 ) ) ;
#14964=CARTESIAN_POINT ( 'NONE',  ( -49.99999999999999289, 29.89999999999999858, -16.24598481164531449 ) ) ;
#14965=CARTESIAN_POINT ( 'NONE',  ( 5.755839955992560641E-15, 193.4213562373095385, 47.00000000000000000 ) ) ;
#14967=CIRCLE ( 'NONE', #1711, 47.00000000000000000 ) ;
#14968=CARTESIAN_POINT ( 'NONE',  ( 49.86468353125001585, 42.75937500034138594, 16.20201782572375038 ) ) ;
#14973=CARTESIAN_POINT ( 'NONE',  ( -40.34137639590981905, 35.65937500034139873, -29.30972558990011478 ) ) ;
#14974=FACE_OUTER_BOUND ( 'NONE', #10868, .T. ) ;
#14978=CYLINDRICAL_SURFACE ( 'NONE', #4701, 50.00000000000000000 ) ;
#14985=CARTESIAN_POINT ( 'NONE',  ( -30.81806926056962226, 38.22187500034139873, 42.41743335407647919 ) ) ;
#14989=VECTOR ( 'NONE', #14052, 1000.000000000000000 ) ;
#14990=CARTESIAN_POINT ( 'NONE',  ( -49.86468353124999453, 45.75937500034140015, -16.20201782572375393 ) ) ;
#14992=CARTESIAN_POINT ( 'NONE',  ( -40.45084971874737079, 23.98125000068279888, 29.38926261462367151 ) ) ;
#14993=CARTESIAN_POINT ( 'NONE',  ( -2.547328955960238000E-13, 34.50000000000000000, 49.99999999999999289 ) ) ;
#14996=CARTESIAN_POINT ( 'NONE',  ( 15.45084971874737789, 40.60000000000000142, 47.55282581475767500 ) ) ;
#14998=CARTESIAN_POINT ( 'NONE',  ( 49.86468353125001585, 26.82187500034138949, 16.20201782572375038 ) ) ;
#15003=CARTESIAN_POINT ( 'NONE',  ( -15.40903463028480580, 36.32187500034140015, 47.42413220539094709 ) ) ;
#15004=CARTESIAN_POINT ( 'NONE',  ( -50.00000000000000000, 41.78125000068280315, 0.000000000000000000 ) ) ;
#15019=AXIS2_PLACEMENT_3D ( 'NONE', #8043, #13114, #1720 ) ;
#15024=CARTESIAN_POINT ( 'NONE',  ( 0.000000000000000000, 193.4213562373095385, 0.000000000000000000 ) ) ;
#15027=CARTESIAN_POINT ( 'NONE',  ( 40.34137639590981195, 25.05937500034139376, -29.30972558990011834 ) ) ;
#15030=ORIENTED_EDGE ( 'NONE', *, *, #10990, .T. ) ;
#15032=CARTESIAN_POINT ( 'NONE',  ( 30.90169943749474157, 35.08125000068278609, -42.53254041760200721 ) ) ;
#15034=LINE ( 'NONE', #9976, #6566 ) ;
#15035=CARTESIAN_POINT ( 'NONE',  ( 0.000000000000000000, 272.0000000000000000, -79.49773270518484480 ) ) ;
#15039=DIRECTION ( 'NONE',  ( 1.000000000000000000, 0.000000000000000000, 0.000000000000000000 ) ) ;
#15042=CYLINDRICAL_SURFACE ( 'NONE', #5427, 82.49773270518484480 ) ;
#15049=CARTESIAN_POINT ( 'NONE',  ( 49.99999999999999289, 31.09999999999999787, -16.24598481164532160 ) ) ;
#15054=( BOUNDED_CURVE ( )  B_SPLINE_CURVE ( 2, ( #13188, #8199, #7952, #9534, #1707, #10449, #1626, #13265, #15751, #1792, #4467, #14578, #6720 ),
 .UNSPECIFIED., .F., .T. ) 
 B_SPLINE_CURVE_WITH_KNOTS ( ( 3, 2, 2, 2, 2, 2, 3 ),
 ( 0.5500000000000000444, 0.5533333333333333437, 0.5600000000000000533, 0.5666666666666666519, 0.5733333333333333615, 0.5799999999999999600, 0.5833333333333333703 ),
 .UNSPECIFIED. ) 
 CURVE ( )  GEOMETRIC_REPRESENTATION_ITEM ( )  RATIONAL_B_SPLINE_CURVE ( ( 0.9755282581475768211, 0.9755282581475771542, 1.000000000000000000, 0.9510565162951535312, 1.000000000000000000, 0.9510565162951535312, 1.000000000000000000, 0.9510565162951535312, 1.000000000000000000, 0.9510565162951535312, 1.000000000000000000, 0.9755282581475763770, 0.9755282581475768211 ) ) 
 REPRESENTATION_ITEM ( '' )  );
#15055=CARTESIAN_POINT ( 'NONE',  ( 30.81806926056964002, 42.55937500034139020, 42.41743335407647209 ) ) ;
#15058=ORIENTED_EDGE ( 'NONE', *, *, #13348, .T. ) ;
#15060=CARTESIAN_POINT ( 'NONE',  ( 40.34137639590981195, 37.05937500034139731, -29.30972558990011834 ) ) ;
#15063=CARTESIAN_POINT ( 'NONE',  ( 0.000000000000000000, 52.00000000000000711, 63.16733765196516970 ) ) ;
#15064=CARTESIAN_POINT ( 'NONE',  ( 46.85365039762147177, 25.00000000000000711, -17.06523097087115914 ) ) ;
#15070=CARTESIAN_POINT ( 'NONE',  ( -15.45084971874737256, 29.38125000068279746, -47.55282581475767500 ) ) ;
#15073=CARTESIAN_POINT ( 'NONE',  ( -15.40903463028481646, 33.52187500034140299, -47.42413220539093999 ) ) ;
#15075=EDGE_LOOP ( 'NONE', ( #9405, #7229, #15745, #7966 ) ) ;
#15076=CARTESIAN_POINT ( 'NONE',  ( 9.631387414534489405E-15, 38.35937500034139447, 52.43083105670540789 ) ) ;
#15080=CARTESIAN_POINT ( 'NONE',  ( 40.45084971874737789, 24.58125000068280031, 29.38926261462365375 ) ) ;
#15082=CARTESIAN_POINT ( 'NONE',  ( -40.34137639590981905, 23.72187500034139873, -29.30972558990011478 ) ) ;
#15084=CIRCLE ( 'NONE', #10324, 50.00000000000000000 ) ;
#15086=CARTESIAN_POINT ( 'NONE',  ( 8.446640517145639571E-15, 26.28125000068279959, 50.00000000000000000 ) ) ;
#15087=CARTESIAN_POINT ( 'NONE',  ( -40.45084971874737789, 49.80000000000000426, -29.38926261462365730 ) ) ;
#15090=LINE ( 'NONE', #3467, #1666 ) ;
#15091=CARTESIAN_POINT ( 'NONE',  ( -30.81806926056962226, 36.22187500034139873, 42.41743335407647919 ) ) ;
#15093=CARTESIAN_POINT ( 'NONE',  ( -49.99999999999999289, 31.68125000068279462, -16.24598481164531449 ) ) ;
#15096=ORIENTED_EDGE ( 'NONE', *, *, #7708, .T. ) ;
#15098=CARTESIAN_POINT ( 'NONE',  ( -3.111920190527341144E-15, 45.50000000000000000, -50.00000000000000000 ) ) ;
#15105=CARTESIAN_POINT ( 'NONE',  ( -3.111920190527341144E-15, 35.28125000068280315, -50.00000000000000000 ) ) ;
#15109=CARTESIAN_POINT ( 'NONE',  ( -49.86468353125000164, 23.85937500034139447, 0.000000000000000000 ) ) ;
#15111=CARTESIAN_POINT ( 'NONE',  ( -7.919222016226802552, 47.33250428222964956, -50.00000000000000000 ) ) ;
#15118=CARTESIAN_POINT ( 'NONE',  ( -40.45084971874737789, 37.79999999999999716, -29.38926261462365730 ) ) ;
#15121=CARTESIAN_POINT ( 'NONE',  ( 7.919222016226822092, 26.33250428222964246, 49.99999999999999289 ) ) ;
#15123=CARTESIAN_POINT ( 'NONE',  ( 0.000000000000000000, 51.99999999999999289, 0.000000000000000000 ) ) ;
#15130=CARTESIAN_POINT ( 'NONE',  ( 40.34137639590981905, 44.65937500034139163, 29.30972558990010768 ) ) ;
#15132=VERTEX_POINT ( 'NONE', #13154 ) ;
#15133=CARTESIAN_POINT ( 'NONE',  ( 0.000000000000000000, 272.0000000000000000, -42.00000000000000711 ) ) ;
#15134=CARTESIAN_POINT ( 'NONE',  ( 15.40903463028481113, 29.25937500034139660, -47.42413220539094709 ) ) ;
#15138=CARTESIAN_POINT ( 'NONE',  ( 45.18727525474233175, 25.00000000000000711, -21.08615623785931348 ) ) ;
#15139=CARTESIAN_POINT ( 'NONE',  ( 49.86468353125001585, 32.82187500034139305, 16.20201782572375038 ) ) ;
#15146=CARTESIAN_POINT ( 'NONE',  ( 7.919222016226693306, 32.55125428154685352, 50.00000000000003553 ) ) ;
#15150=CARTESIAN_POINT ( 'NONE',  ( 9.631387414534489405E-15, 28.42187500034139092, 52.43083105670540789 ) ) ;
#15154=CARTESIAN_POINT ( 'NONE',  ( 40.34137639590981905, 38.65937500034139873, 29.30972558990010768 ) ) ;
#15158=CARTESIAN_POINT ( 'NONE',  ( -30.81806926056962226, 46.15937500034139873, 42.41743335407647919 ) ) ;
#15160=CARTESIAN_POINT ( 'NONE',  ( -49.86468353124999453, 22.02187500034139589, 16.20201782572377525 ) ) ;
#15164=CARTESIAN_POINT ( 'NONE',  ( 40.45084971874737079, 47.20000000000000284, -29.38926261462366440 ) ) ;
#15166=CARTESIAN_POINT ( 'NONE',  ( -49.86468353124999453, 48.02187500034139589, 16.20201782572377525 ) ) ;
#15167=ADVANCED_FACE ( 'NONE', ( #15722 ), #1839, .T. ) ;
#15172=VERTEX_POINT ( 'NONE', #1999 ) ;
#15175=CARTESIAN_POINT ( 'NONE',  ( 50.00000000000000711, 44.90000000000000568, 16.24598481164530739 ) ) ;
#15178=SURFACE_STYLE_FILL_AREA ( #14016 ) ;
#15186=CARTESIAN_POINT ( 'NONE',  ( -49.86468353124999453, 27.95937500034139944, 16.20201782572377525 ) ) ;
#15203=CARTESIAN_POINT ( 'NONE',  ( 30.90169943749475578, 22.69999999999999929, 42.53254041760200010 ) ) ;
#15204=DIRECTION ( 'NONE',  ( -0.000000000000000000, -1.000000000000000000, -0.000000000000000000 ) ) ;
#15206=CARTESIAN_POINT ( 'NONE',  ( 40.34137639590981195, 41.05937500034139731, -29.30972558990011834 ) ) ;
#15212=CARTESIAN_POINT ( 'NONE',  ( 30.81806926056964002, 26.55937500034139376, 42.41743335407647209 ) ) ;
#15213=ORIENTED_EDGE ( 'NONE', *, *, #701, .F. ) ;
#15214=CARTESIAN_POINT ( 'NONE',  ( 15.45084971874736723, 27.40000000000000213, -47.55282581475768211 ) ) ;
#15216=CARTESIAN_POINT ( 'NONE',  ( 47.93512317712437465, 25.00000000000000000, -13.73719875613759989 ) ) ;
#15217=CARTESIAN_POINT ( 'NONE',  ( 40.34137639590981905, 34.72187500034139873, 29.30972558990010768 ) ) ;
#15218=CARTESIAN_POINT ( 'NONE',  ( 15.45084971874737789, 46.38125000068279746, 47.55282581475767500 ) ) ;
#15220=CARTESIAN_POINT ( 'NONE',  ( 0.000000000000000000, 193.4213562373095385, -50.00000000000000000 ) ) ;
#15225=CARTESIAN_POINT ( 'NONE',  ( -3.210462471511496205E-15, 29.42187500034139092, -52.43083105670540789 ) ) ;
#15232=CARTESIAN_POINT ( 'NONE',  ( -30.81806926056962226, 38.15937500034139163, 42.41743335407647209 ) ) ;
#15234=ORIENTED_EDGE ( 'NONE', *, *, #14086, .T. ) ;
#15237=CARTESIAN_POINT ( 'NONE',  ( -15.45084971874736368, 20.18125000068279817, 47.55282581475768211 ) ) ;
#15240=LINE ( 'NONE', #3865, #15770 ) ;
#15241=CARTESIAN_POINT ( 'NONE',  ( 30.81806926056962936, 23.22187500034139163, -42.41743335407647209 ) ) ;
#15243=ADVANCED_FACE ( 'NONE', ( #8567 ), #2124, .T. ) ;
#15246=CARTESIAN_POINT ( 'NONE',  ( 40.45084971874737079, 45.20000000000000284, -29.38926261462366440 ) ) ;
#15249=ADVANCED_FACE ( 'NONE', ( #4283, #10604 ), #15816, .F. ) ;
#15257=CARTESIAN_POINT ( 'NONE',  ( 0.000000000000000000, 53.82568851450475478, 0.000000000000000000 ) ) ;
#15262=CARTESIAN_POINT ( 'NONE',  ( -49.99999999999999289, 40.09999999999999432, 16.24598481164533226 ) ) ;
#15264=CARTESIAN_POINT ( 'NONE',  ( -30.90169943749473447, 36.08125000068279320, 42.53254041760200721 ) ) ;
#15266=ORIENTED_EDGE ( 'NONE', *, *, #13021, .F. ) ;
#15267=CARTESIAN_POINT ( 'NONE',  ( 40.34137639590981905, 48.72187500034139873, 29.30972558990010768 ) ) ;
#15271=ORIENTED_EDGE ( 'NONE', *, *, #8226, .F. ) ;
#15272=VERTEX_POINT ( 'NONE', #11179 ) ;
#15274=DIRECTION ( 'NONE',  ( 0.000000000000000000, 0.000000000000000000, -1.000000000000000000 ) ) ;
#15278=AXIS2_PLACEMENT_3D ( 'NONE', #10136, #3817, #5333 ) ;
#15288=DIRECTION ( 'NONE',  ( 0.000000000000000000, 0.000000000000000000, 1.000000000000000000 ) ) ;
#15295=CARTESIAN_POINT ( 'NONE',  ( 40.34137639590981195, 45.05937500034139731, -29.30972558990011834 ) ) ;
#15296=ORIENTED_EDGE ( 'NONE', *, *, #11096, .F. ) ;
#15302=CARTESIAN_POINT ( 'NONE',  ( -30.81806926056963292, 31.55937500034139731, -42.41743335407647209 ) ) ;
#15307=CARTESIAN_POINT ( 'NONE',  ( 30.81806926056964002, 34.62187500034139731, 42.41743335407646498 ) ) ;
#15312=CARTESIAN_POINT ( 'NONE',  ( 7.919222016226809657, 43.44874571845315359, -50.00000000000000000 ) ) ;
#15315=DIRECTION ( 'NONE',  ( 0.000000000000000000, 0.000000000000000000, -1.000000000000000000 ) ) ;
#15318=CARTESIAN_POINT ( 'NONE',  ( 15.40903463028481113, 33.32187500034139305, -47.42413220539094709 ) ) ;
#15321=CARTESIAN_POINT ( 'NONE',  ( 15.40903463028481113, 33.25937500034140015, -47.42413220539094709 ) ) ;
#15327=CARTESIAN_POINT ( 'NONE',  ( 40.34137639590981195, 49.05937500034139731, -29.30972558990011834 ) ) ;
#15328=DIRECTION ( 'NONE',  ( 0.000000000000000000, 0.000000000000000000, 1.000000000000000000 ) ) ;
#15329=CARTESIAN_POINT ( 'NONE',  ( 49.86468353125001585, 22.82187500034138949, 16.20201782572375038 ) ) ;
#15333=DIRECTION ( 'NONE',  ( 0.000000000000000000, 1.000000000000000000, 0.000000000000000000 ) ) ;
#15334=CARTESIAN_POINT ( 'NONE',  ( 30.90169943749475578, 46.69999999999999574, 42.53254041760200010 ) ) ;
#15342=CARTESIAN_POINT ( 'NONE',  ( 15.45084971874736723, 37.18125000068280173, -47.55282581475768211 ) ) ;
#15345=CARTESIAN_POINT ( 'NONE',  ( 30.90169943749473802, 45.29999999999999005, -42.53254041760200721 ) ) ;
#15346=EDGE_CURVE ( 'NONE', #14468, #11210, #3267, .T. ) ;
#15348=CARTESIAN_POINT ( 'NONE',  ( -30.81806926056963292, 49.62187500034139020, -42.41743335407646498 ) ) ;
#15355=DIRECTION ( 'NONE',  ( 0.000000000000000000, 1.000000000000000000, 0.000000000000000000 ) ) ;
#15356=CARTESIAN_POINT ( 'NONE',  ( 7.919222016226809657, 29.22999571913594963, -50.00000000000000000 ) ) ;
#15357=VERTEX_POINT ( 'NONE', #2257 ) ;
#15359=CARTESIAN_POINT ( 'NONE',  ( 49.86468353124999453, 47.02187500034139589, -16.20201782572376459 ) ) ;
#15369=CARTESIAN_POINT ( 'NONE',  ( 0.000000000000000000, 252.0000000000000000, 0.000000000000000000 ) ) ;
#15375=CARTESIAN_POINT ( 'NONE',  ( -50.00000000000000000, 22.00000000000000355, 0.000000000000000000 ) ) ;
#15379=EDGE_CURVE ( 'NONE', #3842, #1639, #9762, .T. ) ;
#15380=CARTESIAN_POINT ( 'NONE',  ( -30.81806926056963292, 35.55937500034139020, -42.41743335407647209 ) ) ;
#15382=ORIENTED_EDGE ( 'NONE', *, *, #5722, .F. ) ;
#15385=CARTESIAN_POINT ( 'NONE',  ( 15.40903463028482356, 30.45937500034139589, 47.42413220539093999 ) ) ;
#15389=CARTESIAN_POINT ( 'NONE',  ( 47.69912754770714258, 25.00000000000000711, -14.53642574140263299 ) ) ;
#15390=CARTESIAN_POINT ( 'NONE',  ( 30.81806926056962936, 31.22187500034139518, -42.41743335407646498 ) ) ;
#15402=CARTESIAN_POINT ( 'NONE',  ( -30.81806926056963292, 31.62187500034139731, -42.41743335407647209 ) ) ;
#15404=EDGE_CURVE ( 'NONE', #15953, #1138, #266, .T. ) ;
#15406=CARTESIAN_POINT ( 'NONE',  ( -49.86468353124999453, 35.95937500034139589, 16.20201782572377169 ) ) ;
#15407=ORIENTED_EDGE ( 'NONE', *, *, #2445, .F. ) ;
#15410=CARTESIAN_POINT ( 'NONE',  ( 30.81806926056962936, 47.15937500034138452, -42.41743335407647209 ) ) ;
#15412=CARTESIAN_POINT ( 'NONE',  ( -30.81806926056963292, 25.62187500034139731, -42.41743335407647209 ) ) ;
#15416=CARTESIAN_POINT ( 'NONE',  ( -49.99999999999999289, 45.89999999999999858, -16.24598481164531449 ) ) ;
#15422=CARTESIAN_POINT ( 'NONE',  ( -40.45084971874737789, 37.58125000068280031, -29.38926261462365730 ) ) ;
#15427=CARTESIAN_POINT ( 'NONE',  ( 49.86468353125001585, 48.82187500034139305, 16.20201782572375038 ) ) ;
#15438=CARTESIAN_POINT ( 'NONE',  ( 49.86468353125000164, 48.92187500034139447, -6.106662507704105588E-15 ) ) ;
#15445=EDGE_CURVE ( 'NONE', #5291, #495, #4614, .T. ) ;
#15446=EDGE_CURVE ( 'NONE', #5162, #6674, #14137, .T. ) ;
#15455=CARTESIAN_POINT ( 'NONE',  ( -15.45084971874737256, 37.38125000068279746, -47.55282581475767500 ) ) ;
#15456=( BOUNDED_CURVE ( )  B_SPLINE_CURVE ( 2, ( #765, #13400, #5856, #12421, #1012, #2095, #12073, #2258, #6109, #16234, #4868, #3186, #13324 ),
 .UNSPECIFIED., .F., .F. ) 
 B_SPLINE_CURVE_WITH_KNOTS ( ( 3, 2, 2, 2, 2, 2, 3 ),
 ( 0.1499999999999999944, 0.1533333333333333215, 0.1600000000000000033, 0.1666666666666666574, 0.1733333333333333393, 0.1799999999999999933, 0.1833333333333333481 ),
 .UNSPECIFIED. ) 
 CURVE ( )  GEOMETRIC_REPRESENTATION_ITEM ( )  RATIONAL_B_SPLINE_CURVE ( ( 0.9755282581475768211, 0.9755282581475768211, 1.000000000000000000, 0.9510565162951535312, 1.000000000000000000, 0.9510565162951535312, 1.000000000000000000, 0.9510565162951535312, 1.000000000000000000, 0.9510565162951535312, 1.000000000000000000, 0.9755282581475765991, 0.9755282581475767101 ) ) 
 REPRESENTATION_ITEM ( '' )  );
#15457=CARTESIAN_POINT ( 'NONE',  ( -3.219174618344376363E-15, 23.50000000000000000, -52.57311121191334990 ) ) ;
#15460=CARTESIAN_POINT ( 'NONE',  ( -40.34137639590981195, 38.05937500034139731, 29.30972558990012189 ) ) ;
#15462=CARTESIAN_POINT ( 'NONE',  ( 0.000000000000000000, 52.00000000000000711, 0.000000000000000000 ) ) ;
#15463=CARTESIAN_POINT ( 'NONE',  ( 9.735664389687646693E-15, 272.0000000000000000, 79.49773270518484480 ) ) ;
#15464=CARTESIAN_POINT ( 'NONE',  ( -30.81806926056962226, 28.15937500034139518, 42.41743335407647919 ) ) ;
#15470=CARTESIAN_POINT ( 'NONE',  ( 30.81806926056962936, 33.22187500034139163, -42.41743335407646498 ) ) ;
#15478=CARTESIAN_POINT ( 'NONE',  ( -40.34137639590981195, 28.12187500034139731, 29.30972558990012189 ) ) ;
#15481=VERTEX_POINT ( 'NONE', #14381 ) ;
#15482=CARTESIAN_POINT ( 'NONE',  ( -30.81806926056963292, 27.55937500034139376, -42.41743335407646498 ) ) ;
#15485=CARTESIAN_POINT ( 'NONE',  ( 15.45084971874736723, 21.18125000068279817, -47.55282581475768211 ) ) ;
#15493=CARTESIAN_POINT ( 'NONE',  ( -15.45084971874737256, 41.60000000000000142, -47.55282581475767500 ) ) ;
#15496=CARTESIAN_POINT ( 'NONE',  ( -30.81806926056962226, 48.22187500034139163, 42.41743335407647919 ) ) ;
#15501=CARTESIAN_POINT ( 'NONE',  ( 15.45084971874737789, 40.38125000068280457, 47.55282581475767500 ) ) ;
#15506=CARTESIAN_POINT ( 'NONE',  ( -40.34137639590981905, 45.72187500034139873, -29.30972558990011478 ) ) ;
#15509=AXIS2_PLACEMENT_3D ( 'NONE', #16040, #2151, #4925 ) ;
#15512=CARTESIAN_POINT ( 'NONE',  ( 48.35726954556789536, 24.99999999999999645, -12.16803787670825265 ) ) ;
#15516=CARTESIAN_POINT ( 'NONE',  ( 49.86468353125001585, 48.82187500034139305, 16.20201782572375038 ) ) ;
#15521=CONICAL_SURFACE ( 'NONE', #14445, 62.01141590572476758, 0.08726646259971666819 ) ;
#15526=CARTESIAN_POINT ( 'NONE',  ( 49.99999999999999289, 29.10000000000000142, -16.24598481164532160 ) ) ;
#15531=CARTESIAN_POINT ( 'NONE',  ( -50.00000000000000000, 46.00000000000000000, 0.000000000000000000 ) ) ;
#15533=DIRECTION ( 'NONE',  ( 0.000000000000000000, -0.000000000000000000, 1.000000000000000000 ) ) ;
#15536=CARTESIAN_POINT ( 'NONE',  ( -15.45084971874736368, 38.18125000068280173, 47.55282581475768211 ) ) ;
#15538=DIRECTION ( 'NONE',  ( -0.000000000000000000, -1.000000000000000000, -0.000000000000000000 ) ) ;
#15541=ORIENTED_EDGE ( 'NONE', *, *, #13125, .F. ) ;
#15542=CARTESIAN_POINT ( 'NONE',  ( -3.210462471511496205E-15, 35.35937500034140157, -52.43083105670540789 ) ) ;
#15545=CARTESIAN_POINT ( 'NONE',  ( -3.219174618344376363E-15, 47.28125000068278894, -52.57311121191334990 ) ) ;
#15546=AXIS2_PLACEMENT_3D ( 'NONE', #10221, #6576, #15274 ) ;
#15548=CARTESIAN_POINT ( 'NONE',  ( -40.34137639590981195, 20.05937500034139731, 29.30972558990012189 ) ) ;
#15553=CARTESIAN_POINT ( 'NONE',  ( 50.00000000000000000, 35.00000000000000000, -6.123233995736766085E-15 ) ) ;
#15555=CARTESIAN_POINT ( 'NONE',  ( -49.86468353124999453, 26.02187500034139589, 16.20201782572377169 ) ) ;
#15564=CARTESIAN_POINT ( 'NONE',  ( 50.00000000000000000, 35.00000000000000000, -6.123233995736766085E-15 ) ) ;
#15568=AXIS2_PLACEMENT_3D ( 'NONE', #12551, #2405, #7651 ) ;
#15573=CARTESIAN_POINT ( 'NONE',  ( 49.86468353125001585, 26.75937500034139660, 16.20201782572375038 ) ) ;
#15576=CARTESIAN_POINT ( 'NONE',  ( 49.86468353125001585, 42.75937500034138594, 16.20201782572375038 ) ) ;
#15580=VECTOR ( 'NONE', #79, 1000.000000000000000 ) ;
#15585=CARTESIAN_POINT ( 'NONE',  ( 50.00000000000000000, 39.00000000000000000, -6.123233995736766085E-15 ) ) ;
#15587=CARTESIAN_POINT ( 'NONE',  ( -15.40903463028481646, 43.52187500034139589, -47.42413220539093999 ) ) ;
#15592=( BOUNDED_CURVE ( )  B_SPLINE_CURVE ( 2, ( #13813, #3848, #7586, #3931, #6431, #2425, #14060, #6266, #8913, #12664, #2676, #11337, #16404 ),
 .UNSPECIFIED., .F., .F. ) 
 B_SPLINE_CURVE_WITH_KNOTS ( ( 3, 2, 2, 2, 2, 2, 3 ),
 ( 0.6166666666666666963, 0.6199999999999999956, 0.6266666666666667052, 0.6333333333333333037, 0.6400000000000000133, 0.6466666666666666119, 0.6500000000000000222 ),
 .UNSPECIFIED. ) 
 CURVE ( )  GEOMETRIC_REPRESENTATION_ITEM ( )  RATIONAL_B_SPLINE_CURVE ( ( 0.9755282581475768211, 0.9755282581475771542, 1.000000000000000000, 0.9510565162951535312, 1.000000000000000000, 0.9510565162951535312, 1.000000000000000000, 0.9510565162951535312, 1.000000000000000000, 0.9510565162951535312, 1.000000000000000000, 0.9755282581475763770, 0.9755282581475768211 ) ) 
 REPRESENTATION_ITEM ( '' )  );
#15595=CARTESIAN_POINT ( 'NONE',  ( 40.45084971874737079, 30.98125000068279888, -29.38926261462366440 ) ) ;
#15596=AXIS2_PLACEMENT_3D ( 'NONE', #16068, #7359, #15985 ) ;
#15601=CARTESIAN_POINT ( 'NONE',  ( -49.86468353124999453, 44.02187500034139589, 16.20201782572377169 ) ) ;
#15605=PRODUCT_CONTEXT ( 'NONE', #13844, 'mechanical' ) ;
#15610=CARTESIAN_POINT ( 'NONE',  ( 40.34137639590981195, 21.05937500034139376, -29.30972558990011834 ) ) ;
#15615=LINE ( 'NONE', #6742, #2106 ) ;
#15629=CARTESIAN_POINT ( 'NONE',  ( 40.34137639590981905, 36.65937500034139873, 29.30972558990010768 ) ) ;
#15636=CARTESIAN_POINT ( 'NONE',  ( -30.81806926056963292, 21.55937500034140086, -42.41743335407647209 ) ) ;
#15639=CARTESIAN_POINT ( 'NONE',  ( 7.919222016226809657, 35.44874571845314648, -50.00000000000000000 ) ) ;
#15641=CARTESIAN_POINT ( 'NONE',  ( 40.34137639590981905, 30.72187500034139518, 29.30972558990010768 ) ) ;
#15647=MECHANICAL_DESIGN_GEOMETRIC_PRESENTATION_REPRESENTATION('',(#5827),#14049);
#15648=CARTESIAN_POINT ( 'NONE',  ( -15.45084971874736368, 34.39999999999999858, 47.55282581475768211 ) ) ;
#15653=CARTESIAN_POINT ( 'NONE',  ( -3.210462471511496205E-15, 29.35937500034139802, -52.43083105670540789 ) ) ;
#15656=CARTESIAN_POINT ( 'NONE',  ( 49.86468353125001585, 44.75937500034138594, 16.20201782572375038 ) ) ;
#15666=CARTESIAN_POINT ( 'NONE',  ( -15.45084971874737256, 43.60000000000000142, -47.55282581475767500 ) ) ;
#15669=CARTESIAN_POINT ( 'NONE',  ( -30.81806926056963292, 43.62187500034139020, -42.41743335407647209 ) ) ;
#15673=CARTESIAN_POINT ( 'NONE',  ( -30.90169943749474868, 31.48125000068279533, -42.53254041760200721 ) ) ;
#15674=VERTEX_POINT ( 'NONE', #10824 ) ;
#15676=DIRECTION ( 'NONE',  ( 0.8660254037844513642, 0.4999999999999780731, 0.000000000000000000 ) ) ;
#15677=CARTESIAN_POINT ( 'NONE',  ( 49.86468353124999453, 49.02187500034140299, -16.20201782572376104 ) ) ;
#15683=ORIENTED_EDGE ( 'NONE', *, *, #16062, .F. ) ;
#15684=CARTESIAN_POINT ( 'NONE',  ( 15.40903463028481113, 41.32187500034140015, -47.42413220539094709 ) ) ;
#15687=ORIENTED_EDGE ( 'NONE', *, *, #4003, .F. ) ;
#15693=CARTESIAN_POINT ( 'NONE',  ( 7.919222016226822092, 48.33250428222964246, 49.99999999999999289 ) ) ;
#15695=CARTESIAN_POINT ( 'NONE',  ( -49.99999999999999289, 46.09999999999999432, 16.24598481164533226 ) ) ;
#15704=CARTESIAN_POINT ( 'NONE',  ( -30.81806926056962226, 36.15937500034139163, 42.41743335407647919 ) ) ;
#15709=CARTESIAN_POINT ( 'NONE',  ( 30.81806926056964002, 22.55937500034139020, 42.41743335407647209 ) ) ;
#15714=CARTESIAN_POINT ( 'NONE',  ( 40.34137639590981195, 25.12187500034139376, -29.30972558990011834 ) ) ;
#15719=CARTESIAN_POINT ( 'NONE',  ( 0.000000000000000000, 193.4213562373095385, 0.000000000000000000 ) ) ;
#15720=CARTESIAN_POINT ( 'NONE',  ( 50.00000000000000711, 34.89999999999998437, 16.24598481164530739 ) ) ;
#15722=FACE_OUTER_BOUND ( 'NONE', #8866, .T. ) ;
#15726=CARTESIAN_POINT ( 'NONE',  ( 49.86468353124999453, 28.95937500034139589, -16.20201782572376104 ) ) ;
#15728=CARTESIAN_POINT ( 'NONE',  ( -3.111920190527341144E-15, 35.50000000000000000, -50.00000000000000000 ) ) ;
#15729=CARTESIAN_POINT ( 'NONE',  ( 49.86468353125000164, 42.85937500034140157, -6.106662507704105588E-15 ) ) ;
#15735=CARTESIAN_POINT ( 'NONE',  ( -30.81806926056962226, 30.22187500034139518, 42.41743335407647919 ) ) ;
#15736=CARTESIAN_POINT ( 'NONE',  ( 15.45084971874737789, 40.60000000000000142, 47.55282581475767500 ) ) ;
#15740=CARTESIAN_POINT ( 'NONE',  ( -3.210462471511496205E-15, 41.42187500034140157, -52.43083105670540789 ) ) ;
#15744=CARTESIAN_POINT ( 'NONE',  ( 9.631387414534489405E-15, 46.35937500034139447, 52.43083105670540789 ) ) ;
#15745=ORIENTED_EDGE ( 'NONE', *, *, #11930, .F. ) ;
#15746=CARTESIAN_POINT ( 'NONE',  ( 30.90169943749475578, 30.48125000068279533, 42.53254041760200010 ) ) ;
#15750=CARTESIAN_POINT ( 'NONE',  ( 0.000000000000000000, 193.4213562373095385, 0.000000000000000000 ) ) ;
#15751=CARTESIAN_POINT ( 'NONE',  ( 40.45084971874737789, 32.58125000068280031, 29.38926261462365375 ) ) ;
#15752=CARTESIAN_POINT ( 'NONE',  ( 40.34137639590981905, 40.72187500034139873, 29.30972558990010768 ) ) ;
#15763=CARTESIAN_POINT ( 'NONE',  ( -3.210462471511496205E-15, 41.42187500034140157, -52.43083105670540789 ) ) ;
#15769=DIRECTION ( 'NONE',  ( 0.000000000000000000, 1.000000000000000000, 0.000000000000000000 ) ) ;
#15770=VECTOR ( 'NONE', #5377, 1000.000000000000227 ) ;
#15777=CARTESIAN_POINT ( 'NONE',  ( -30.90169943749474513, 33.48125000068279888, -42.53254041760200721 ) ) ;
#15779=CARTESIAN_POINT ( 'NONE',  ( -49.93234176562499727, 49.96093750017070079, 0.000000000000000000 ) ) ;
#15782=VECTOR ( 'NONE', #10625, 1000.000000000000000 ) ;
#15785=CARTESIAN_POINT ( 'NONE',  ( -3.210462471511496205E-15, 29.35937500034139802, -52.43083105670540789 ) ) ;
#15789=ADVANCED_FACE ( 'NONE', ( #3421 ), #9649, .F. ) ;
#15790=CARTESIAN_POINT ( 'NONE',  ( 15.45084971874737789, 48.38125000068280457, 47.55282581475767500 ) ) ;
#15792=CARTESIAN_POINT ( 'NONE',  ( -3.210462471511496205E-15, 21.35937500034139092, -52.43083105670540789 ) ) ;
#15793=VERTEX_POINT ( 'NONE', #2078 ) ;
#15797=CARTESIAN_POINT ( 'NONE',  ( -15.40903463028480580, 28.32187500034139660, 47.42413220539094709 ) ) ;
#15799=CARTESIAN_POINT ( 'NONE',  ( 7.919222016226758143, 38.55125428154684641, 50.00000000000000711 ) ) ;
#15804=CARTESIAN_POINT ( 'NONE',  ( -49.99999999999999289, 33.90000000000000568, -16.24598481164531449 ) ) ;
#15806=CARTESIAN_POINT ( 'NONE',  ( -30.81806926056963292, 47.55937500034139731, -42.41743335407647209 ) ) ;
#15810=CARTESIAN_POINT ( 'NONE',  ( -40.34137639590981905, 31.65937500034139873, -29.30972558990011478 ) ) ;
#15812=AXIS2_PLACEMENT_3D ( 'NONE', #2158, #11073, #8560 ) ;
#15814=CARTESIAN_POINT ( 'NONE',  ( -3.210462471511496205E-15, 39.35937500034138736, -52.43083105670540789 ) ) ;
#15815=ADVANCED_FACE ( 'NONE', ( #10979 ), #16043, .F. ) ;
#15816=PLANE ( 'NONE',  #13090 ) ;
#15821=AXIS2_PLACEMENT_3D ( 'NONE', #2421, #9841, #16063 ) ;
#15823=CARTESIAN_POINT ( 'NONE',  ( 40.34137639590981195, 29.12187500034139376, -29.30972558990011834 ) ) ;
#15825=CARTESIAN_POINT ( 'NONE',  ( 30.90169943749474157, 43.30000000000000426, -42.53254041760200721 ) ) ;
#15827=CARTESIAN_POINT ( 'NONE',  ( -15.40903463028480580, 46.32187500034140015, 47.42413220539094709 ) ) ;
#15833=CARTESIAN_POINT ( 'NONE',  ( -49.86468353125000164, 49.85937500034139447, 0.000000000000000000 ) ) ;
#15839=CARTESIAN_POINT ( 'NONE',  ( -40.45084971874737079, 31.98125000068280244, 29.38926261462367151 ) ) ;
#15844=CARTESIAN_POINT ( 'NONE',  ( -49.86468353124999453, 40.02187500034139589, 16.20201782572377169 ) ) ;
#15853=CARTESIAN_POINT ( 'NONE',  ( -15.45084971874737256, 45.38125000068279746, -47.55282581475767500 ) ) ;
#15855=CARTESIAN_POINT ( 'NONE',  ( 40.34137639590981195, 41.12187500034139731, -29.30972558990011834 ) ) ;
#15856=ORIENTED_EDGE ( 'NONE', *, *, #8445, .F. ) ;
#15859=ORIENTED_EDGE ( 'NONE', *, *, #3634, .F. ) ;
#15862=CARTESIAN_POINT ( 'NONE',  ( 0.000000000000000000, 252.0000000000000000, 0.000000000000000000 ) ) ;
#15870=DIRECTION ( 'NONE',  ( -0.000000000000000000, -1.000000000000000000, -0.000000000000000000 ) ) ;
#15872=CIRCLE ( 'NONE', #208, 47.00000000000000000 ) ;
#15873=CARTESIAN_POINT ( 'NONE',  ( 7.513064459987437071E-14, 42.28125000068280315, 50.00000000000000000 ) ) ;
#15876=CARTESIAN_POINT ( 'NONE',  ( -40.34137639590981195, 34.05937500034139731, 29.30972558990012189 ) ) ;
#15877=ORIENTED_EDGE ( 'NONE', *, *, #9667, .T. ) ;
#15879=ORIENTED_EDGE ( 'NONE', *, *, #4962, .T. ) ;
#15880=CARTESIAN_POINT ( 'NONE',  ( -30.90169943749473802, 46.08125000068278609, 42.53254041760200721 ) ) ;
#15882=DIRECTION ( 'NONE',  ( 0.000000000000000000, 1.000000000000000000, 0.000000000000000000 ) ) ;
#15883=EDGE_LOOP ( 'NONE', ( #9285, #7622 ) ) ;
#15885=CARTESIAN_POINT ( 'NONE',  ( -50.00000000000000000, 48.00000000000000000, 0.000000000000000000 ) ) ;
#15888=CARTESIAN_POINT ( 'NONE',  ( 9.631387414534489405E-15, 26.42187500034139447, 52.43083105670540789 ) ) ;
#15892=ADVANCED_FACE ( 'NONE', ( #3670 ), #15042, .T. ) ;
#15895=CARTESIAN_POINT ( 'NONE',  ( 9.657523855033129090E-15, 36.50000000000000711, 52.57311121191334990 ) ) ;
#15897=CARTESIAN_POINT ( 'NONE',  ( -15.40903463028481646, 49.45937500034140299, -47.42413220539093999 ) ) ;
#15901=CARTESIAN_POINT ( 'NONE',  ( 6.123233995736766085E-15, 193.4213562373095385, 50.00000000000000000 ) ) ;
#15904=CARTESIAN_POINT ( 'NONE',  ( 49.86468353125001585, 38.75937500034139305, 16.20201782572375038 ) ) ;
#15910=CARTESIAN_POINT ( 'NONE',  ( 40.34137639590981905, 32.72187500034139873, 29.30972558990010768 ) ) ;
#15913=CARTESIAN_POINT ( 'NONE',  ( 30.81806926056962936, 47.22187500034139873, -42.41743335407647209 ) ) ;
#15918=CARTESIAN_POINT ( 'NONE',  ( -49.86468353124999453, 49.75937500034137884, -16.20201782572375393 ) ) ;
#15921=CARTESIAN_POINT ( 'NONE',  ( -40.45084971874737789, 33.58125000068280031, -29.38926261462365730 ) ) ;
#15924=CARTESIAN_POINT ( 'NONE',  ( 49.86468353125000164, 40.92187500034139447, -6.106662507704105588E-15 ) ) ;
#15927=( BOUNDED_CURVE ( )  B_SPLINE_CURVE ( 2, ( #15086, #3790, #7613, #11360, #12687, #8855, #1284, #12932, #7853, #2620, #7524, #4033, #6626 ),
 .UNSPECIFIED., .F., .F. ) 
 B_SPLINE_CURVE_WITH_KNOTS ( ( 3, 2, 2, 2, 2, 2, 3 ),
 ( 0.7833333333333333259, 0.7866666666666666252, 0.7933333333333333348, 0.8000000000000000444, 0.8066666666666666430, 0.8133333333333333526, 0.8166666666666666519 ),
 .UNSPECIFIED. ) 
 CURVE ( )  GEOMETRIC_REPRESENTATION_ITEM ( )  RATIONAL_B_SPLINE_CURVE ( ( 0.9755282581475768211, 0.9755282581475768211, 1.000000000000000000, 0.9510565162951535312, 1.000000000000000000, 0.9510565162951535312, 1.000000000000000000, 0.9510565162951535312, 1.000000000000000000, 0.9510565162951535312, 1.000000000000000000, 0.9755282581475768211, 0.9755282581475768211 ) ) 
 REPRESENTATION_ITEM ( '' )  );
#15928=CARTESIAN_POINT ( 'NONE',  ( 9.631387414534489405E-15, 24.42187500034139447, 52.43083105670540789 ) ) ;
#15933=CARTESIAN_POINT ( 'NONE',  ( -3.210462471511496205E-15, 39.42187500034140157, -52.43083105670540789 ) ) ;
#15944=DIRECTION ( 'NONE',  ( -0.000000000000000000, -1.000000000000000000, -0.000000000000000000 ) ) ;
#15945=( NAMED_UNIT ( * ) SI_UNIT ( $, .STERADIAN. ) SOLID_ANGLE_UNIT ( ) );
#15950=ORIENTED_EDGE ( 'NONE', *, *, #15379, .T. ) ;
#15951=CARTESIAN_POINT ( 'NONE',  ( 49.86468353125000164, 30.85937500034139802, -6.106662507704105588E-15 ) ) ;
#15953=VERTEX_POINT ( 'NONE', #9902 ) ;
#15956=CARTESIAN_POINT ( 'NONE',  ( -15.45084971874737256, 45.38125000068279746, -47.55282581475767500 ) ) ;
#15960=CARTESIAN_POINT ( 'NONE',  ( -49.99999999999999289, 27.88125000068280102, 16.24598481164533226 ) ) ;
#15968=LINE ( 'NONE', #8321, #11709 ) ;
#15972=CARTESIAN_POINT ( 'NONE',  ( -15.45084971874737256, 27.60000000000000142, -47.55282581475767500 ) ) ;
#15974=CARTESIAN_POINT ( 'NONE',  ( 49.86468353125000164, 48.85937500034139447, -6.106662507704105588E-15 ) ) ;
#15976=CARTESIAN_POINT ( 'NONE',  ( 43.10890719796073256, 25.03031439394993640, -25.50054622961014061 ) ) ;
#15979=CARTESIAN_POINT ( 'NONE',  ( -30.81806926056963292, 33.55937500034138310, -42.41743335407647209 ) ) ;
#15985=DIRECTION ( 'NONE',  ( 0.000000000000000000, 0.000000000000000000, 1.000000000000000000 ) ) ;
#15986=CARTESIAN_POINT ( 'NONE',  ( -40.34137639590981195, 30.12187500034139731, 29.30972558990012189 ) ) ;
#15990=CARTESIAN_POINT ( 'NONE',  ( 40.34137639590981195, 35.12187500034139731, -29.30972558990011834 ) ) ;
#15993=VERTEX_POINT ( 'NONE', #3912 ) ;
#15994=CARTESIAN_POINT ( 'NONE',  ( -49.86468353124999453, 39.75937500034139305, -16.20201782572375393 ) ) ;
#15996=CARTESIAN_POINT ( 'NONE',  ( 50.00000000000000711, 22.68125000068279462, 16.24598481164530739 ) ) ;
#16000=CARTESIAN_POINT ( 'NONE',  ( 15.40903463028481113, 41.32187500034140015, -47.42413220539094709 ) ) ;
#16001=EDGE_CURVE ( 'NONE', #7138, #14296, #3299, .T. ) ;
#16004=CARTESIAN_POINT ( 'NONE',  ( 15.40903463028482356, 26.52187500034139589, 47.42413220539093999 ) ) ;
#16011=CARTESIAN_POINT ( 'NONE',  ( 49.86468353125001585, 42.82187500034139305, 16.20201782572375038 ) ) ;
#16012=CARTESIAN_POINT ( 'NONE',  ( -7.919222016226688865, 31.33250428222963890, -50.00000000000003553 ) ) ;
#16018=( BOUNDED_CURVE ( )  B_SPLINE_CURVE ( 2, ( #15098, #10292, #5235, #15345, #11371, #11212, #16437, #15175, #5071, #8702, #10124, #3803, #8867 ),
 .UNSPECIFIED., .F., .F. ) 
 B_SPLINE_CURVE_WITH_KNOTS ( ( 3, 2, 2, 2, 2, 2, 3 ),
 ( 0.1499999999999999944, 0.1533333333333333215, 0.1600000000000000033, 0.1666666666666666574, 0.1733333333333333393, 0.1799999999999999933, 0.1833333333333333481 ),
 .UNSPECIFIED. ) 
 CURVE ( )  GEOMETRIC_REPRESENTATION_ITEM ( )  RATIONAL_B_SPLINE_CURVE ( ( 0.9755282581475768211, 0.9755282581475768211, 1.000000000000000000, 0.9510565162951535312, 1.000000000000000000, 0.9510565162951535312, 1.000000000000000000, 0.9510565162951535312, 1.000000000000000000, 0.9510565162951535312, 1.000000000000000000, 0.9755282581475765991, 0.9755282581475767101 ) ) 
 REPRESENTATION_ITEM ( '' )  );
#16031=CARTESIAN_POINT ( 'NONE',  ( -30.81806926056962226, 32.15937500034139873, 42.41743335407647919 ) ) ;
#16035=ORIENTED_EDGE ( 'NONE', *, *, #14923, .T. ) ;
#16036=CARTESIAN_POINT ( 'NONE',  ( -49.99999999999999289, 41.68125000068280173, -16.24598481164531449 ) ) ;
#16040=CARTESIAN_POINT ( 'NONE',  ( 0.000000000000000000, 272.0000000000000000, 0.000000000000000000 ) ) ;
#16043=CYLINDRICAL_SURFACE ( 'NONE', #12840, 47.00000000000000000 ) ;
#16052=CARTESIAN_POINT ( 'NONE',  ( -50.00000000000000000, 26.00000000000000355, 0.000000000000000000 ) ) ;
#16057=CARTESIAN_POINT ( 'NONE',  ( -49.86468353125000164, 25.85937500034139802, 0.000000000000000000 ) ) ;
#16058=VERTEX_POINT ( 'NONE', #13208 ) ;
#16060=CARTESIAN_POINT ( 'NONE',  ( -3.210462471511496205E-15, 35.35937500034140157, -52.43083105670540789 ) ) ;
#16062=EDGE_CURVE ( 'NONE', #15993, #4476, #8836, .T. ) ;
#16063=DIRECTION ( 'NONE',  ( 0.000000000000000000, 0.000000000000000000, 1.000000000000000000 ) ) ;
#16068=CARTESIAN_POINT ( 'NONE',  ( 0.000000000000000000, 52.26146722824297797, 0.000000000000000000 ) ) ;
#16069=CARTESIAN_POINT ( 'NONE',  ( 30.81806926056964002, 30.62187500034139020, 42.41743335407647209 ) ) ;
#16073=CARTESIAN_POINT ( 'NONE',  ( -40.34137639590981905, 37.72187500034139873, -29.30972558990011478 ) ) ;
#16079=CARTESIAN_POINT ( 'NONE',  ( -30.81806926056962226, 44.15937500034139163, 42.41743335407647209 ) ) ;
#16080=ORIENTED_EDGE ( 'NONE', *, *, #6710, .T. ) ;
#16081=CARTESIAN_POINT ( 'NONE',  ( -50.00000000000000000, 25.78125000068279959, 0.000000000000000000 ) ) ;
#16084=AXIS2_PLACEMENT_3D ( 'NONE', #10004, #3438, #3349 ) ;
#16087=CARTESIAN_POINT ( 'NONE',  ( -49.99999999999999289, 35.89999999999999858, -16.24598481164531449 ) ) ;
#16088=CARTESIAN_POINT ( 'NONE',  ( 40.34137639590981195, 39.12187500034139731, -29.30972558990011834 ) ) ;
#16090=APPLICATION_CONTEXT ( 'automotive_design' ) ;
#16092=CARTESIAN_POINT ( 'NONE',  ( 40.45084971874737079, 41.20000000000000284, -29.38926261462366440 ) ) ;
#16093=CARTESIAN_POINT ( 'NONE',  ( 49.86468353125000164, 26.92187500034139802, -6.106662507704105588E-15 ) ) ;
#16101=ORIENTED_EDGE ( 'NONE', *, *, #4203, .F. ) ;
#16102=CARTESIAN_POINT ( 'NONE',  ( 30.81806926056964002, 36.62187500034139731, 42.41743335407647209 ) ) ;
#16103=CARTESIAN_POINT ( 'NONE',  ( -15.45084971874736368, 44.18125000068280173, 47.55282581475768211 ) ) ;
#16108=CARTESIAN_POINT ( 'NONE',  ( -50.00000000000000000, 50.00000000000000000, 0.000000000000000000 ) ) ;
#16118=SURFACE_STYLE_FILL_AREA ( #7311 ) ;
#16119=CYLINDRICAL_SURFACE ( 'NONE', #1950, 42.00000000000000711 ) ;
#16124=CARTESIAN_POINT ( 'NONE',  ( 30.81806926056964002, 30.55937500034139731, 42.41743335407647209 ) ) ;
#16129=AXIS2_PLACEMENT_3D ( 'NONE', #13682, #10952, #4483 ) ;
#16131=CARTESIAN_POINT ( 'NONE',  ( -15.45084971874737256, 43.38125000068279746, -47.55282581475767500 ) ) ;
#16140=CARTESIAN_POINT ( 'NONE',  ( 30.90169943749475223, 38.69999999999999574, 42.53254041760199300 ) ) ;
#16145=CARTESIAN_POINT ( 'NONE',  ( 50.00000000000000000, 31.00000000000000355, -6.123233995736766085E-15 ) ) ;
#16153=CARTESIAN_POINT ( 'NONE',  ( 49.86468353125001585, 32.75937500034140015, 16.20201782572375038 ) ) ;
#16154=CARTESIAN_POINT ( 'NONE',  ( 7.919222016226758143, 40.33250428222964246, 50.00000000000000711 ) ) ;
#16165=CARTESIAN_POINT ( 'NONE',  ( -49.86468353124999453, 38.02187500034140299, 16.20201782572377525 ) ) ;
#16169=CARTESIAN_POINT ( 'NONE',  ( 15.40903463028481113, 45.25937500034140015, -47.42413220539094709 ) ) ;
#16171=CARTESIAN_POINT ( 'NONE',  ( 15.45084971874737789, 26.38125000068280102, 47.55282581475767500 ) ) ;
#16176=CARTESIAN_POINT ( 'NONE',  ( -40.34137639590981905, 33.72187500034139873, -29.30972558990011478 ) ) ;
#16179=CARTESIAN_POINT ( 'NONE',  ( 7.919222016226940219, 31.44874571845315714, -49.99999999999996447 ) ) ;
#16180=CARTESIAN_POINT ( 'NONE',  ( -15.40903463028481646, 25.52187500034139589, -47.42413220539093999 ) ) ;
#16186=CARTESIAN_POINT ( 'NONE',  ( -3.210462471511496205E-15, 37.42187500034140157, -52.43083105670540789 ) ) ;
#16191=LINE ( 'NONE', #801, #5775 ) ;
#16195=AXIS2_PLACEMENT_3D ( 'NONE', #8214, #5493, #11876 ) ;
#16199=CARTESIAN_POINT ( 'NONE',  ( -30.90169943749473447, 40.30000000000000426, 42.53254041760200721 ) ) ;
#16203=CARTESIAN_POINT ( 'NONE',  ( -3.210462471511496205E-15, 25.35937500034139802, -52.43083105670540789 ) ) ;
#16206=ORIENTED_EDGE ( 'NONE', *, *, #1806, .F. ) ;
#16207=CARTESIAN_POINT ( 'NONE',  ( 50.00000000000000000, 46.78125000068279604, -6.123233995736766085E-15 ) ) ;
#16209=DIRECTION ( 'NONE',  ( 0.000000000000000000, 0.000000000000000000, 1.000000000000000000 ) ) ;
#16211=CARTESIAN_POINT ( 'NONE',  ( -30.90169943749473447, 28.08125000068280031, 42.53254041760200721 ) ) ;
#16221=CARTESIAN_POINT ( 'NONE',  ( 50.00000000000000711, 30.89999999999999503, 16.24598481164530739 ) ) ;
#16225=CARTESIAN_POINT ( 'NONE',  ( 15.40903463028482356, 42.45937500034140299, 47.42413220539093999 ) ) ;
#16228=EDGE_LOOP ( 'NONE', ( #10101, #6154, #6867, #4171 ) ) ;
#16230=CARTESIAN_POINT ( 'NONE',  ( 15.40903463028482356, 36.45937500034139589, 47.42413220539093999 ) ) ;
#16234=CARTESIAN_POINT ( 'NONE',  ( 30.90169943749475223, 44.48125000068279888, 42.53254041760199300 ) ) ;
#16241=CARTESIAN_POINT ( 'NONE',  ( -40.34137639590981905, 39.72187500034139873, -29.30972558990011478 ) ) ;
#16245=CARTESIAN_POINT ( 'NONE',  ( -49.86468353124999453, 41.75937500034139305, -16.20201782572375393 ) ) ;
#16247=CARTESIAN_POINT ( 'NONE',  ( -3.219174618344376363E-15, 25.28125000068279604, -52.57311121191334990 ) ) ;
#16252=CARTESIAN_POINT ( 'NONE',  ( -40.34137639590981195, 26.12187500034139731, 29.30972558990012189 ) ) ;
#16257=CARTESIAN_POINT ( 'NONE',  ( 40.34137639590981195, 35.12187500034139731, -29.30972558990011834 ) ) ;
#16258=CARTESIAN_POINT ( 'NONE',  ( -50.00000000000000000, 31.78125000068279959, 0.000000000000000000 ) ) ;
#16261=ORIENTED_EDGE ( 'NONE', *, *, #15446, .F. ) ;
#16265=CARTESIAN_POINT ( 'NONE',  ( -40.45084971874737789, 31.80000000000000071, -29.38926261462365730 ) ) ;
#16269=DIRECTION ( 'NONE',  ( 0.000000000000000000, 0.000000000000000000, 1.000000000000000000 ) ) ;
#16274=CARTESIAN_POINT ( 'NONE',  ( 0.000000000000000000, 25.00000000000000000, 0.000000000000000000 ) ) ;
#16279=CARTESIAN_POINT ( 'NONE',  ( 49.86468353125001585, 24.75937500034140015, 16.20201782572375038 ) ) ;
#16283=CARTESIAN_POINT ( 'NONE',  ( -40.45084971874737079, 37.98125000068279888, 29.38926261462367151 ) ) ;
#16288=ORIENTED_EDGE ( 'NONE', *, *, #3765, .F. ) ;
#16299=CARTESIAN_POINT ( 'NONE',  ( 15.45084971874736723, 29.40000000000000213, -47.55282581475768211 ) ) ;
#16303=AXIS2_PLACEMENT_3D ( 'NONE', #15779, #10960, #8541 ) ;
#16304=CARTESIAN_POINT ( 'NONE',  ( 15.40903463028482356, 46.45937500034139589, 47.42413220539093999 ) ) ;
#16310=CARTESIAN_POINT ( 'NONE',  ( 15.40903463028481113, 37.25937500034140015, -47.42413220539094709 ) ) ;
#16313=CARTESIAN_POINT ( 'NONE',  ( 46.19495089481205241, 24.99999999999999289, -18.77607397657055799 ) ) ;
#16315=CARTESIAN_POINT ( 'NONE',  ( 30.90169943749473802, 47.08125000068280031, -42.53254041760200721 ) ) ;
#16320=CARTESIAN_POINT ( 'NONE',  ( -30.90169943749473447, 30.08125000068279675, 42.53254041760200721 ) ) ;
#16323=CARTESIAN_POINT ( 'NONE',  ( 15.40903463028481113, 37.32187500034140015, -47.42413220539094709 ) ) ;
#16327=CARTESIAN_POINT ( 'NONE',  ( 40.34137639590981905, 40.65937500034139873, 29.30972558990010768 ) ) ;
#16329=CARTESIAN_POINT ( 'NONE',  ( -40.45084971874737079, 25.98125000068279888, 29.38926261462367151 ) ) ;
#16331=CARTESIAN_POINT ( 'NONE',  ( 40.34137639590981905, 22.72187500034139518, 29.30972558990010768 ) ) ;
#16336=CARTESIAN_POINT ( 'NONE',  ( 9.631387414534489405E-15, 20.42187500034139802, 52.43083105670540789 ) ) ;
#16339=DIRECTION ( 'NONE',  ( -0.000000000000000000, -1.000000000000000000, -0.000000000000000000 ) ) ;
#16340=CARTESIAN_POINT ( 'NONE',  ( -49.86468353124999453, 33.82187500034138594, -16.20201782572375393 ) ) ;
#16341=CARTESIAN_POINT ( 'NONE',  ( -40.45084971874737079, 41.98125000068279888, 29.38926261462367151 ) ) ;
#16343=CONICAL_SURFACE ( 'NONE', #9186, 65.00000000000000000, 0.08726646259971666819 ) ;
#16355=DIRECTION ( 'NONE',  ( 0.000000000000000000, 0.000000000000000000, 1.000000000000000000 ) ) ;
#16362=CARTESIAN_POINT ( 'NONE',  ( 40.34137639590981905, 24.65937500034139873, 29.30972558990010768 ) ) ;
#16363=CARTESIAN_POINT ( 'NONE',  ( -15.45084971874737256, 47.38125000068279746, -47.55282581475767500 ) ) ;
#16365=EDGE_LOOP ( 'NONE', ( #2472, #7816, #10532, #3298 ) ) ;
#16367=CARTESIAN_POINT ( 'NONE',  ( -3.219174618344376363E-15, 35.28125000068280315, -52.57311121191334990 ) ) ;
#16373=VECTOR ( 'NONE', #10408, 1000.000000000000000 ) ;
#16384=DIRECTION ( 'NONE',  ( 0.000000000000000000, 1.000000000000000000, 0.000000000000000000 ) ) ;
#16388=CARTESIAN_POINT ( 'NONE',  ( -30.90169943749473802, 24.29999999999999716, 42.53254041760200721 ) ) ;
#16392=CARTESIAN_POINT ( 'NONE',  ( -49.86468353125000164, 45.85937500034140157, 0.000000000000000000 ) ) ;
#16398=CARTESIAN_POINT ( 'NONE',  ( -49.86468353124999453, 27.75937500034139660, -16.20201782572375393 ) ) ;
#16400=DIRECTION ( 'NONE',  ( -0.000000000000000000, -1.000000000000000000, -0.000000000000000000 ) ) ;
#16403=CARTESIAN_POINT ( 'NONE',  ( 45.54143403682535052, 25.00000000000000000, -20.30922080093668924 ) ) ;
#16404=CARTESIAN_POINT ( 'NONE',  ( -2.547328955960238000E-13, 30.28125000068279604, 49.99999999999999289 ) ) ;
#16410=CARTESIAN_POINT ( 'NONE',  ( -40.45084971874737789, 29.58125000068279675, -29.38926261462365730 ) ) ;
#16413=CARTESIAN_POINT ( 'NONE',  ( 40.34137639590981905, 28.72187500034139873, 29.30972558990010768 ) ) ;
#16416=CARTESIAN_POINT ( 'NONE',  ( 40.34137639590981195, 39.05937500034140442, -29.30972558990011834 ) ) ;
#16420=CARTESIAN_POINT ( 'NONE',  ( 50.00000000000000000, 20.78125000068279959, -6.123233995736766085E-15 ) ) ;
#16422=CARTESIAN_POINT ( 'NONE',  ( -30.81806926056962226, 22.22187500034139163, 42.41743335407647919 ) ) ;
#16427=CARTESIAN_POINT ( 'NONE',  ( -30.90169943749474868, 45.70000000000000995, -42.53254041760200721 ) ) ;
#16428=EDGE_CURVE ( 'NONE', #14468, #3644, #10020, .T. ) ;
#16430=CARTESIAN_POINT ( 'NONE',  ( 49.86468353124999453, 49.02187500034140299, -16.20201782572376459 ) ) ;
#16437=CARTESIAN_POINT ( 'NONE',  ( 50.00000000000000000, 45.00000000000000711, -6.123233995736766085E-15 ) ) ;
#16445=CARTESIAN_POINT ( 'NONE',  ( 1.293669679204937499E-13, 39.50000000000000711, -50.00000000000000000 ) ) ;
#16449=CARTESIAN_POINT ( 'NONE',  ( -15.40903463028481646, 27.45937500034139944, -47.42413220539093999 ) ) ;
#16452=EDGE_LOOP ( 'NONE', ( #12807, #15030, #12181, #14611 ) ) ;
#16453=ORIENTED_EDGE ( 'NONE', *, *, #14582, .F. ) ;
#16456=LINE ( 'NONE', #15035, #3051 ) ;
#16461=CARTESIAN_POINT ( 'NONE',  ( 8.446640517145639571E-15, 26.28125000068279959, 50.00000000000000000 ) ) ;
#16464=CARTESIAN_POINT ( 'NONE',  ( 0.000000000000000000, 193.4213562373095385, -50.00000000000000000 ) ) ;
#16465=DIRECTION ( 'NONE',  ( 0.000000000000000000, 0.000000000000000000, 1.000000000000000000 ) ) ;
ENDSEC;
END-ISO-10303-21;
